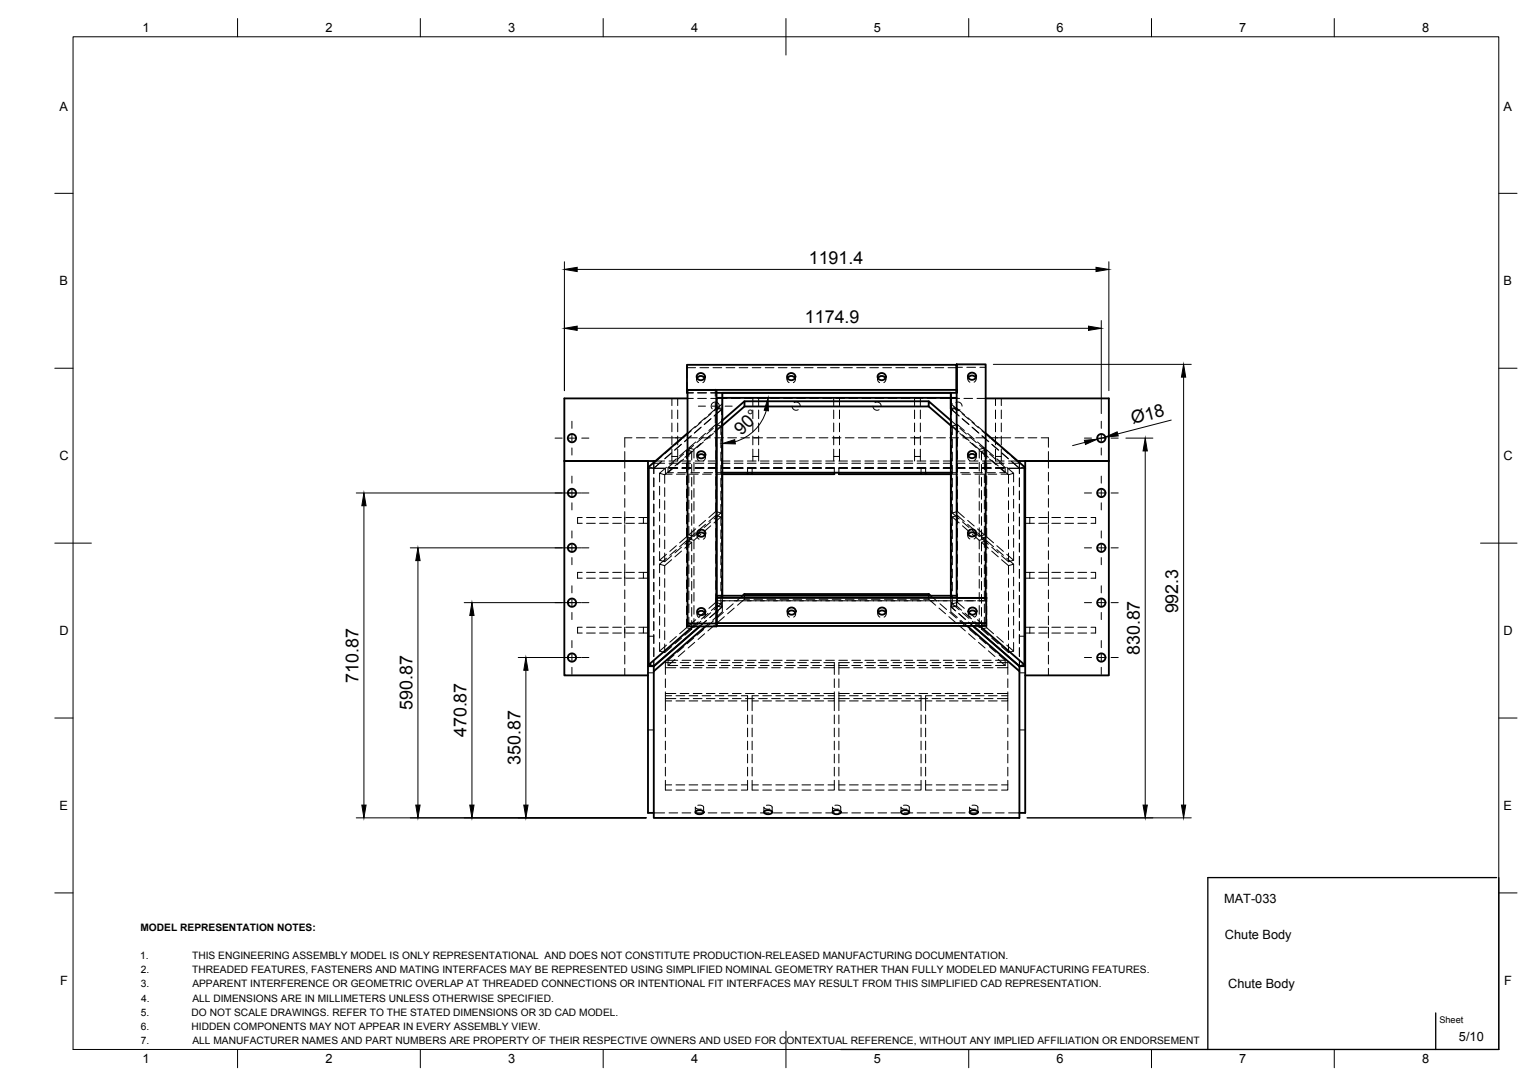
ISO-10303-21;
HEADER;
/* Generated by software containing ST-Developer
 * from STEP Tools, Inc. (www.steptools.com) 
 */

FILE_DESCRIPTION(
/* description */ ('STEP AP214'),
/* implementation_level */ '2;1');

FILE_NAME(
/* name */ 'Chute Body.step',
/* time_stamp */ '2026-11-14T07:13:32-08:00',
/* author */ (''),
/* organization */ (''),
/* preprocessor_version */ 'ST-DEVELOPER v20.2',
/* originating_system */ 'Autodesk Translation Framework v15.17.0.0',
/* authorisation */ '');

FILE_SCHEMA (('AUTOMOTIVE_DESIGN { 1 0 10303 214 3 1 1 }'));
ENDSEC;

DATA;
#10=MECHANICAL_DESIGN_GEOMETRIC_PRESENTATION_REPRESENTATION('',(#1325,#1326,#1327,#1328,#1329,#1330,#1331,#1332,#1333,#1334,#1335,#1336,#1337,#1338,#1339,#1340,#1341,#1342,#1343,#1344,#1345,#1346,#1347,#1348,#1349,#1350,#1351,#1352,#1353,#1354,#1355,#1356,#1357,#1358,#1359,#1360,#1361,#1362,#1363,#1364,#1365,#1366,#1367,#1368,#1369,#1370,#1371,#1372,#1373,#1374,#1375,#1376),#32903);
#682=SHAPE_REPRESENTATION_RELATIONSHIP('SRR','None',#33024,#696);
#696=ADVANCED_BREP_SHAPE_REPRESENTATION('',(#1414,#1415,#1416,#1417,#1418,
#1419,#1420,#1421,#1422,#1423,#1424,#1425,#1426,#1427,#1428,#1429,#1430,
#1431,#1432,#1433,#1434,#1435,#1436,#1437,#1438,#1439,#1440,#1441,#1442,
#1443,#1444,#1445,#1446,#1447,#1448,#1449,#1450,#1451,#1452,#1453,#1454,
#1455,#1456,#1457,#1458,#1459,#1460,#1461,#1462,#1463,#1464,#1465),#32899);
#969=CIRCLE('',#16556,40.);
#970=CIRCLE('',#16557,40.);
#971=CIRCLE('',#16559,75.);
#972=CIRCLE('',#16561,75.);
#973=CIRCLE('',#16569,40.);
#974=CIRCLE('',#16570,40.);
#975=CIRCLE('',#16572,75.);
#976=CIRCLE('',#16574,75.);
#977=CIRCLE('',#16582,8.99999999999999);
#978=CIRCLE('',#16583,8.99999999999999);
#979=CIRCLE('',#16585,8.99999999999999);
#980=CIRCLE('',#16586,8.99999999999999);
#981=CIRCLE('',#16588,8.99999999999998);
#982=CIRCLE('',#16589,8.99999999999998);
#983=CIRCLE('',#16591,9.);
#984=CIRCLE('',#16592,8.99999999999999);
#985=CIRCLE('',#16594,8.99999999999999);
#986=CIRCLE('',#16595,8.99999999999999);
#987=CIRCLE('',#16627,8.99999999999997);
#988=CIRCLE('',#16628,8.99999999999997);
#989=CIRCLE('',#16630,8.99999999999999);
#990=CIRCLE('',#16631,8.99999999999999);
#991=CIRCLE('',#16633,8.99999999999997);
#992=CIRCLE('',#16634,8.99999999999997);
#993=CIRCLE('',#16642,8.99999999999998);
#994=CIRCLE('',#16643,8.99999999999998);
#995=CIRCLE('',#16645,9.);
#996=CIRCLE('',#16646,9.);
#997=CIRCLE('',#16648,8.99999999999995);
#998=CIRCLE('',#16649,8.99999999999995);
#999=CIRCLE('',#16657,8.99999999999998);
#1000=CIRCLE('',#16658,8.99999999999998);
#1001=CIRCLE('',#16660,8.99999999999999);
#1002=CIRCLE('',#16661,8.99999999999999);
#1003=CIRCLE('',#16663,8.99999999999997);
#1004=CIRCLE('',#16664,8.99999999999997);
#1005=CIRCLE('',#16672,8.99999999999998);
#1006=CIRCLE('',#16673,8.99999999999998);
#1007=CIRCLE('',#16675,9.);
#1008=CIRCLE('',#16676,9.);
#1009=CIRCLE('',#16678,8.99999999999995);
#1010=CIRCLE('',#16679,8.99999999999995);
#1011=CIRCLE('',#16717,9.00000000000004);
#1012=CIRCLE('',#16718,9.00000000000004);
#1013=CIRCLE('',#16720,9.00000000000004);
#1014=CIRCLE('',#16721,9.00000000000004);
#1015=CIRCLE('',#16723,9.00000000000006);
#1016=CIRCLE('',#16724,9.00000000000006);
#1017=CIRCLE('',#16726,9.00000000000006);
#1018=CIRCLE('',#16727,9.00000000000006);
#1019=CIRCLE('',#16735,9.00000000000004);
#1020=CIRCLE('',#16736,9.00000000000004);
#1021=CIRCLE('',#16738,9.00000000000004);
#1022=CIRCLE('',#16739,9.00000000000004);
#1023=CIRCLE('',#16741,9.00000000000004);
#1024=CIRCLE('',#16742,9.00000000000004);
#1025=CIRCLE('',#16744,9.00000000000004);
#1026=CIRCLE('',#16745,9.00000000000004);
#1027=CIRCLE('',#16747,9.00000000000004);
#1028=CIRCLE('',#16748,9.00000000000004);
#1029=CIRCLE('',#16750,9.00000000000004);
#1030=CIRCLE('',#16751,9.00000000000004);
#1031=CIRCLE('',#16858,9.00000000000004);
#1032=CIRCLE('',#16859,9.00000000000004);
#1033=CIRCLE('',#16861,9.00000000000004);
#1034=CIRCLE('',#16862,9.00000000000004);
#1035=CIRCLE('',#16864,9.00000000000006);
#1036=CIRCLE('',#16865,9.00000000000006);
#1037=CIRCLE('',#16867,9.00000000000006);
#1038=CIRCLE('',#16868,9.00000000000006);
#1250=CYLINDRICAL_SURFACE('',#16555,40.);
#1251=CYLINDRICAL_SURFACE('',#16566,75.);
#1252=CYLINDRICAL_SURFACE('',#16568,40.);
#1253=CYLINDRICAL_SURFACE('',#16579,75.);
#1254=CYLINDRICAL_SURFACE('',#16581,8.99999999999999);
#1255=CYLINDRICAL_SURFACE('',#16584,8.99999999999999);
#1256=CYLINDRICAL_SURFACE('',#16587,8.99999999999998);
#1257=CYLINDRICAL_SURFACE('',#16590,9.);
#1258=CYLINDRICAL_SURFACE('',#16593,8.99999999999999);
#1259=CYLINDRICAL_SURFACE('',#16626,8.99999999999997);
#1260=CYLINDRICAL_SURFACE('',#16629,8.99999999999999);
#1261=CYLINDRICAL_SURFACE('',#16632,8.99999999999997);
#1262=CYLINDRICAL_SURFACE('',#16641,8.99999999999998);
#1263=CYLINDRICAL_SURFACE('',#16644,9.);
#1264=CYLINDRICAL_SURFACE('',#16647,8.99999999999995);
#1265=CYLINDRICAL_SURFACE('',#16656,8.99999999999998);
#1266=CYLINDRICAL_SURFACE('',#16659,8.99999999999999);
#1267=CYLINDRICAL_SURFACE('',#16662,8.99999999999997);
#1268=CYLINDRICAL_SURFACE('',#16671,8.99999999999998);
#1269=CYLINDRICAL_SURFACE('',#16674,9.);
#1270=CYLINDRICAL_SURFACE('',#16677,8.99999999999996);
#1271=CYLINDRICAL_SURFACE('',#16716,9.00000000000004);
#1272=CYLINDRICAL_SURFACE('',#16719,9.00000000000004);
#1273=CYLINDRICAL_SURFACE('',#16722,9.00000000000006);
#1274=CYLINDRICAL_SURFACE('',#16725,9.00000000000006);
#1275=CYLINDRICAL_SURFACE('',#16734,9.00000000000004);
#1276=CYLINDRICAL_SURFACE('',#16737,9.00000000000004);
#1277=CYLINDRICAL_SURFACE('',#16740,9.00000000000004);
#1278=CYLINDRICAL_SURFACE('',#16743,9.00000000000004);
#1279=CYLINDRICAL_SURFACE('',#16746,9.00000000000004);
#1280=CYLINDRICAL_SURFACE('',#16749,9.00000000000004);
#1281=CYLINDRICAL_SURFACE('',#16857,9.00000000000004);
#1282=CYLINDRICAL_SURFACE('',#16860,9.00000000000004);
#1283=CYLINDRICAL_SURFACE('',#16863,9.00000000000006);
#1284=CYLINDRICAL_SURFACE('',#16866,9.00000000000006);
#1325=STYLED_ITEM('',(#33101),#1414);
#1326=STYLED_ITEM('',(#33101),#1415);
#1327=STYLED_ITEM('',(#33101),#1416);
#1328=STYLED_ITEM('',(#33101),#1417);
#1329=STYLED_ITEM('',(#33101),#1418);
#1330=STYLED_ITEM('',(#33101),#1419);
#1331=STYLED_ITEM('',(#33101),#1420);
#1332=STYLED_ITEM('',(#33101),#1421);
#1333=STYLED_ITEM('',(#33101),#1422);
#1334=STYLED_ITEM('',(#33101),#1423);
#1335=STYLED_ITEM('',(#33101),#1424);
#1336=STYLED_ITEM('',(#33101),#1425);
#1337=STYLED_ITEM('',(#33101),#1426);
#1338=STYLED_ITEM('',(#33101),#1427);
#1339=STYLED_ITEM('',(#33101),#1428);
#1340=STYLED_ITEM('',(#33101),#1429);
#1341=STYLED_ITEM('',(#33101),#1430);
#1342=STYLED_ITEM('',(#33101),#1431);
#1343=STYLED_ITEM('',(#33101),#1432);
#1344=STYLED_ITEM('',(#33101),#1433);
#1345=STYLED_ITEM('',(#33101),#1434);
#1346=STYLED_ITEM('',(#33101),#1435);
#1347=STYLED_ITEM('',(#33101),#1436);
#1348=STYLED_ITEM('',(#33101),#1437);
#1349=STYLED_ITEM('',(#33101),#1438);
#1350=STYLED_ITEM('',(#33101),#1439);
#1351=STYLED_ITEM('',(#33101),#1440);
#1352=STYLED_ITEM('',(#33101),#1441);
#1353=STYLED_ITEM('',(#33101),#1442);
#1354=STYLED_ITEM('',(#33101),#1443);
#1355=STYLED_ITEM('',(#33101),#1444);
#1356=STYLED_ITEM('',(#33101),#1445);
#1357=STYLED_ITEM('',(#33101),#1446);
#1358=STYLED_ITEM('',(#33101),#1447);
#1359=STYLED_ITEM('',(#33101),#1448);
#1360=STYLED_ITEM('',(#33101),#1449);
#1361=STYLED_ITEM('',(#33101),#1450);
#1362=STYLED_ITEM('',(#33101),#1451);
#1363=STYLED_ITEM('',(#33101),#1452);
#1364=STYLED_ITEM('',(#33101),#1453);
#1365=STYLED_ITEM('',(#33101),#1454);
#1366=STYLED_ITEM('',(#33101),#1455);
#1367=STYLED_ITEM('',(#33101),#1456);
#1368=STYLED_ITEM('',(#33101),#1457);
#1369=STYLED_ITEM('',(#33101),#1458);
#1370=STYLED_ITEM('',(#33101),#1459);
#1371=STYLED_ITEM('',(#33101),#1460);
#1372=STYLED_ITEM('',(#33101),#1461);
#1373=STYLED_ITEM('',(#33101),#1462);
#1374=STYLED_ITEM('',(#33101),#1463);
#1375=STYLED_ITEM('',(#33101),#1464);
#1376=STYLED_ITEM('',(#33101),#1465);
#1414=MANIFOLD_SOLID_BREP('Body1',#15573);
#1415=MANIFOLD_SOLID_BREP('Body2',#15574);
#1416=MANIFOLD_SOLID_BREP('Body3',#15575);
#1417=MANIFOLD_SOLID_BREP('Body4',#15576);
#1418=MANIFOLD_SOLID_BREP('Body5',#15577);
#1419=MANIFOLD_SOLID_BREP('Body6',#15578);
#1420=MANIFOLD_SOLID_BREP('Body7',#15579);
#1421=MANIFOLD_SOLID_BREP('Body8',#15580);
#1422=MANIFOLD_SOLID_BREP('Body9',#15581);
#1423=MANIFOLD_SOLID_BREP('Body10',#15582);
#1424=MANIFOLD_SOLID_BREP('Body11',#15583);
#1425=MANIFOLD_SOLID_BREP('Body12',#15584);
#1426=MANIFOLD_SOLID_BREP('Body13',#15585);
#1427=MANIFOLD_SOLID_BREP('Body14',#15586);
#1428=MANIFOLD_SOLID_BREP('Body15',#15587);
#1429=MANIFOLD_SOLID_BREP('Body16',#15588);
#1430=MANIFOLD_SOLID_BREP('Body17',#15589);
#1431=MANIFOLD_SOLID_BREP('Body18',#15590);
#1432=MANIFOLD_SOLID_BREP('Body19',#15591);
#1433=MANIFOLD_SOLID_BREP('Body20',#15592);
#1434=MANIFOLD_SOLID_BREP('Body21',#15593);
#1435=MANIFOLD_SOLID_BREP('Body22',#15594);
#1436=MANIFOLD_SOLID_BREP('Body23',#15595);
#1437=MANIFOLD_SOLID_BREP('Body24',#15596);
#1438=MANIFOLD_SOLID_BREP('Body25',#15597);
#1439=MANIFOLD_SOLID_BREP('Body26',#15598);
#1440=MANIFOLD_SOLID_BREP('Body27',#15599);
#1441=MANIFOLD_SOLID_BREP('Body28',#15600);
#1442=MANIFOLD_SOLID_BREP('Body29',#15601);
#1443=MANIFOLD_SOLID_BREP('Body30',#15602);
#1444=MANIFOLD_SOLID_BREP('Body31',#15603);
#1445=MANIFOLD_SOLID_BREP('Body32',#15604);
#1446=MANIFOLD_SOLID_BREP('Body33',#15605);
#1447=MANIFOLD_SOLID_BREP('Body34',#15606);
#1448=MANIFOLD_SOLID_BREP('Body35',#15607);
#1449=MANIFOLD_SOLID_BREP('Body36',#15608);
#1450=MANIFOLD_SOLID_BREP('Body37',#15609);
#1451=MANIFOLD_SOLID_BREP('Body38',#15610);
#1452=MANIFOLD_SOLID_BREP('Body39',#15611);
#1453=MANIFOLD_SOLID_BREP('Body40',#15612);
#1454=MANIFOLD_SOLID_BREP('Body41',#15613);
#1455=MANIFOLD_SOLID_BREP('Body42',#15614);
#1456=MANIFOLD_SOLID_BREP('Body43',#15615);
#1457=MANIFOLD_SOLID_BREP('Body44',#15616);
#1458=MANIFOLD_SOLID_BREP('Body45',#15617);
#1459=MANIFOLD_SOLID_BREP('Body46',#15618);
#1460=MANIFOLD_SOLID_BREP('Body47',#15619);
#1461=MANIFOLD_SOLID_BREP('Body48',#15620);
#1462=MANIFOLD_SOLID_BREP('Body49',#15621);
#1463=MANIFOLD_SOLID_BREP('Body50',#15622);
#1464=MANIFOLD_SOLID_BREP('Body51',#15623);
#1465=MANIFOLD_SOLID_BREP('Body52',#15624);
#1605=FACE_BOUND('',#3169,.T.);
#1606=FACE_BOUND('',#3171,.T.);
#1607=FACE_BOUND('',#3180,.T.);
#1608=FACE_BOUND('',#3182,.T.);
#1609=FACE_BOUND('',#3195,.T.);
#1610=FACE_BOUND('',#3196,.T.);
#1611=FACE_BOUND('',#3197,.T.);
#1612=FACE_BOUND('',#3198,.T.);
#1613=FACE_BOUND('',#3199,.T.);
#1614=FACE_BOUND('',#3201,.T.);
#1615=FACE_BOUND('',#3202,.T.);
#1616=FACE_BOUND('',#3203,.T.);
#1617=FACE_BOUND('',#3204,.T.);
#1618=FACE_BOUND('',#3205,.T.);
#1619=FACE_BOUND('',#3238,.T.);
#1620=FACE_BOUND('',#3239,.T.);
#1621=FACE_BOUND('',#3240,.T.);
#1622=FACE_BOUND('',#3242,.T.);
#1623=FACE_BOUND('',#3243,.T.);
#1624=FACE_BOUND('',#3244,.T.);
#1625=FACE_BOUND('',#3253,.T.);
#1626=FACE_BOUND('',#3254,.T.);
#1627=FACE_BOUND('',#3255,.T.);
#1628=FACE_BOUND('',#3257,.T.);
#1629=FACE_BOUND('',#3258,.T.);
#1630=FACE_BOUND('',#3259,.T.);
#1631=FACE_BOUND('',#3268,.T.);
#1632=FACE_BOUND('',#3269,.T.);
#1633=FACE_BOUND('',#3270,.T.);
#1634=FACE_BOUND('',#3272,.T.);
#1635=FACE_BOUND('',#3273,.T.);
#1636=FACE_BOUND('',#3274,.T.);
#1637=FACE_BOUND('',#3283,.T.);
#1638=FACE_BOUND('',#3284,.T.);
#1639=FACE_BOUND('',#3285,.T.);
#1640=FACE_BOUND('',#3287,.T.);
#1641=FACE_BOUND('',#3288,.T.);
#1642=FACE_BOUND('',#3289,.T.);
#1643=FACE_BOUND('',#3329,.T.);
#1644=FACE_BOUND('',#3330,.T.);
#1645=FACE_BOUND('',#3331,.T.);
#1646=FACE_BOUND('',#3332,.T.);
#1647=FACE_BOUND('',#3334,.T.);
#1648=FACE_BOUND('',#3335,.T.);
#1649=FACE_BOUND('',#3336,.T.);
#1650=FACE_BOUND('',#3337,.T.);
#1651=FACE_BOUND('',#3353,.T.);
#1652=FACE_BOUND('',#3354,.T.);
#1653=FACE_BOUND('',#3355,.T.);
#1654=FACE_BOUND('',#3356,.T.);
#1655=FACE_BOUND('',#3357,.T.);
#1656=FACE_BOUND('',#3358,.T.);
#1657=FACE_BOUND('',#3360,.T.);
#1658=FACE_BOUND('',#3361,.T.);
#1659=FACE_BOUND('',#3362,.T.);
#1660=FACE_BOUND('',#3363,.T.);
#1661=FACE_BOUND('',#3364,.T.);
#1662=FACE_BOUND('',#3365,.T.);
#1663=FACE_BOUND('',#3470,.T.);
#1664=FACE_BOUND('',#3471,.T.);
#1665=FACE_BOUND('',#3472,.T.);
#1666=FACE_BOUND('',#3473,.T.);
#1667=FACE_BOUND('',#3475,.T.);
#1668=FACE_BOUND('',#3476,.T.);
#1669=FACE_BOUND('',#3477,.T.);
#1670=FACE_BOUND('',#3478,.T.);
#2130=FACE_OUTER_BOUND('',#3161,.T.);
#2131=FACE_OUTER_BOUND('',#3162,.T.);
#2132=FACE_OUTER_BOUND('',#3163,.T.);
#2133=FACE_OUTER_BOUND('',#3164,.T.);
#2134=FACE_OUTER_BOUND('',#3165,.T.);
#2135=FACE_OUTER_BOUND('',#3166,.T.);
#2136=FACE_OUTER_BOUND('',#3167,.T.);
#2137=FACE_OUTER_BOUND('',#3168,.T.);
#2138=FACE_OUTER_BOUND('',#3170,.T.);
#2139=FACE_OUTER_BOUND('',#3172,.T.);
#2140=FACE_OUTER_BOUND('',#3173,.T.);
#2141=FACE_OUTER_BOUND('',#3174,.T.);
#2142=FACE_OUTER_BOUND('',#3175,.T.);
#2143=FACE_OUTER_BOUND('',#3176,.T.);
#2144=FACE_OUTER_BOUND('',#3177,.T.);
#2145=FACE_OUTER_BOUND('',#3178,.T.);
#2146=FACE_OUTER_BOUND('',#3179,.T.);
#2147=FACE_OUTER_BOUND('',#3181,.T.);
#2148=FACE_OUTER_BOUND('',#3183,.T.);
#2149=FACE_OUTER_BOUND('',#3184,.T.);
#2150=FACE_OUTER_BOUND('',#3185,.T.);
#2151=FACE_OUTER_BOUND('',#3186,.T.);
#2152=FACE_OUTER_BOUND('',#3187,.T.);
#2153=FACE_OUTER_BOUND('',#3188,.T.);
#2154=FACE_OUTER_BOUND('',#3189,.T.);
#2155=FACE_OUTER_BOUND('',#3190,.T.);
#2156=FACE_OUTER_BOUND('',#3191,.T.);
#2157=FACE_OUTER_BOUND('',#3192,.T.);
#2158=FACE_OUTER_BOUND('',#3193,.T.);
#2159=FACE_OUTER_BOUND('',#3194,.T.);
#2160=FACE_OUTER_BOUND('',#3200,.T.);
#2161=FACE_OUTER_BOUND('',#3206,.T.);
#2162=FACE_OUTER_BOUND('',#3207,.T.);
#2163=FACE_OUTER_BOUND('',#3208,.T.);
#2164=FACE_OUTER_BOUND('',#3209,.T.);
#2165=FACE_OUTER_BOUND('',#3210,.T.);
#2166=FACE_OUTER_BOUND('',#3211,.T.);
#2167=FACE_OUTER_BOUND('',#3212,.T.);
#2168=FACE_OUTER_BOUND('',#3213,.T.);
#2169=FACE_OUTER_BOUND('',#3214,.T.);
#2170=FACE_OUTER_BOUND('',#3215,.T.);
#2171=FACE_OUTER_BOUND('',#3216,.T.);
#2172=FACE_OUTER_BOUND('',#3217,.T.);
#2173=FACE_OUTER_BOUND('',#3218,.T.);
#2174=FACE_OUTER_BOUND('',#3219,.T.);
#2175=FACE_OUTER_BOUND('',#3220,.T.);
#2176=FACE_OUTER_BOUND('',#3221,.T.);
#2177=FACE_OUTER_BOUND('',#3222,.T.);
#2178=FACE_OUTER_BOUND('',#3223,.T.);
#2179=FACE_OUTER_BOUND('',#3224,.T.);
#2180=FACE_OUTER_BOUND('',#3225,.T.);
#2181=FACE_OUTER_BOUND('',#3226,.T.);
#2182=FACE_OUTER_BOUND('',#3227,.T.);
#2183=FACE_OUTER_BOUND('',#3228,.T.);
#2184=FACE_OUTER_BOUND('',#3229,.T.);
#2185=FACE_OUTER_BOUND('',#3230,.T.);
#2186=FACE_OUTER_BOUND('',#3231,.T.);
#2187=FACE_OUTER_BOUND('',#3232,.T.);
#2188=FACE_OUTER_BOUND('',#3233,.T.);
#2189=FACE_OUTER_BOUND('',#3234,.T.);
#2190=FACE_OUTER_BOUND('',#3235,.T.);
#2191=FACE_OUTER_BOUND('',#3236,.T.);
#2192=FACE_OUTER_BOUND('',#3237,.T.);
#2193=FACE_OUTER_BOUND('',#3241,.T.);
#2194=FACE_OUTER_BOUND('',#3245,.T.);
#2195=FACE_OUTER_BOUND('',#3246,.T.);
#2196=FACE_OUTER_BOUND('',#3247,.T.);
#2197=FACE_OUTER_BOUND('',#3248,.T.);
#2198=FACE_OUTER_BOUND('',#3249,.T.);
#2199=FACE_OUTER_BOUND('',#3250,.T.);
#2200=FACE_OUTER_BOUND('',#3251,.T.);
#2201=FACE_OUTER_BOUND('',#3252,.T.);
#2202=FACE_OUTER_BOUND('',#3256,.T.);
#2203=FACE_OUTER_BOUND('',#3260,.T.);
#2204=FACE_OUTER_BOUND('',#3261,.T.);
#2205=FACE_OUTER_BOUND('',#3262,.T.);
#2206=FACE_OUTER_BOUND('',#3263,.T.);
#2207=FACE_OUTER_BOUND('',#3264,.T.);
#2208=FACE_OUTER_BOUND('',#3265,.T.);
#2209=FACE_OUTER_BOUND('',#3266,.T.);
#2210=FACE_OUTER_BOUND('',#3267,.T.);
#2211=FACE_OUTER_BOUND('',#3271,.T.);
#2212=FACE_OUTER_BOUND('',#3275,.T.);
#2213=FACE_OUTER_BOUND('',#3276,.T.);
#2214=FACE_OUTER_BOUND('',#3277,.T.);
#2215=FACE_OUTER_BOUND('',#3278,.T.);
#2216=FACE_OUTER_BOUND('',#3279,.T.);
#2217=FACE_OUTER_BOUND('',#3280,.T.);
#2218=FACE_OUTER_BOUND('',#3281,.T.);
#2219=FACE_OUTER_BOUND('',#3282,.T.);
#2220=FACE_OUTER_BOUND('',#3286,.T.);
#2221=FACE_OUTER_BOUND('',#3290,.T.);
#2222=FACE_OUTER_BOUND('',#3291,.T.);
#2223=FACE_OUTER_BOUND('',#3292,.T.);
#2224=FACE_OUTER_BOUND('',#3293,.T.);
#2225=FACE_OUTER_BOUND('',#3294,.T.);
#2226=FACE_OUTER_BOUND('',#3295,.T.);
#2227=FACE_OUTER_BOUND('',#3296,.T.);
#2228=FACE_OUTER_BOUND('',#3297,.T.);
#2229=FACE_OUTER_BOUND('',#3298,.T.);
#2230=FACE_OUTER_BOUND('',#3299,.T.);
#2231=FACE_OUTER_BOUND('',#3300,.T.);
#2232=FACE_OUTER_BOUND('',#3301,.T.);
#2233=FACE_OUTER_BOUND('',#3302,.T.);
#2234=FACE_OUTER_BOUND('',#3303,.T.);
#2235=FACE_OUTER_BOUND('',#3304,.T.);
#2236=FACE_OUTER_BOUND('',#3305,.T.);
#2237=FACE_OUTER_BOUND('',#3306,.T.);
#2238=FACE_OUTER_BOUND('',#3307,.T.);
#2239=FACE_OUTER_BOUND('',#3308,.T.);
#2240=FACE_OUTER_BOUND('',#3309,.T.);
#2241=FACE_OUTER_BOUND('',#3310,.T.);
#2242=FACE_OUTER_BOUND('',#3311,.T.);
#2243=FACE_OUTER_BOUND('',#3312,.T.);
#2244=FACE_OUTER_BOUND('',#3313,.T.);
#2245=FACE_OUTER_BOUND('',#3314,.T.);
#2246=FACE_OUTER_BOUND('',#3315,.T.);
#2247=FACE_OUTER_BOUND('',#3316,.T.);
#2248=FACE_OUTER_BOUND('',#3317,.T.);
#2249=FACE_OUTER_BOUND('',#3318,.T.);
#2250=FACE_OUTER_BOUND('',#3319,.T.);
#2251=FACE_OUTER_BOUND('',#3320,.T.);
#2252=FACE_OUTER_BOUND('',#3321,.T.);
#2253=FACE_OUTER_BOUND('',#3322,.T.);
#2254=FACE_OUTER_BOUND('',#3323,.T.);
#2255=FACE_OUTER_BOUND('',#3324,.T.);
#2256=FACE_OUTER_BOUND('',#3325,.T.);
#2257=FACE_OUTER_BOUND('',#3326,.T.);
#2258=FACE_OUTER_BOUND('',#3327,.T.);
#2259=FACE_OUTER_BOUND('',#3328,.T.);
#2260=FACE_OUTER_BOUND('',#3333,.T.);
#2261=FACE_OUTER_BOUND('',#3338,.T.);
#2262=FACE_OUTER_BOUND('',#3339,.T.);
#2263=FACE_OUTER_BOUND('',#3340,.T.);
#2264=FACE_OUTER_BOUND('',#3341,.T.);
#2265=FACE_OUTER_BOUND('',#3342,.T.);
#2266=FACE_OUTER_BOUND('',#3343,.T.);
#2267=FACE_OUTER_BOUND('',#3344,.T.);
#2268=FACE_OUTER_BOUND('',#3345,.T.);
#2269=FACE_OUTER_BOUND('',#3346,.T.);
#2270=FACE_OUTER_BOUND('',#3347,.T.);
#2271=FACE_OUTER_BOUND('',#3348,.T.);
#2272=FACE_OUTER_BOUND('',#3349,.T.);
#2273=FACE_OUTER_BOUND('',#3350,.T.);
#2274=FACE_OUTER_BOUND('',#3351,.T.);
#2275=FACE_OUTER_BOUND('',#3352,.T.);
#2276=FACE_OUTER_BOUND('',#3359,.T.);
#2277=FACE_OUTER_BOUND('',#3366,.T.);
#2278=FACE_OUTER_BOUND('',#3367,.T.);
#2279=FACE_OUTER_BOUND('',#3368,.T.);
#2280=FACE_OUTER_BOUND('',#3369,.T.);
#2281=FACE_OUTER_BOUND('',#3370,.T.);
#2282=FACE_OUTER_BOUND('',#3371,.T.);
#2283=FACE_OUTER_BOUND('',#3372,.T.);
#2284=FACE_OUTER_BOUND('',#3373,.T.);
#2285=FACE_OUTER_BOUND('',#3374,.T.);
#2286=FACE_OUTER_BOUND('',#3375,.T.);
#2287=FACE_OUTER_BOUND('',#3376,.T.);
#2288=FACE_OUTER_BOUND('',#3377,.T.);
#2289=FACE_OUTER_BOUND('',#3378,.T.);
#2290=FACE_OUTER_BOUND('',#3379,.T.);
#2291=FACE_OUTER_BOUND('',#3380,.T.);
#2292=FACE_OUTER_BOUND('',#3381,.T.);
#2293=FACE_OUTER_BOUND('',#3382,.T.);
#2294=FACE_OUTER_BOUND('',#3383,.T.);
#2295=FACE_OUTER_BOUND('',#3384,.T.);
#2296=FACE_OUTER_BOUND('',#3385,.T.);
#2297=FACE_OUTER_BOUND('',#3386,.T.);
#2298=FACE_OUTER_BOUND('',#3387,.T.);
#2299=FACE_OUTER_BOUND('',#3388,.T.);
#2300=FACE_OUTER_BOUND('',#3389,.T.);
#2301=FACE_OUTER_BOUND('',#3390,.T.);
#2302=FACE_OUTER_BOUND('',#3391,.T.);
#2303=FACE_OUTER_BOUND('',#3392,.T.);
#2304=FACE_OUTER_BOUND('',#3393,.T.);
#2305=FACE_OUTER_BOUND('',#3394,.T.);
#2306=FACE_OUTER_BOUND('',#3395,.T.);
#2307=FACE_OUTER_BOUND('',#3396,.T.);
#2308=FACE_OUTER_BOUND('',#3397,.T.);
#2309=FACE_OUTER_BOUND('',#3398,.T.);
#2310=FACE_OUTER_BOUND('',#3399,.T.);
#2311=FACE_OUTER_BOUND('',#3400,.T.);
#2312=FACE_OUTER_BOUND('',#3401,.T.);
#2313=FACE_OUTER_BOUND('',#3402,.T.);
#2314=FACE_OUTER_BOUND('',#3403,.T.);
#2315=FACE_OUTER_BOUND('',#3404,.T.);
#2316=FACE_OUTER_BOUND('',#3405,.T.);
#2317=FACE_OUTER_BOUND('',#3406,.T.);
#2318=FACE_OUTER_BOUND('',#3407,.T.);
#2319=FACE_OUTER_BOUND('',#3408,.T.);
#2320=FACE_OUTER_BOUND('',#3409,.T.);
#2321=FACE_OUTER_BOUND('',#3410,.T.);
#2322=FACE_OUTER_BOUND('',#3411,.T.);
#2323=FACE_OUTER_BOUND('',#3412,.T.);
#2324=FACE_OUTER_BOUND('',#3413,.T.);
#2325=FACE_OUTER_BOUND('',#3414,.T.);
#2326=FACE_OUTER_BOUND('',#3415,.T.);
#2327=FACE_OUTER_BOUND('',#3416,.T.);
#2328=FACE_OUTER_BOUND('',#3417,.T.);
#2329=FACE_OUTER_BOUND('',#3418,.T.);
#2330=FACE_OUTER_BOUND('',#3419,.T.);
#2331=FACE_OUTER_BOUND('',#3420,.T.);
#2332=FACE_OUTER_BOUND('',#3421,.T.);
#2333=FACE_OUTER_BOUND('',#3422,.T.);
#2334=FACE_OUTER_BOUND('',#3423,.T.);
#2335=FACE_OUTER_BOUND('',#3424,.T.);
#2336=FACE_OUTER_BOUND('',#3425,.T.);
#2337=FACE_OUTER_BOUND('',#3426,.T.);
#2338=FACE_OUTER_BOUND('',#3427,.T.);
#2339=FACE_OUTER_BOUND('',#3428,.T.);
#2340=FACE_OUTER_BOUND('',#3429,.T.);
#2341=FACE_OUTER_BOUND('',#3430,.T.);
#2342=FACE_OUTER_BOUND('',#3431,.T.);
#2343=FACE_OUTER_BOUND('',#3432,.T.);
#2344=FACE_OUTER_BOUND('',#3433,.T.);
#2345=FACE_OUTER_BOUND('',#3434,.T.);
#2346=FACE_OUTER_BOUND('',#3435,.T.);
#2347=FACE_OUTER_BOUND('',#3436,.T.);
#2348=FACE_OUTER_BOUND('',#3437,.T.);
#2349=FACE_OUTER_BOUND('',#3438,.T.);
#2350=FACE_OUTER_BOUND('',#3439,.T.);
#2351=FACE_OUTER_BOUND('',#3440,.T.);
#2352=FACE_OUTER_BOUND('',#3441,.T.);
#2353=FACE_OUTER_BOUND('',#3442,.T.);
#2354=FACE_OUTER_BOUND('',#3443,.T.);
#2355=FACE_OUTER_BOUND('',#3444,.T.);
#2356=FACE_OUTER_BOUND('',#3445,.T.);
#2357=FACE_OUTER_BOUND('',#3446,.T.);
#2358=FACE_OUTER_BOUND('',#3447,.T.);
#2359=FACE_OUTER_BOUND('',#3448,.T.);
#2360=FACE_OUTER_BOUND('',#3449,.T.);
#2361=FACE_OUTER_BOUND('',#3450,.T.);
#2362=FACE_OUTER_BOUND('',#3451,.T.);
#2363=FACE_OUTER_BOUND('',#3452,.T.);
#2364=FACE_OUTER_BOUND('',#3453,.T.);
#2365=FACE_OUTER_BOUND('',#3454,.T.);
#2366=FACE_OUTER_BOUND('',#3455,.T.);
#2367=FACE_OUTER_BOUND('',#3456,.T.);
#2368=FACE_OUTER_BOUND('',#3457,.T.);
#2369=FACE_OUTER_BOUND('',#3458,.T.);
#2370=FACE_OUTER_BOUND('',#3459,.T.);
#2371=FACE_OUTER_BOUND('',#3460,.T.);
#2372=FACE_OUTER_BOUND('',#3461,.T.);
#2373=FACE_OUTER_BOUND('',#3462,.T.);
#2374=FACE_OUTER_BOUND('',#3463,.T.);
#2375=FACE_OUTER_BOUND('',#3464,.T.);
#2376=FACE_OUTER_BOUND('',#3465,.T.);
#2377=FACE_OUTER_BOUND('',#3466,.T.);
#2378=FACE_OUTER_BOUND('',#3467,.T.);
#2379=FACE_OUTER_BOUND('',#3468,.T.);
#2380=FACE_OUTER_BOUND('',#3469,.T.);
#2381=FACE_OUTER_BOUND('',#3474,.T.);
#2382=FACE_OUTER_BOUND('',#3479,.T.);
#2383=FACE_OUTER_BOUND('',#3480,.T.);
#2384=FACE_OUTER_BOUND('',#3481,.T.);
#2385=FACE_OUTER_BOUND('',#3482,.T.);
#2386=FACE_OUTER_BOUND('',#3483,.T.);
#2387=FACE_OUTER_BOUND('',#3484,.T.);
#2388=FACE_OUTER_BOUND('',#3485,.T.);
#2389=FACE_OUTER_BOUND('',#3486,.T.);
#2390=FACE_OUTER_BOUND('',#3487,.T.);
#2391=FACE_OUTER_BOUND('',#3488,.T.);
#2392=FACE_OUTER_BOUND('',#3489,.T.);
#2393=FACE_OUTER_BOUND('',#3490,.T.);
#2394=FACE_OUTER_BOUND('',#3491,.T.);
#2395=FACE_OUTER_BOUND('',#3492,.T.);
#2396=FACE_OUTER_BOUND('',#3493,.T.);
#2397=FACE_OUTER_BOUND('',#3494,.T.);
#2398=FACE_OUTER_BOUND('',#3495,.T.);
#2399=FACE_OUTER_BOUND('',#3496,.T.);
#2400=FACE_OUTER_BOUND('',#3497,.T.);
#2401=FACE_OUTER_BOUND('',#3498,.T.);
#2402=FACE_OUTER_BOUND('',#3499,.T.);
#2403=FACE_OUTER_BOUND('',#3500,.T.);
#2404=FACE_OUTER_BOUND('',#3501,.T.);
#2405=FACE_OUTER_BOUND('',#3502,.T.);
#2406=FACE_OUTER_BOUND('',#3503,.T.);
#2407=FACE_OUTER_BOUND('',#3504,.T.);
#2408=FACE_OUTER_BOUND('',#3505,.T.);
#2409=FACE_OUTER_BOUND('',#3506,.T.);
#2410=FACE_OUTER_BOUND('',#3507,.T.);
#2411=FACE_OUTER_BOUND('',#3508,.T.);
#2412=FACE_OUTER_BOUND('',#3509,.T.);
#2413=FACE_OUTER_BOUND('',#3510,.T.);
#2414=FACE_OUTER_BOUND('',#3511,.T.);
#2415=FACE_OUTER_BOUND('',#3512,.T.);
#2416=FACE_OUTER_BOUND('',#3513,.T.);
#2417=FACE_OUTER_BOUND('',#3514,.T.);
#2418=FACE_OUTER_BOUND('',#3515,.T.);
#2419=FACE_OUTER_BOUND('',#3516,.T.);
#2420=FACE_OUTER_BOUND('',#3517,.T.);
#2421=FACE_OUTER_BOUND('',#3518,.T.);
#2422=FACE_OUTER_BOUND('',#3519,.T.);
#2423=FACE_OUTER_BOUND('',#3520,.T.);
#2424=FACE_OUTER_BOUND('',#3521,.T.);
#2425=FACE_OUTER_BOUND('',#3522,.T.);
#2426=FACE_OUTER_BOUND('',#3523,.T.);
#2427=FACE_OUTER_BOUND('',#3524,.T.);
#2428=FACE_OUTER_BOUND('',#3525,.T.);
#2429=FACE_OUTER_BOUND('',#3526,.T.);
#2430=FACE_OUTER_BOUND('',#3527,.T.);
#2431=FACE_OUTER_BOUND('',#3528,.T.);
#2432=FACE_OUTER_BOUND('',#3529,.T.);
#2433=FACE_OUTER_BOUND('',#3530,.T.);
#2434=FACE_OUTER_BOUND('',#3531,.T.);
#2435=FACE_OUTER_BOUND('',#3532,.T.);
#2436=FACE_OUTER_BOUND('',#3533,.T.);
#2437=FACE_OUTER_BOUND('',#3534,.T.);
#2438=FACE_OUTER_BOUND('',#3535,.T.);
#2439=FACE_OUTER_BOUND('',#3536,.T.);
#2440=FACE_OUTER_BOUND('',#3537,.T.);
#2441=FACE_OUTER_BOUND('',#3538,.T.);
#2442=FACE_OUTER_BOUND('',#3539,.T.);
#2443=FACE_OUTER_BOUND('',#3540,.T.);
#2444=FACE_OUTER_BOUND('',#3541,.T.);
#2445=FACE_OUTER_BOUND('',#3542,.T.);
#2446=FACE_OUTER_BOUND('',#3543,.T.);
#2447=FACE_OUTER_BOUND('',#3544,.T.);
#2448=FACE_OUTER_BOUND('',#3545,.T.);
#2449=FACE_OUTER_BOUND('',#3546,.T.);
#2450=FACE_OUTER_BOUND('',#3547,.T.);
#2451=FACE_OUTER_BOUND('',#3548,.T.);
#2452=FACE_OUTER_BOUND('',#3549,.T.);
#2453=FACE_OUTER_BOUND('',#3550,.T.);
#2454=FACE_OUTER_BOUND('',#3551,.T.);
#2455=FACE_OUTER_BOUND('',#3552,.T.);
#2456=FACE_OUTER_BOUND('',#3553,.T.);
#2457=FACE_OUTER_BOUND('',#3554,.T.);
#2458=FACE_OUTER_BOUND('',#3555,.T.);
#2459=FACE_OUTER_BOUND('',#3556,.T.);
#2460=FACE_OUTER_BOUND('',#3557,.T.);
#2461=FACE_OUTER_BOUND('',#3558,.T.);
#2462=FACE_OUTER_BOUND('',#3559,.T.);
#2463=FACE_OUTER_BOUND('',#3560,.T.);
#2464=FACE_OUTER_BOUND('',#3561,.T.);
#2465=FACE_OUTER_BOUND('',#3562,.T.);
#2466=FACE_OUTER_BOUND('',#3563,.T.);
#2467=FACE_OUTER_BOUND('',#3564,.T.);
#2468=FACE_OUTER_BOUND('',#3565,.T.);
#2469=FACE_OUTER_BOUND('',#3566,.T.);
#2470=FACE_OUTER_BOUND('',#3567,.T.);
#2471=FACE_OUTER_BOUND('',#3568,.T.);
#2472=FACE_OUTER_BOUND('',#3569,.T.);
#2473=FACE_OUTER_BOUND('',#3570,.T.);
#2474=FACE_OUTER_BOUND('',#3571,.T.);
#2475=FACE_OUTER_BOUND('',#3572,.T.);
#2476=FACE_OUTER_BOUND('',#3573,.T.);
#2477=FACE_OUTER_BOUND('',#3574,.T.);
#2478=FACE_OUTER_BOUND('',#3575,.T.);
#2479=FACE_OUTER_BOUND('',#3576,.T.);
#2480=FACE_OUTER_BOUND('',#3577,.T.);
#2481=FACE_OUTER_BOUND('',#3578,.T.);
#2482=FACE_OUTER_BOUND('',#3579,.T.);
#2483=FACE_OUTER_BOUND('',#3580,.T.);
#2484=FACE_OUTER_BOUND('',#3581,.T.);
#2485=FACE_OUTER_BOUND('',#3582,.T.);
#2486=FACE_OUTER_BOUND('',#3583,.T.);
#2487=FACE_OUTER_BOUND('',#3584,.T.);
#2488=FACE_OUTER_BOUND('',#3585,.T.);
#2489=FACE_OUTER_BOUND('',#3586,.T.);
#2490=FACE_OUTER_BOUND('',#3587,.T.);
#2491=FACE_OUTER_BOUND('',#3588,.T.);
#2492=FACE_OUTER_BOUND('',#3589,.T.);
#2493=FACE_OUTER_BOUND('',#3590,.T.);
#2494=FACE_OUTER_BOUND('',#3591,.T.);
#2495=FACE_OUTER_BOUND('',#3592,.T.);
#2496=FACE_OUTER_BOUND('',#3593,.T.);
#2497=FACE_OUTER_BOUND('',#3594,.T.);
#2498=FACE_OUTER_BOUND('',#3595,.T.);
#2499=FACE_OUTER_BOUND('',#3596,.T.);
#2500=FACE_OUTER_BOUND('',#3597,.T.);
#2501=FACE_OUTER_BOUND('',#3598,.T.);
#2502=FACE_OUTER_BOUND('',#3599,.T.);
#2503=FACE_OUTER_BOUND('',#3600,.T.);
#2504=FACE_OUTER_BOUND('',#3601,.T.);
#2505=FACE_OUTER_BOUND('',#3602,.T.);
#2506=FACE_OUTER_BOUND('',#3603,.T.);
#2507=FACE_OUTER_BOUND('',#3604,.T.);
#2508=FACE_OUTER_BOUND('',#3605,.T.);
#2509=FACE_OUTER_BOUND('',#3606,.T.);
#2510=FACE_OUTER_BOUND('',#3607,.T.);
#2511=FACE_OUTER_BOUND('',#3608,.T.);
#2512=FACE_OUTER_BOUND('',#3609,.T.);
#2513=FACE_OUTER_BOUND('',#3610,.T.);
#2514=FACE_OUTER_BOUND('',#3611,.T.);
#2515=FACE_OUTER_BOUND('',#3612,.T.);
#2516=FACE_OUTER_BOUND('',#3613,.T.);
#2517=FACE_OUTER_BOUND('',#3614,.T.);
#3161=EDGE_LOOP('',(#12121,#12122,#12123,#12124));
#3162=EDGE_LOOP('',(#12125,#12126,#12127,#12128));
#3163=EDGE_LOOP('',(#12129,#12130,#12131,#12132));
#3164=EDGE_LOOP('',(#12133,#12134,#12135,#12136));
#3165=EDGE_LOOP('',(#12137,#12138,#12139,#12140));
#3166=EDGE_LOOP('',(#12141,#12142,#12143,#12144));
#3167=EDGE_LOOP('',(#12145,#12146,#12147,#12148));
#3168=EDGE_LOOP('',(#12149,#12150,#12151,#12152,#12153,#12154));
#3169=EDGE_LOOP('',(#12155));
#3170=EDGE_LOOP('',(#12156,#12157,#12158,#12159,#12160,#12161));
#3171=EDGE_LOOP('',(#12162));
#3172=EDGE_LOOP('',(#12163,#12164,#12165,#12166));
#3173=EDGE_LOOP('',(#12167,#12168,#12169,#12170));
#3174=EDGE_LOOP('',(#12171,#12172,#12173,#12174));
#3175=EDGE_LOOP('',(#12175,#12176,#12177,#12178));
#3176=EDGE_LOOP('',(#12179,#12180,#12181,#12182));
#3177=EDGE_LOOP('',(#12183,#12184,#12185,#12186));
#3178=EDGE_LOOP('',(#12187,#12188,#12189,#12190));
#3179=EDGE_LOOP('',(#12191,#12192,#12193,#12194,#12195,#12196));
#3180=EDGE_LOOP('',(#12197));
#3181=EDGE_LOOP('',(#12198,#12199,#12200,#12201,#12202,#12203));
#3182=EDGE_LOOP('',(#12204));
#3183=EDGE_LOOP('',(#12205,#12206,#12207,#12208));
#3184=EDGE_LOOP('',(#12209,#12210,#12211,#12212));
#3185=EDGE_LOOP('',(#12213,#12214,#12215,#12216));
#3186=EDGE_LOOP('',(#12217,#12218,#12219,#12220));
#3187=EDGE_LOOP('',(#12221,#12222,#12223,#12224));
#3188=EDGE_LOOP('',(#12225,#12226,#12227,#12228));
#3189=EDGE_LOOP('',(#12229,#12230,#12231,#12232));
#3190=EDGE_LOOP('',(#12233,#12234,#12235,#12236));
#3191=EDGE_LOOP('',(#12237,#12238,#12239,#12240));
#3192=EDGE_LOOP('',(#12241,#12242,#12243,#12244));
#3193=EDGE_LOOP('',(#12245,#12246,#12247,#12248));
#3194=EDGE_LOOP('',(#12249,#12250,#12251,#12252,#12253,#12254,#12255,#12256));
#3195=EDGE_LOOP('',(#12257));
#3196=EDGE_LOOP('',(#12258));
#3197=EDGE_LOOP('',(#12259));
#3198=EDGE_LOOP('',(#12260));
#3199=EDGE_LOOP('',(#12261));
#3200=EDGE_LOOP('',(#12262,#12263,#12264,#12265,#12266,#12267,#12268,#12269));
#3201=EDGE_LOOP('',(#12270));
#3202=EDGE_LOOP('',(#12271));
#3203=EDGE_LOOP('',(#12272));
#3204=EDGE_LOOP('',(#12273));
#3205=EDGE_LOOP('',(#12274));
#3206=EDGE_LOOP('',(#12275,#12276,#12277,#12278));
#3207=EDGE_LOOP('',(#12279,#12280,#12281,#12282));
#3208=EDGE_LOOP('',(#12283,#12284,#12285,#12286));
#3209=EDGE_LOOP('',(#12287,#12288,#12289,#12290));
#3210=EDGE_LOOP('',(#12291,#12292,#12293,#12294));
#3211=EDGE_LOOP('',(#12295,#12296,#12297,#12298));
#3212=EDGE_LOOP('',(#12299,#12300,#12301,#12302));
#3213=EDGE_LOOP('',(#12303,#12304,#12305,#12306));
#3214=EDGE_LOOP('',(#12307,#12308,#12309,#12310));
#3215=EDGE_LOOP('',(#12311,#12312,#12313,#12314));
#3216=EDGE_LOOP('',(#12315,#12316,#12317,#12318));
#3217=EDGE_LOOP('',(#12319,#12320,#12321,#12322));
#3218=EDGE_LOOP('',(#12323,#12324,#12325,#12326));
#3219=EDGE_LOOP('',(#12327,#12328,#12329,#12330));
#3220=EDGE_LOOP('',(#12331,#12332,#12333,#12334));
#3221=EDGE_LOOP('',(#12335,#12336,#12337,#12338));
#3222=EDGE_LOOP('',(#12339,#12340,#12341,#12342));
#3223=EDGE_LOOP('',(#12343,#12344,#12345,#12346));
#3224=EDGE_LOOP('',(#12347,#12348,#12349,#12350));
#3225=EDGE_LOOP('',(#12351,#12352,#12353,#12354));
#3226=EDGE_LOOP('',(#12355,#12356,#12357,#12358));
#3227=EDGE_LOOP('',(#12359,#12360,#12361,#12362));
#3228=EDGE_LOOP('',(#12363,#12364,#12365,#12366));
#3229=EDGE_LOOP('',(#12367,#12368,#12369,#12370));
#3230=EDGE_LOOP('',(#12371,#12372,#12373,#12374));
#3231=EDGE_LOOP('',(#12375,#12376,#12377,#12378));
#3232=EDGE_LOOP('',(#12379,#12380,#12381,#12382,#12383,#12384));
#3233=EDGE_LOOP('',(#12385,#12386,#12387,#12388,#12389,#12390));
#3234=EDGE_LOOP('',(#12391,#12392,#12393,#12394));
#3235=EDGE_LOOP('',(#12395,#12396,#12397,#12398));
#3236=EDGE_LOOP('',(#12399,#12400,#12401,#12402));
#3237=EDGE_LOOP('',(#12403,#12404,#12405,#12406));
#3238=EDGE_LOOP('',(#12407));
#3239=EDGE_LOOP('',(#12408));
#3240=EDGE_LOOP('',(#12409));
#3241=EDGE_LOOP('',(#12410,#12411,#12412,#12413));
#3242=EDGE_LOOP('',(#12414));
#3243=EDGE_LOOP('',(#12415));
#3244=EDGE_LOOP('',(#12416));
#3245=EDGE_LOOP('',(#12417,#12418,#12419,#12420));
#3246=EDGE_LOOP('',(#12421,#12422,#12423,#12424));
#3247=EDGE_LOOP('',(#12425,#12426,#12427,#12428));
#3248=EDGE_LOOP('',(#12429,#12430,#12431,#12432));
#3249=EDGE_LOOP('',(#12433,#12434,#12435,#12436));
#3250=EDGE_LOOP('',(#12437,#12438,#12439,#12440));
#3251=EDGE_LOOP('',(#12441,#12442,#12443,#12444));
#3252=EDGE_LOOP('',(#12445,#12446,#12447,#12448));
#3253=EDGE_LOOP('',(#12449));
#3254=EDGE_LOOP('',(#12450));
#3255=EDGE_LOOP('',(#12451));
#3256=EDGE_LOOP('',(#12452,#12453,#12454,#12455));
#3257=EDGE_LOOP('',(#12456));
#3258=EDGE_LOOP('',(#12457));
#3259=EDGE_LOOP('',(#12458));
#3260=EDGE_LOOP('',(#12459,#12460,#12461,#12462));
#3261=EDGE_LOOP('',(#12463,#12464,#12465,#12466));
#3262=EDGE_LOOP('',(#12467,#12468,#12469,#12470));
#3263=EDGE_LOOP('',(#12471,#12472,#12473,#12474));
#3264=EDGE_LOOP('',(#12475,#12476,#12477,#12478));
#3265=EDGE_LOOP('',(#12479,#12480,#12481,#12482));
#3266=EDGE_LOOP('',(#12483,#12484,#12485,#12486));
#3267=EDGE_LOOP('',(#12487,#12488,#12489,#12490));
#3268=EDGE_LOOP('',(#12491));
#3269=EDGE_LOOP('',(#12492));
#3270=EDGE_LOOP('',(#12493));
#3271=EDGE_LOOP('',(#12494,#12495,#12496,#12497));
#3272=EDGE_LOOP('',(#12498));
#3273=EDGE_LOOP('',(#12499));
#3274=EDGE_LOOP('',(#12500));
#3275=EDGE_LOOP('',(#12501,#12502,#12503,#12504));
#3276=EDGE_LOOP('',(#12505,#12506,#12507,#12508));
#3277=EDGE_LOOP('',(#12509,#12510,#12511,#12512));
#3278=EDGE_LOOP('',(#12513,#12514,#12515,#12516));
#3279=EDGE_LOOP('',(#12517,#12518,#12519,#12520));
#3280=EDGE_LOOP('',(#12521,#12522,#12523,#12524));
#3281=EDGE_LOOP('',(#12525,#12526,#12527,#12528));
#3282=EDGE_LOOP('',(#12529,#12530,#12531,#12532));
#3283=EDGE_LOOP('',(#12533));
#3284=EDGE_LOOP('',(#12534));
#3285=EDGE_LOOP('',(#12535));
#3286=EDGE_LOOP('',(#12536,#12537,#12538,#12539));
#3287=EDGE_LOOP('',(#12540));
#3288=EDGE_LOOP('',(#12541));
#3289=EDGE_LOOP('',(#12542));
#3290=EDGE_LOOP('',(#12543,#12544,#12545,#12546));
#3291=EDGE_LOOP('',(#12547,#12548,#12549,#12550));
#3292=EDGE_LOOP('',(#12551,#12552,#12553,#12554));
#3293=EDGE_LOOP('',(#12555,#12556,#12557,#12558));
#3294=EDGE_LOOP('',(#12559,#12560,#12561,#12562));
#3295=EDGE_LOOP('',(#12563,#12564,#12565,#12566));
#3296=EDGE_LOOP('',(#12567,#12568,#12569,#12570));
#3297=EDGE_LOOP('',(#12571,#12572,#12573,#12574));
#3298=EDGE_LOOP('',(#12575,#12576,#12577,#12578));
#3299=EDGE_LOOP('',(#12579,#12580,#12581,#12582));
#3300=EDGE_LOOP('',(#12583,#12584,#12585,#12586));
#3301=EDGE_LOOP('',(#12587,#12588,#12589,#12590));
#3302=EDGE_LOOP('',(#12591,#12592,#12593,#12594));
#3303=EDGE_LOOP('',(#12595,#12596,#12597,#12598));
#3304=EDGE_LOOP('',(#12599,#12600,#12601,#12602));
#3305=EDGE_LOOP('',(#12603,#12604,#12605,#12606));
#3306=EDGE_LOOP('',(#12607,#12608,#12609,#12610));
#3307=EDGE_LOOP('',(#12611,#12612,#12613,#12614));
#3308=EDGE_LOOP('',(#12615,#12616,#12617,#12618));
#3309=EDGE_LOOP('',(#12619,#12620,#12621,#12622));
#3310=EDGE_LOOP('',(#12623,#12624,#12625,#12626));
#3311=EDGE_LOOP('',(#12627,#12628,#12629,#12630));
#3312=EDGE_LOOP('',(#12631,#12632,#12633,#12634));
#3313=EDGE_LOOP('',(#12635,#12636,#12637,#12638));
#3314=EDGE_LOOP('',(#12639,#12640,#12641,#12642));
#3315=EDGE_LOOP('',(#12643,#12644,#12645,#12646));
#3316=EDGE_LOOP('',(#12647,#12648,#12649,#12650));
#3317=EDGE_LOOP('',(#12651,#12652,#12653,#12654));
#3318=EDGE_LOOP('',(#12655,#12656,#12657,#12658));
#3319=EDGE_LOOP('',(#12659,#12660,#12661,#12662));
#3320=EDGE_LOOP('',(#12663,#12664,#12665,#12666));
#3321=EDGE_LOOP('',(#12667,#12668,#12669,#12670));
#3322=EDGE_LOOP('',(#12671,#12672,#12673,#12674));
#3323=EDGE_LOOP('',(#12675,#12676,#12677,#12678));
#3324=EDGE_LOOP('',(#12679,#12680,#12681,#12682));
#3325=EDGE_LOOP('',(#12683,#12684,#12685,#12686));
#3326=EDGE_LOOP('',(#12687,#12688,#12689,#12690));
#3327=EDGE_LOOP('',(#12691,#12692,#12693,#12694));
#3328=EDGE_LOOP('',(#12695,#12696,#12697,#12698));
#3329=EDGE_LOOP('',(#12699));
#3330=EDGE_LOOP('',(#12700));
#3331=EDGE_LOOP('',(#12701));
#3332=EDGE_LOOP('',(#12702));
#3333=EDGE_LOOP('',(#12703,#12704,#12705,#12706));
#3334=EDGE_LOOP('',(#12707));
#3335=EDGE_LOOP('',(#12708));
#3336=EDGE_LOOP('',(#12709));
#3337=EDGE_LOOP('',(#12710));
#3338=EDGE_LOOP('',(#12711,#12712,#12713,#12714));
#3339=EDGE_LOOP('',(#12715,#12716,#12717,#12718));
#3340=EDGE_LOOP('',(#12719,#12720,#12721,#12722));
#3341=EDGE_LOOP('',(#12723,#12724,#12725,#12726));
#3342=EDGE_LOOP('',(#12727,#12728,#12729,#12730));
#3343=EDGE_LOOP('',(#12731,#12732,#12733,#12734));
#3344=EDGE_LOOP('',(#12735,#12736,#12737,#12738));
#3345=EDGE_LOOP('',(#12739,#12740,#12741,#12742));
#3346=EDGE_LOOP('',(#12743,#12744,#12745,#12746));
#3347=EDGE_LOOP('',(#12747,#12748,#12749,#12750));
#3348=EDGE_LOOP('',(#12751,#12752,#12753,#12754));
#3349=EDGE_LOOP('',(#12755,#12756,#12757,#12758));
#3350=EDGE_LOOP('',(#12759,#12760,#12761,#12762));
#3351=EDGE_LOOP('',(#12763,#12764,#12765,#12766));
#3352=EDGE_LOOP('',(#12767,#12768,#12769,#12770));
#3353=EDGE_LOOP('',(#12771));
#3354=EDGE_LOOP('',(#12772));
#3355=EDGE_LOOP('',(#12773));
#3356=EDGE_LOOP('',(#12774));
#3357=EDGE_LOOP('',(#12775));
#3358=EDGE_LOOP('',(#12776));
#3359=EDGE_LOOP('',(#12777,#12778,#12779,#12780));
#3360=EDGE_LOOP('',(#12781));
#3361=EDGE_LOOP('',(#12782));
#3362=EDGE_LOOP('',(#12783));
#3363=EDGE_LOOP('',(#12784));
#3364=EDGE_LOOP('',(#12785));
#3365=EDGE_LOOP('',(#12786));
#3366=EDGE_LOOP('',(#12787,#12788,#12789,#12790));
#3367=EDGE_LOOP('',(#12791,#12792,#12793,#12794));
#3368=EDGE_LOOP('',(#12795,#12796,#12797,#12798));
#3369=EDGE_LOOP('',(#12799,#12800,#12801,#12802));
#3370=EDGE_LOOP('',(#12803,#12804,#12805,#12806));
#3371=EDGE_LOOP('',(#12807,#12808,#12809,#12810));
#3372=EDGE_LOOP('',(#12811,#12812,#12813,#12814));
#3373=EDGE_LOOP('',(#12815,#12816,#12817,#12818,#12819,#12820,#12821));
#3374=EDGE_LOOP('',(#12822,#12823,#12824,#12825,#12826,#12827,#12828));
#3375=EDGE_LOOP('',(#12829,#12830,#12831,#12832));
#3376=EDGE_LOOP('',(#12833,#12834,#12835,#12836));
#3377=EDGE_LOOP('',(#12837,#12838,#12839,#12840));
#3378=EDGE_LOOP('',(#12841,#12842,#12843,#12844));
#3379=EDGE_LOOP('',(#12845,#12846,#12847,#12848));
#3380=EDGE_LOOP('',(#12849,#12850,#12851,#12852));
#3381=EDGE_LOOP('',(#12853,#12854,#12855,#12856));
#3382=EDGE_LOOP('',(#12857,#12858,#12859,#12860,#12861,#12862,#12863));
#3383=EDGE_LOOP('',(#12864,#12865,#12866,#12867,#12868,#12869,#12870));
#3384=EDGE_LOOP('',(#12871,#12872,#12873,#12874));
#3385=EDGE_LOOP('',(#12875,#12876,#12877,#12878));
#3386=EDGE_LOOP('',(#12879,#12880,#12881,#12882));
#3387=EDGE_LOOP('',(#12883,#12884,#12885,#12886));
#3388=EDGE_LOOP('',(#12887,#12888,#12889,#12890));
#3389=EDGE_LOOP('',(#12891,#12892,#12893,#12894));
#3390=EDGE_LOOP('',(#12895,#12896,#12897,#12898));
#3391=EDGE_LOOP('',(#12899,#12900,#12901,#12902,#12903,#12904,#12905));
#3392=EDGE_LOOP('',(#12906,#12907,#12908,#12909,#12910,#12911,#12912));
#3393=EDGE_LOOP('',(#12913,#12914,#12915,#12916));
#3394=EDGE_LOOP('',(#12917,#12918,#12919,#12920));
#3395=EDGE_LOOP('',(#12921,#12922,#12923,#12924));
#3396=EDGE_LOOP('',(#12925,#12926,#12927,#12928));
#3397=EDGE_LOOP('',(#12929,#12930,#12931,#12932));
#3398=EDGE_LOOP('',(#12933,#12934,#12935,#12936));
#3399=EDGE_LOOP('',(#12937,#12938,#12939,#12940));
#3400=EDGE_LOOP('',(#12941,#12942,#12943,#12944,#12945,#12946,#12947));
#3401=EDGE_LOOP('',(#12948,#12949,#12950,#12951,#12952,#12953,#12954));
#3402=EDGE_LOOP('',(#12955,#12956,#12957,#12958));
#3403=EDGE_LOOP('',(#12959,#12960,#12961,#12962));
#3404=EDGE_LOOP('',(#12963,#12964,#12965,#12966));
#3405=EDGE_LOOP('',(#12967,#12968,#12969,#12970));
#3406=EDGE_LOOP('',(#12971,#12972,#12973,#12974));
#3407=EDGE_LOOP('',(#12975,#12976,#12977,#12978));
#3408=EDGE_LOOP('',(#12979,#12980,#12981,#12982));
#3409=EDGE_LOOP('',(#12983,#12984,#12985,#12986,#12987,#12988,#12989));
#3410=EDGE_LOOP('',(#12990,#12991,#12992,#12993,#12994,#12995,#12996));
#3411=EDGE_LOOP('',(#12997,#12998,#12999,#13000));
#3412=EDGE_LOOP('',(#13001,#13002,#13003,#13004));
#3413=EDGE_LOOP('',(#13005,#13006,#13007,#13008));
#3414=EDGE_LOOP('',(#13009,#13010,#13011,#13012));
#3415=EDGE_LOOP('',(#13013,#13014,#13015,#13016));
#3416=EDGE_LOOP('',(#13017,#13018,#13019,#13020));
#3417=EDGE_LOOP('',(#13021,#13022,#13023,#13024));
#3418=EDGE_LOOP('',(#13025,#13026,#13027,#13028,#13029,#13030,#13031));
#3419=EDGE_LOOP('',(#13032,#13033,#13034,#13035,#13036,#13037,#13038));
#3420=EDGE_LOOP('',(#13039,#13040,#13041,#13042));
#3421=EDGE_LOOP('',(#13043,#13044,#13045,#13046));
#3422=EDGE_LOOP('',(#13047,#13048,#13049,#13050));
#3423=EDGE_LOOP('',(#13051,#13052,#13053,#13054));
#3424=EDGE_LOOP('',(#13055,#13056,#13057,#13058));
#3425=EDGE_LOOP('',(#13059,#13060,#13061,#13062));
#3426=EDGE_LOOP('',(#13063,#13064,#13065,#13066));
#3427=EDGE_LOOP('',(#13067,#13068,#13069,#13070,#13071,#13072,#13073));
#3428=EDGE_LOOP('',(#13074,#13075,#13076,#13077,#13078,#13079,#13080));
#3429=EDGE_LOOP('',(#13081,#13082,#13083,#13084));
#3430=EDGE_LOOP('',(#13085,#13086,#13087,#13088));
#3431=EDGE_LOOP('',(#13089,#13090,#13091,#13092));
#3432=EDGE_LOOP('',(#13093,#13094,#13095,#13096));
#3433=EDGE_LOOP('',(#13097,#13098,#13099,#13100));
#3434=EDGE_LOOP('',(#13101,#13102,#13103,#13104));
#3435=EDGE_LOOP('',(#13105,#13106,#13107,#13108));
#3436=EDGE_LOOP('',(#13109,#13110,#13111,#13112,#13113,#13114,#13115));
#3437=EDGE_LOOP('',(#13116,#13117,#13118,#13119,#13120,#13121,#13122));
#3438=EDGE_LOOP('',(#13123,#13124,#13125,#13126));
#3439=EDGE_LOOP('',(#13127,#13128,#13129,#13130));
#3440=EDGE_LOOP('',(#13131,#13132,#13133,#13134));
#3441=EDGE_LOOP('',(#13135,#13136,#13137,#13138));
#3442=EDGE_LOOP('',(#13139,#13140,#13141,#13142));
#3443=EDGE_LOOP('',(#13143,#13144,#13145,#13146));
#3444=EDGE_LOOP('',(#13147,#13148,#13149,#13150));
#3445=EDGE_LOOP('',(#13151,#13152,#13153,#13154,#13155,#13156,#13157));
#3446=EDGE_LOOP('',(#13158,#13159,#13160,#13161,#13162,#13163,#13164));
#3447=EDGE_LOOP('',(#13165,#13166,#13167,#13168));
#3448=EDGE_LOOP('',(#13169,#13170,#13171,#13172));
#3449=EDGE_LOOP('',(#13173,#13174,#13175,#13176));
#3450=EDGE_LOOP('',(#13177,#13178,#13179,#13180));
#3451=EDGE_LOOP('',(#13181,#13182,#13183,#13184));
#3452=EDGE_LOOP('',(#13185,#13186,#13187,#13188));
#3453=EDGE_LOOP('',(#13189,#13190,#13191,#13192));
#3454=EDGE_LOOP('',(#13193,#13194,#13195,#13196,#13197,#13198,#13199));
#3455=EDGE_LOOP('',(#13200,#13201,#13202,#13203,#13204,#13205,#13206));
#3456=EDGE_LOOP('',(#13207,#13208,#13209,#13210));
#3457=EDGE_LOOP('',(#13211,#13212,#13213,#13214));
#3458=EDGE_LOOP('',(#13215,#13216,#13217,#13218));
#3459=EDGE_LOOP('',(#13219,#13220,#13221,#13222));
#3460=EDGE_LOOP('',(#13223,#13224,#13225,#13226));
#3461=EDGE_LOOP('',(#13227,#13228,#13229,#13230));
#3462=EDGE_LOOP('',(#13231,#13232,#13233,#13234));
#3463=EDGE_LOOP('',(#13235,#13236,#13237,#13238,#13239,#13240,#13241));
#3464=EDGE_LOOP('',(#13242,#13243,#13244,#13245,#13246,#13247,#13248));
#3465=EDGE_LOOP('',(#13249,#13250,#13251,#13252));
#3466=EDGE_LOOP('',(#13253,#13254,#13255,#13256));
#3467=EDGE_LOOP('',(#13257,#13258,#13259,#13260));
#3468=EDGE_LOOP('',(#13261,#13262,#13263,#13264));
#3469=EDGE_LOOP('',(#13265,#13266,#13267,#13268));
#3470=EDGE_LOOP('',(#13269));
#3471=EDGE_LOOP('',(#13270));
#3472=EDGE_LOOP('',(#13271));
#3473=EDGE_LOOP('',(#13272));
#3474=EDGE_LOOP('',(#13273,#13274,#13275,#13276));
#3475=EDGE_LOOP('',(#13277));
#3476=EDGE_LOOP('',(#13278));
#3477=EDGE_LOOP('',(#13279));
#3478=EDGE_LOOP('',(#13280));
#3479=EDGE_LOOP('',(#13281,#13282,#13283,#13284));
#3480=EDGE_LOOP('',(#13285,#13286,#13287,#13288));
#3481=EDGE_LOOP('',(#13289,#13290,#13291,#13292));
#3482=EDGE_LOOP('',(#13293,#13294,#13295,#13296));
#3483=EDGE_LOOP('',(#13297,#13298,#13299,#13300));
#3484=EDGE_LOOP('',(#13301,#13302,#13303,#13304));
#3485=EDGE_LOOP('',(#13305,#13306,#13307,#13308));
#3486=EDGE_LOOP('',(#13309,#13310,#13311,#13312));
#3487=EDGE_LOOP('',(#13313,#13314,#13315,#13316));
#3488=EDGE_LOOP('',(#13317,#13318,#13319,#13320));
#3489=EDGE_LOOP('',(#13321,#13322,#13323,#13324));
#3490=EDGE_LOOP('',(#13325,#13326,#13327,#13328));
#3491=EDGE_LOOP('',(#13329,#13330,#13331,#13332));
#3492=EDGE_LOOP('',(#13333,#13334,#13335,#13336));
#3493=EDGE_LOOP('',(#13337,#13338,#13339,#13340));
#3494=EDGE_LOOP('',(#13341,#13342,#13343,#13344));
#3495=EDGE_LOOP('',(#13345,#13346,#13347,#13348));
#3496=EDGE_LOOP('',(#13349,#13350,#13351,#13352));
#3497=EDGE_LOOP('',(#13353,#13354,#13355,#13356));
#3498=EDGE_LOOP('',(#13357,#13358,#13359,#13360));
#3499=EDGE_LOOP('',(#13361,#13362,#13363,#13364));
#3500=EDGE_LOOP('',(#13365,#13366,#13367,#13368));
#3501=EDGE_LOOP('',(#13369,#13370,#13371,#13372));
#3502=EDGE_LOOP('',(#13373,#13374,#13375,#13376));
#3503=EDGE_LOOP('',(#13377,#13378,#13379,#13380));
#3504=EDGE_LOOP('',(#13381,#13382,#13383,#13384));
#3505=EDGE_LOOP('',(#13385,#13386,#13387,#13388));
#3506=EDGE_LOOP('',(#13389,#13390,#13391,#13392));
#3507=EDGE_LOOP('',(#13393,#13394,#13395,#13396));
#3508=EDGE_LOOP('',(#13397,#13398,#13399,#13400));
#3509=EDGE_LOOP('',(#13401,#13402,#13403,#13404));
#3510=EDGE_LOOP('',(#13405,#13406,#13407,#13408));
#3511=EDGE_LOOP('',(#13409,#13410,#13411,#13412));
#3512=EDGE_LOOP('',(#13413,#13414,#13415,#13416));
#3513=EDGE_LOOP('',(#13417,#13418,#13419,#13420));
#3514=EDGE_LOOP('',(#13421,#13422,#13423,#13424));
#3515=EDGE_LOOP('',(#13425,#13426,#13427,#13428));
#3516=EDGE_LOOP('',(#13429,#13430,#13431,#13432));
#3517=EDGE_LOOP('',(#13433,#13434,#13435,#13436));
#3518=EDGE_LOOP('',(#13437,#13438,#13439,#13440));
#3519=EDGE_LOOP('',(#13441,#13442,#13443,#13444));
#3520=EDGE_LOOP('',(#13445,#13446,#13447,#13448));
#3521=EDGE_LOOP('',(#13449,#13450,#13451,#13452));
#3522=EDGE_LOOP('',(#13453,#13454,#13455,#13456));
#3523=EDGE_LOOP('',(#13457,#13458,#13459,#13460));
#3524=EDGE_LOOP('',(#13461,#13462,#13463,#13464));
#3525=EDGE_LOOP('',(#13465,#13466,#13467,#13468));
#3526=EDGE_LOOP('',(#13469,#13470,#13471,#13472));
#3527=EDGE_LOOP('',(#13473,#13474,#13475,#13476));
#3528=EDGE_LOOP('',(#13477,#13478,#13479,#13480));
#3529=EDGE_LOOP('',(#13481,#13482,#13483,#13484));
#3530=EDGE_LOOP('',(#13485,#13486,#13487,#13488));
#3531=EDGE_LOOP('',(#13489,#13490,#13491,#13492));
#3532=EDGE_LOOP('',(#13493,#13494,#13495,#13496));
#3533=EDGE_LOOP('',(#13497,#13498,#13499,#13500));
#3534=EDGE_LOOP('',(#13501,#13502,#13503,#13504));
#3535=EDGE_LOOP('',(#13505,#13506,#13507,#13508));
#3536=EDGE_LOOP('',(#13509,#13510,#13511,#13512));
#3537=EDGE_LOOP('',(#13513,#13514,#13515,#13516));
#3538=EDGE_LOOP('',(#13517,#13518,#13519,#13520));
#3539=EDGE_LOOP('',(#13521,#13522,#13523,#13524));
#3540=EDGE_LOOP('',(#13525,#13526,#13527,#13528));
#3541=EDGE_LOOP('',(#13529,#13530,#13531,#13532));
#3542=EDGE_LOOP('',(#13533,#13534,#13535,#13536));
#3543=EDGE_LOOP('',(#13537,#13538,#13539,#13540));
#3544=EDGE_LOOP('',(#13541,#13542,#13543,#13544));
#3545=EDGE_LOOP('',(#13545,#13546,#13547,#13548));
#3546=EDGE_LOOP('',(#13549,#13550,#13551,#13552));
#3547=EDGE_LOOP('',(#13553,#13554,#13555,#13556));
#3548=EDGE_LOOP('',(#13557,#13558,#13559,#13560));
#3549=EDGE_LOOP('',(#13561,#13562,#13563,#13564));
#3550=EDGE_LOOP('',(#13565,#13566,#13567,#13568));
#3551=EDGE_LOOP('',(#13569,#13570,#13571,#13572));
#3552=EDGE_LOOP('',(#13573,#13574,#13575,#13576));
#3553=EDGE_LOOP('',(#13577,#13578,#13579,#13580));
#3554=EDGE_LOOP('',(#13581,#13582,#13583,#13584));
#3555=EDGE_LOOP('',(#13585,#13586,#13587,#13588));
#3556=EDGE_LOOP('',(#13589,#13590,#13591,#13592));
#3557=EDGE_LOOP('',(#13593,#13594,#13595,#13596));
#3558=EDGE_LOOP('',(#13597,#13598,#13599,#13600));
#3559=EDGE_LOOP('',(#13601,#13602,#13603,#13604));
#3560=EDGE_LOOP('',(#13605,#13606,#13607,#13608));
#3561=EDGE_LOOP('',(#13609,#13610,#13611,#13612));
#3562=EDGE_LOOP('',(#13613,#13614,#13615,#13616));
#3563=EDGE_LOOP('',(#13617,#13618,#13619,#13620));
#3564=EDGE_LOOP('',(#13621,#13622,#13623,#13624));
#3565=EDGE_LOOP('',(#13625,#13626,#13627,#13628));
#3566=EDGE_LOOP('',(#13629,#13630,#13631,#13632));
#3567=EDGE_LOOP('',(#13633,#13634,#13635,#13636));
#3568=EDGE_LOOP('',(#13637,#13638,#13639,#13640));
#3569=EDGE_LOOP('',(#13641,#13642,#13643,#13644));
#3570=EDGE_LOOP('',(#13645,#13646,#13647,#13648));
#3571=EDGE_LOOP('',(#13649,#13650,#13651,#13652));
#3572=EDGE_LOOP('',(#13653,#13654,#13655,#13656));
#3573=EDGE_LOOP('',(#13657,#13658,#13659,#13660));
#3574=EDGE_LOOP('',(#13661,#13662,#13663,#13664));
#3575=EDGE_LOOP('',(#13665,#13666,#13667,#13668));
#3576=EDGE_LOOP('',(#13669,#13670,#13671,#13672));
#3577=EDGE_LOOP('',(#13673,#13674,#13675,#13676));
#3578=EDGE_LOOP('',(#13677,#13678,#13679,#13680));
#3579=EDGE_LOOP('',(#13681,#13682,#13683,#13684));
#3580=EDGE_LOOP('',(#13685,#13686,#13687,#13688));
#3581=EDGE_LOOP('',(#13689,#13690,#13691,#13692));
#3582=EDGE_LOOP('',(#13693,#13694,#13695,#13696));
#3583=EDGE_LOOP('',(#13697,#13698,#13699,#13700));
#3584=EDGE_LOOP('',(#13701,#13702,#13703,#13704));
#3585=EDGE_LOOP('',(#13705,#13706,#13707,#13708));
#3586=EDGE_LOOP('',(#13709,#13710,#13711,#13712));
#3587=EDGE_LOOP('',(#13713,#13714,#13715,#13716));
#3588=EDGE_LOOP('',(#13717,#13718,#13719,#13720));
#3589=EDGE_LOOP('',(#13721,#13722,#13723,#13724));
#3590=EDGE_LOOP('',(#13725,#13726,#13727,#13728));
#3591=EDGE_LOOP('',(#13729,#13730,#13731,#13732));
#3592=EDGE_LOOP('',(#13733,#13734,#13735,#13736));
#3593=EDGE_LOOP('',(#13737,#13738,#13739,#13740));
#3594=EDGE_LOOP('',(#13741,#13742,#13743,#13744));
#3595=EDGE_LOOP('',(#13745,#13746,#13747,#13748));
#3596=EDGE_LOOP('',(#13749,#13750,#13751,#13752));
#3597=EDGE_LOOP('',(#13753,#13754,#13755,#13756));
#3598=EDGE_LOOP('',(#13757,#13758,#13759,#13760));
#3599=EDGE_LOOP('',(#13761,#13762,#13763,#13764));
#3600=EDGE_LOOP('',(#13765,#13766,#13767,#13768));
#3601=EDGE_LOOP('',(#13769,#13770,#13771,#13772));
#3602=EDGE_LOOP('',(#13773,#13774,#13775,#13776));
#3603=EDGE_LOOP('',(#13777,#13778,#13779,#13780));
#3604=EDGE_LOOP('',(#13781,#13782,#13783,#13784));
#3605=EDGE_LOOP('',(#13785,#13786,#13787,#13788));
#3606=EDGE_LOOP('',(#13789,#13790,#13791,#13792));
#3607=EDGE_LOOP('',(#13793,#13794,#13795,#13796));
#3608=EDGE_LOOP('',(#13797,#13798,#13799,#13800));
#3609=EDGE_LOOP('',(#13801,#13802,#13803,#13804));
#3610=EDGE_LOOP('',(#13805,#13806,#13807,#13808));
#3611=EDGE_LOOP('',(#13809,#13810,#13811,#13812));
#3612=EDGE_LOOP('',(#13813,#13814,#13815,#13816));
#3613=EDGE_LOOP('',(#13817,#13818,#13819,#13820));
#3614=EDGE_LOOP('',(#13821,#13822,#13823,#13824));
#4262=LINE('',#30709,#5666);
#4263=LINE('',#30711,#5667);
#4264=LINE('',#30713,#5668);
#4265=LINE('',#30714,#5669);
#4266=LINE('',#30717,#5670);
#4267=LINE('',#30719,#5671);
#4268=LINE('',#30720,#5672);
#4269=LINE('',#30723,#5673);
#4270=LINE('',#30725,#5674);
#4271=LINE('',#30726,#5675);
#4272=LINE('',#30728,#5676);
#4273=LINE('',#30729,#5677);
#4274=LINE('',#30736,#5678);
#4275=LINE('',#30741,#5679);
#4276=LINE('',#30743,#5680);
#4277=LINE('',#30745,#5681);
#4278=LINE('',#30747,#5682);
#4279=LINE('',#30750,#5683);
#4280=LINE('',#30754,#5684);
#4281=LINE('',#30756,#5685);
#4282=LINE('',#30760,#5686);
#4283=LINE('',#30762,#5687);
#4284=LINE('',#30763,#5688);
#4285=LINE('',#30765,#5689);
#4286=LINE('',#30766,#5690);
#4287=LINE('',#30768,#5691);
#4288=LINE('',#30770,#5692);
#4289=LINE('',#30772,#5693);
#4290=LINE('',#30774,#5694);
#4291=LINE('',#30780,#5695);
#4292=LINE('',#30785,#5696);
#4293=LINE('',#30787,#5697);
#4294=LINE('',#30791,#5698);
#4295=LINE('',#30793,#5699);
#4296=LINE('',#30794,#5700);
#4297=LINE('',#30798,#5701);
#4298=LINE('',#30800,#5702);
#4299=LINE('',#30802,#5703);
#4300=LINE('',#30804,#5704);
#4301=LINE('',#30807,#5705);
#4302=LINE('',#30809,#5706);
#4303=LINE('',#30810,#5707);
#4304=LINE('',#30812,#5708);
#4305=LINE('',#30814,#5709);
#4306=LINE('',#30816,#5710);
#4307=LINE('',#30818,#5711);
#4308=LINE('',#30824,#5712);
#4309=LINE('',#30830,#5713);
#4310=LINE('',#30836,#5714);
#4311=LINE('',#30842,#5715);
#4312=LINE('',#30848,#5716);
#4313=LINE('',#30853,#5717);
#4314=LINE('',#30855,#5718);
#4315=LINE('',#30857,#5719);
#4316=LINE('',#30859,#5720);
#4317=LINE('',#30861,#5721);
#4318=LINE('',#30863,#5722);
#4319=LINE('',#30865,#5723);
#4320=LINE('',#30866,#5724);
#4321=LINE('',#30870,#5725);
#4322=LINE('',#30872,#5726);
#4323=LINE('',#30874,#5727);
#4324=LINE('',#30876,#5728);
#4325=LINE('',#30878,#5729);
#4326=LINE('',#30880,#5730);
#4327=LINE('',#30882,#5731);
#4328=LINE('',#30883,#5732);
#4329=LINE('',#30885,#5733);
#4330=LINE('',#30886,#5734);
#4331=LINE('',#30888,#5735);
#4332=LINE('',#30890,#5736);
#4333=LINE('',#30892,#5737);
#4334=LINE('',#30894,#5738);
#4335=LINE('',#30896,#5739);
#4336=LINE('',#30898,#5740);
#4337=LINE('',#30903,#5741);
#4338=LINE('',#30905,#5742);
#4339=LINE('',#30907,#5743);
#4340=LINE('',#30908,#5744);
#4341=LINE('',#30911,#5745);
#4342=LINE('',#30913,#5746);
#4343=LINE('',#30914,#5747);
#4344=LINE('',#30917,#5748);
#4345=LINE('',#30919,#5749);
#4346=LINE('',#30920,#5750);
#4347=LINE('',#30922,#5751);
#4348=LINE('',#30923,#5752);
#4349=LINE('',#30929,#5753);
#4350=LINE('',#30931,#5754);
#4351=LINE('',#30933,#5755);
#4352=LINE('',#30934,#5756);
#4353=LINE('',#30937,#5757);
#4354=LINE('',#30939,#5758);
#4355=LINE('',#30940,#5759);
#4356=LINE('',#30943,#5760);
#4357=LINE('',#30945,#5761);
#4358=LINE('',#30946,#5762);
#4359=LINE('',#30948,#5763);
#4360=LINE('',#30949,#5764);
#4361=LINE('',#30955,#5765);
#4362=LINE('',#30957,#5766);
#4363=LINE('',#30959,#5767);
#4364=LINE('',#30960,#5768);
#4365=LINE('',#30963,#5769);
#4366=LINE('',#30965,#5770);
#4367=LINE('',#30966,#5771);
#4368=LINE('',#30969,#5772);
#4369=LINE('',#30971,#5773);
#4370=LINE('',#30972,#5774);
#4371=LINE('',#30975,#5775);
#4372=LINE('',#30977,#5776);
#4373=LINE('',#30978,#5777);
#4374=LINE('',#30981,#5778);
#4375=LINE('',#30983,#5779);
#4376=LINE('',#30984,#5780);
#4377=LINE('',#30986,#5781);
#4378=LINE('',#30987,#5782);
#4379=LINE('',#30994,#5783);
#4380=LINE('',#31000,#5784);
#4381=LINE('',#31006,#5785);
#4382=LINE('',#31011,#5786);
#4383=LINE('',#31013,#5787);
#4384=LINE('',#31015,#5788);
#4385=LINE('',#31016,#5789);
#4386=LINE('',#31020,#5790);
#4387=LINE('',#31022,#5791);
#4388=LINE('',#31024,#5792);
#4389=LINE('',#31025,#5793);
#4390=LINE('',#31027,#5794);
#4391=LINE('',#31028,#5795);
#4392=LINE('',#31030,#5796);
#4393=LINE('',#31032,#5797);
#4394=LINE('',#31038,#5798);
#4395=LINE('',#31044,#5799);
#4396=LINE('',#31050,#5800);
#4397=LINE('',#31055,#5801);
#4398=LINE('',#31057,#5802);
#4399=LINE('',#31059,#5803);
#4400=LINE('',#31060,#5804);
#4401=LINE('',#31064,#5805);
#4402=LINE('',#31066,#5806);
#4403=LINE('',#31068,#5807);
#4404=LINE('',#31069,#5808);
#4405=LINE('',#31071,#5809);
#4406=LINE('',#31072,#5810);
#4407=LINE('',#31074,#5811);
#4408=LINE('',#31076,#5812);
#4409=LINE('',#31082,#5813);
#4410=LINE('',#31088,#5814);
#4411=LINE('',#31094,#5815);
#4412=LINE('',#31099,#5816);
#4413=LINE('',#31101,#5817);
#4414=LINE('',#31103,#5818);
#4415=LINE('',#31104,#5819);
#4416=LINE('',#31108,#5820);
#4417=LINE('',#31110,#5821);
#4418=LINE('',#31112,#5822);
#4419=LINE('',#31113,#5823);
#4420=LINE('',#31115,#5824);
#4421=LINE('',#31116,#5825);
#4422=LINE('',#31118,#5826);
#4423=LINE('',#31120,#5827);
#4424=LINE('',#31126,#5828);
#4425=LINE('',#31132,#5829);
#4426=LINE('',#31138,#5830);
#4427=LINE('',#31143,#5831);
#4428=LINE('',#31145,#5832);
#4429=LINE('',#31147,#5833);
#4430=LINE('',#31148,#5834);
#4431=LINE('',#31152,#5835);
#4432=LINE('',#31154,#5836);
#4433=LINE('',#31156,#5837);
#4434=LINE('',#31157,#5838);
#4435=LINE('',#31159,#5839);
#4436=LINE('',#31160,#5840);
#4437=LINE('',#31162,#5841);
#4438=LINE('',#31164,#5842);
#4439=LINE('',#31169,#5843);
#4440=LINE('',#31171,#5844);
#4441=LINE('',#31173,#5845);
#4442=LINE('',#31174,#5846);
#4443=LINE('',#31177,#5847);
#4444=LINE('',#31179,#5848);
#4445=LINE('',#31180,#5849);
#4446=LINE('',#31183,#5850);
#4447=LINE('',#31185,#5851);
#4448=LINE('',#31186,#5852);
#4449=LINE('',#31188,#5853);
#4450=LINE('',#31189,#5854);
#4451=LINE('',#31195,#5855);
#4452=LINE('',#31197,#5856);
#4453=LINE('',#31199,#5857);
#4454=LINE('',#31200,#5858);
#4455=LINE('',#31203,#5859);
#4456=LINE('',#31205,#5860);
#4457=LINE('',#31206,#5861);
#4458=LINE('',#31209,#5862);
#4459=LINE('',#31211,#5863);
#4460=LINE('',#31212,#5864);
#4461=LINE('',#31214,#5865);
#4462=LINE('',#31215,#5866);
#4463=LINE('',#31221,#5867);
#4464=LINE('',#31223,#5868);
#4465=LINE('',#31225,#5869);
#4466=LINE('',#31226,#5870);
#4467=LINE('',#31229,#5871);
#4468=LINE('',#31231,#5872);
#4469=LINE('',#31232,#5873);
#4470=LINE('',#31235,#5874);
#4471=LINE('',#31237,#5875);
#4472=LINE('',#31238,#5876);
#4473=LINE('',#31240,#5877);
#4474=LINE('',#31241,#5878);
#4475=LINE('',#31247,#5879);
#4476=LINE('',#31249,#5880);
#4477=LINE('',#31251,#5881);
#4478=LINE('',#31252,#5882);
#4479=LINE('',#31255,#5883);
#4480=LINE('',#31257,#5884);
#4481=LINE('',#31258,#5885);
#4482=LINE('',#31261,#5886);
#4483=LINE('',#31263,#5887);
#4484=LINE('',#31264,#5888);
#4485=LINE('',#31266,#5889);
#4486=LINE('',#31267,#5890);
#4487=LINE('',#31273,#5891);
#4488=LINE('',#31275,#5892);
#4489=LINE('',#31277,#5893);
#4490=LINE('',#31278,#5894);
#4491=LINE('',#31281,#5895);
#4492=LINE('',#31283,#5896);
#4493=LINE('',#31284,#5897);
#4494=LINE('',#31287,#5898);
#4495=LINE('',#31289,#5899);
#4496=LINE('',#31290,#5900);
#4497=LINE('',#31292,#5901);
#4498=LINE('',#31293,#5902);
#4499=LINE('',#31300,#5903);
#4500=LINE('',#31306,#5904);
#4501=LINE('',#31312,#5905);
#4502=LINE('',#31318,#5906);
#4503=LINE('',#31323,#5907);
#4504=LINE('',#31325,#5908);
#4505=LINE('',#31327,#5909);
#4506=LINE('',#31328,#5910);
#4507=LINE('',#31332,#5911);
#4508=LINE('',#31334,#5912);
#4509=LINE('',#31336,#5913);
#4510=LINE('',#31337,#5914);
#4511=LINE('',#31339,#5915);
#4512=LINE('',#31340,#5916);
#4513=LINE('',#31342,#5917);
#4514=LINE('',#31344,#5918);
#4515=LINE('',#31350,#5919);
#4516=LINE('',#31356,#5920);
#4517=LINE('',#31362,#5921);
#4518=LINE('',#31368,#5922);
#4519=LINE('',#31374,#5923);
#4520=LINE('',#31380,#5924);
#4521=LINE('',#31385,#5925);
#4522=LINE('',#31387,#5926);
#4523=LINE('',#31389,#5927);
#4524=LINE('',#31390,#5928);
#4525=LINE('',#31393,#5929);
#4526=LINE('',#31395,#5930);
#4527=LINE('',#31396,#5931);
#4528=LINE('',#31399,#5932);
#4529=LINE('',#31401,#5933);
#4530=LINE('',#31402,#5934);
#4531=LINE('',#31404,#5935);
#4532=LINE('',#31405,#5936);
#4533=LINE('',#31411,#5937);
#4534=LINE('',#31413,#5938);
#4535=LINE('',#31415,#5939);
#4536=LINE('',#31416,#5940);
#4537=LINE('',#31419,#5941);
#4538=LINE('',#31421,#5942);
#4539=LINE('',#31422,#5943);
#4540=LINE('',#31425,#5944);
#4541=LINE('',#31427,#5945);
#4542=LINE('',#31428,#5946);
#4543=LINE('',#31431,#5947);
#4544=LINE('',#31433,#5948);
#4545=LINE('',#31434,#5949);
#4546=LINE('',#31437,#5950);
#4547=LINE('',#31439,#5951);
#4548=LINE('',#31440,#5952);
#4549=LINE('',#31443,#5953);
#4550=LINE('',#31445,#5954);
#4551=LINE('',#31446,#5955);
#4552=LINE('',#31448,#5956);
#4553=LINE('',#31449,#5957);
#4554=LINE('',#31455,#5958);
#4555=LINE('',#31457,#5959);
#4556=LINE('',#31459,#5960);
#4557=LINE('',#31460,#5961);
#4558=LINE('',#31463,#5962);
#4559=LINE('',#31465,#5963);
#4560=LINE('',#31466,#5964);
#4561=LINE('',#31469,#5965);
#4562=LINE('',#31471,#5966);
#4563=LINE('',#31472,#5967);
#4564=LINE('',#31475,#5968);
#4565=LINE('',#31477,#5969);
#4566=LINE('',#31478,#5970);
#4567=LINE('',#31481,#5971);
#4568=LINE('',#31483,#5972);
#4569=LINE('',#31484,#5973);
#4570=LINE('',#31487,#5974);
#4571=LINE('',#31489,#5975);
#4572=LINE('',#31490,#5976);
#4573=LINE('',#31492,#5977);
#4574=LINE('',#31493,#5978);
#4575=LINE('',#31499,#5979);
#4576=LINE('',#31501,#5980);
#4577=LINE('',#31503,#5981);
#4578=LINE('',#31504,#5982);
#4579=LINE('',#31507,#5983);
#4580=LINE('',#31509,#5984);
#4581=LINE('',#31510,#5985);
#4582=LINE('',#31513,#5986);
#4583=LINE('',#31515,#5987);
#4584=LINE('',#31516,#5988);
#4585=LINE('',#31519,#5989);
#4586=LINE('',#31521,#5990);
#4587=LINE('',#31522,#5991);
#4588=LINE('',#31525,#5992);
#4589=LINE('',#31527,#5993);
#4590=LINE('',#31528,#5994);
#4591=LINE('',#31531,#5995);
#4592=LINE('',#31533,#5996);
#4593=LINE('',#31534,#5997);
#4594=LINE('',#31536,#5998);
#4595=LINE('',#31537,#5999);
#4596=LINE('',#31543,#6000);
#4597=LINE('',#31545,#6001);
#4598=LINE('',#31547,#6002);
#4599=LINE('',#31548,#6003);
#4600=LINE('',#31551,#6004);
#4601=LINE('',#31553,#6005);
#4602=LINE('',#31554,#6006);
#4603=LINE('',#31557,#6007);
#4604=LINE('',#31559,#6008);
#4605=LINE('',#31560,#6009);
#4606=LINE('',#31563,#6010);
#4607=LINE('',#31565,#6011);
#4608=LINE('',#31566,#6012);
#4609=LINE('',#31569,#6013);
#4610=LINE('',#31571,#6014);
#4611=LINE('',#31572,#6015);
#4612=LINE('',#31575,#6016);
#4613=LINE('',#31577,#6017);
#4614=LINE('',#31578,#6018);
#4615=LINE('',#31580,#6019);
#4616=LINE('',#31581,#6020);
#4617=LINE('',#31587,#6021);
#4618=LINE('',#31589,#6022);
#4619=LINE('',#31591,#6023);
#4620=LINE('',#31592,#6024);
#4621=LINE('',#31595,#6025);
#4622=LINE('',#31597,#6026);
#4623=LINE('',#31598,#6027);
#4624=LINE('',#31601,#6028);
#4625=LINE('',#31603,#6029);
#4626=LINE('',#31604,#6030);
#4627=LINE('',#31607,#6031);
#4628=LINE('',#31609,#6032);
#4629=LINE('',#31610,#6033);
#4630=LINE('',#31613,#6034);
#4631=LINE('',#31615,#6035);
#4632=LINE('',#31616,#6036);
#4633=LINE('',#31619,#6037);
#4634=LINE('',#31621,#6038);
#4635=LINE('',#31622,#6039);
#4636=LINE('',#31624,#6040);
#4637=LINE('',#31625,#6041);
#4638=LINE('',#31631,#6042);
#4639=LINE('',#31633,#6043);
#4640=LINE('',#31635,#6044);
#4641=LINE('',#31636,#6045);
#4642=LINE('',#31639,#6046);
#4643=LINE('',#31641,#6047);
#4644=LINE('',#31642,#6048);
#4645=LINE('',#31645,#6049);
#4646=LINE('',#31647,#6050);
#4647=LINE('',#31648,#6051);
#4648=LINE('',#31651,#6052);
#4649=LINE('',#31653,#6053);
#4650=LINE('',#31654,#6054);
#4651=LINE('',#31657,#6055);
#4652=LINE('',#31659,#6056);
#4653=LINE('',#31660,#6057);
#4654=LINE('',#31663,#6058);
#4655=LINE('',#31665,#6059);
#4656=LINE('',#31666,#6060);
#4657=LINE('',#31668,#6061);
#4658=LINE('',#31669,#6062);
#4659=LINE('',#31675,#6063);
#4660=LINE('',#31677,#6064);
#4661=LINE('',#31679,#6065);
#4662=LINE('',#31680,#6066);
#4663=LINE('',#31683,#6067);
#4664=LINE('',#31685,#6068);
#4665=LINE('',#31686,#6069);
#4666=LINE('',#31689,#6070);
#4667=LINE('',#31691,#6071);
#4668=LINE('',#31692,#6072);
#4669=LINE('',#31695,#6073);
#4670=LINE('',#31697,#6074);
#4671=LINE('',#31698,#6075);
#4672=LINE('',#31701,#6076);
#4673=LINE('',#31703,#6077);
#4674=LINE('',#31704,#6078);
#4675=LINE('',#31707,#6079);
#4676=LINE('',#31709,#6080);
#4677=LINE('',#31710,#6081);
#4678=LINE('',#31712,#6082);
#4679=LINE('',#31713,#6083);
#4680=LINE('',#31719,#6084);
#4681=LINE('',#31721,#6085);
#4682=LINE('',#31723,#6086);
#4683=LINE('',#31724,#6087);
#4684=LINE('',#31727,#6088);
#4685=LINE('',#31729,#6089);
#4686=LINE('',#31730,#6090);
#4687=LINE('',#31733,#6091);
#4688=LINE('',#31735,#6092);
#4689=LINE('',#31736,#6093);
#4690=LINE('',#31739,#6094);
#4691=LINE('',#31741,#6095);
#4692=LINE('',#31742,#6096);
#4693=LINE('',#31745,#6097);
#4694=LINE('',#31747,#6098);
#4695=LINE('',#31748,#6099);
#4696=LINE('',#31751,#6100);
#4697=LINE('',#31753,#6101);
#4698=LINE('',#31754,#6102);
#4699=LINE('',#31756,#6103);
#4700=LINE('',#31757,#6104);
#4701=LINE('',#31763,#6105);
#4702=LINE('',#31765,#6106);
#4703=LINE('',#31767,#6107);
#4704=LINE('',#31768,#6108);
#4705=LINE('',#31771,#6109);
#4706=LINE('',#31773,#6110);
#4707=LINE('',#31774,#6111);
#4708=LINE('',#31777,#6112);
#4709=LINE('',#31779,#6113);
#4710=LINE('',#31780,#6114);
#4711=LINE('',#31783,#6115);
#4712=LINE('',#31785,#6116);
#4713=LINE('',#31786,#6117);
#4714=LINE('',#31789,#6118);
#4715=LINE('',#31791,#6119);
#4716=LINE('',#31792,#6120);
#4717=LINE('',#31795,#6121);
#4718=LINE('',#31797,#6122);
#4719=LINE('',#31798,#6123);
#4720=LINE('',#31800,#6124);
#4721=LINE('',#31801,#6125);
#4722=LINE('',#31807,#6126);
#4723=LINE('',#31809,#6127);
#4724=LINE('',#31811,#6128);
#4725=LINE('',#31812,#6129);
#4726=LINE('',#31815,#6130);
#4727=LINE('',#31817,#6131);
#4728=LINE('',#31818,#6132);
#4729=LINE('',#31821,#6133);
#4730=LINE('',#31823,#6134);
#4731=LINE('',#31824,#6135);
#4732=LINE('',#31827,#6136);
#4733=LINE('',#31829,#6137);
#4734=LINE('',#31830,#6138);
#4735=LINE('',#31833,#6139);
#4736=LINE('',#31835,#6140);
#4737=LINE('',#31836,#6141);
#4738=LINE('',#31839,#6142);
#4739=LINE('',#31841,#6143);
#4740=LINE('',#31842,#6144);
#4741=LINE('',#31844,#6145);
#4742=LINE('',#31845,#6146);
#4743=LINE('',#31851,#6147);
#4744=LINE('',#31853,#6148);
#4745=LINE('',#31855,#6149);
#4746=LINE('',#31856,#6150);
#4747=LINE('',#31859,#6151);
#4748=LINE('',#31861,#6152);
#4749=LINE('',#31862,#6153);
#4750=LINE('',#31865,#6154);
#4751=LINE('',#31867,#6155);
#4752=LINE('',#31868,#6156);
#4753=LINE('',#31871,#6157);
#4754=LINE('',#31873,#6158);
#4755=LINE('',#31874,#6159);
#4756=LINE('',#31877,#6160);
#4757=LINE('',#31879,#6161);
#4758=LINE('',#31880,#6162);
#4759=LINE('',#31883,#6163);
#4760=LINE('',#31885,#6164);
#4761=LINE('',#31886,#6165);
#4762=LINE('',#31888,#6166);
#4763=LINE('',#31889,#6167);
#4764=LINE('',#31896,#6168);
#4765=LINE('',#31902,#6169);
#4766=LINE('',#31908,#6170);
#4767=LINE('',#31914,#6171);
#4768=LINE('',#31919,#6172);
#4769=LINE('',#31921,#6173);
#4770=LINE('',#31923,#6174);
#4771=LINE('',#31924,#6175);
#4772=LINE('',#31928,#6176);
#4773=LINE('',#31930,#6177);
#4774=LINE('',#31932,#6178);
#4775=LINE('',#31933,#6179);
#4776=LINE('',#31935,#6180);
#4777=LINE('',#31936,#6181);
#4778=LINE('',#31938,#6182);
#4779=LINE('',#31940,#6183);
#4780=LINE('',#31945,#6184);
#4781=LINE('',#31947,#6185);
#4782=LINE('',#31949,#6186);
#4783=LINE('',#31950,#6187);
#4784=LINE('',#31953,#6188);
#4785=LINE('',#31955,#6189);
#4786=LINE('',#31956,#6190);
#4787=LINE('',#31959,#6191);
#4788=LINE('',#31961,#6192);
#4789=LINE('',#31962,#6193);
#4790=LINE('',#31964,#6194);
#4791=LINE('',#31965,#6195);
#4792=LINE('',#31971,#6196);
#4793=LINE('',#31973,#6197);
#4794=LINE('',#31975,#6198);
#4795=LINE('',#31976,#6199);
#4796=LINE('',#31979,#6200);
#4797=LINE('',#31981,#6201);
#4798=LINE('',#31982,#6202);
#4799=LINE('',#31985,#6203);
#4800=LINE('',#31987,#6204);
#4801=LINE('',#31988,#6205);
#4802=LINE('',#31990,#6206);
#4803=LINE('',#31991,#6207);
#4804=LINE('',#31997,#6208);
#4805=LINE('',#31999,#6209);
#4806=LINE('',#32001,#6210);
#4807=LINE('',#32002,#6211);
#4808=LINE('',#32005,#6212);
#4809=LINE('',#32007,#6213);
#4810=LINE('',#32008,#6214);
#4811=LINE('',#32011,#6215);
#4812=LINE('',#32013,#6216);
#4813=LINE('',#32014,#6217);
#4814=LINE('',#32016,#6218);
#4815=LINE('',#32017,#6219);
#4816=LINE('',#32023,#6220);
#4817=LINE('',#32025,#6221);
#4818=LINE('',#32027,#6222);
#4819=LINE('',#32028,#6223);
#4820=LINE('',#32031,#6224);
#4821=LINE('',#32033,#6225);
#4822=LINE('',#32034,#6226);
#4823=LINE('',#32037,#6227);
#4824=LINE('',#32039,#6228);
#4825=LINE('',#32040,#6229);
#4826=LINE('',#32042,#6230);
#4827=LINE('',#32043,#6231);
#4828=LINE('',#32049,#6232);
#4829=LINE('',#32051,#6233);
#4830=LINE('',#32053,#6234);
#4831=LINE('',#32054,#6235);
#4832=LINE('',#32057,#6236);
#4833=LINE('',#32059,#6237);
#4834=LINE('',#32060,#6238);
#4835=LINE('',#32063,#6239);
#4836=LINE('',#32065,#6240);
#4837=LINE('',#32066,#6241);
#4838=LINE('',#32068,#6242);
#4839=LINE('',#32069,#6243);
#4840=LINE('',#32075,#6244);
#4841=LINE('',#32077,#6245);
#4842=LINE('',#32079,#6246);
#4843=LINE('',#32080,#6247);
#4844=LINE('',#32083,#6248);
#4845=LINE('',#32085,#6249);
#4846=LINE('',#32086,#6250);
#4847=LINE('',#32089,#6251);
#4848=LINE('',#32091,#6252);
#4849=LINE('',#32092,#6253);
#4850=LINE('',#32094,#6254);
#4851=LINE('',#32095,#6255);
#4852=LINE('',#32101,#6256);
#4853=LINE('',#32103,#6257);
#4854=LINE('',#32105,#6258);
#4855=LINE('',#32106,#6259);
#4856=LINE('',#32109,#6260);
#4857=LINE('',#32111,#6261);
#4858=LINE('',#32112,#6262);
#4859=LINE('',#32115,#6263);
#4860=LINE('',#32117,#6264);
#4861=LINE('',#32118,#6265);
#4862=LINE('',#32120,#6266);
#4863=LINE('',#32121,#6267);
#4864=LINE('',#32127,#6268);
#4865=LINE('',#32129,#6269);
#4866=LINE('',#32131,#6270);
#4867=LINE('',#32132,#6271);
#4868=LINE('',#32135,#6272);
#4869=LINE('',#32137,#6273);
#4870=LINE('',#32138,#6274);
#4871=LINE('',#32141,#6275);
#4872=LINE('',#32143,#6276);
#4873=LINE('',#32144,#6277);
#4874=LINE('',#32146,#6278);
#4875=LINE('',#32147,#6279);
#4876=LINE('',#32153,#6280);
#4877=LINE('',#32155,#6281);
#4878=LINE('',#32157,#6282);
#4879=LINE('',#32158,#6283);
#4880=LINE('',#32161,#6284);
#4881=LINE('',#32163,#6285);
#4882=LINE('',#32164,#6286);
#4883=LINE('',#32167,#6287);
#4884=LINE('',#32169,#6288);
#4885=LINE('',#32170,#6289);
#4886=LINE('',#32172,#6290);
#4887=LINE('',#32173,#6291);
#4888=LINE('',#32179,#6292);
#4889=LINE('',#32181,#6293);
#4890=LINE('',#32183,#6294);
#4891=LINE('',#32184,#6295);
#4892=LINE('',#32187,#6296);
#4893=LINE('',#32189,#6297);
#4894=LINE('',#32190,#6298);
#4895=LINE('',#32193,#6299);
#4896=LINE('',#32195,#6300);
#4897=LINE('',#32196,#6301);
#4898=LINE('',#32198,#6302);
#4899=LINE('',#32199,#6303);
#4900=LINE('',#32205,#6304);
#4901=LINE('',#32207,#6305);
#4902=LINE('',#32209,#6306);
#4903=LINE('',#32210,#6307);
#4904=LINE('',#32213,#6308);
#4905=LINE('',#32215,#6309);
#4906=LINE('',#32216,#6310);
#4907=LINE('',#32219,#6311);
#4908=LINE('',#32221,#6312);
#4909=LINE('',#32222,#6313);
#4910=LINE('',#32224,#6314);
#4911=LINE('',#32225,#6315);
#4912=LINE('',#32231,#6316);
#4913=LINE('',#32233,#6317);
#4914=LINE('',#32235,#6318);
#4915=LINE('',#32236,#6319);
#4916=LINE('',#32239,#6320);
#4917=LINE('',#32241,#6321);
#4918=LINE('',#32242,#6322);
#4919=LINE('',#32245,#6323);
#4920=LINE('',#32247,#6324);
#4921=LINE('',#32248,#6325);
#4922=LINE('',#32250,#6326);
#4923=LINE('',#32251,#6327);
#4924=LINE('',#32257,#6328);
#4925=LINE('',#32259,#6329);
#4926=LINE('',#32261,#6330);
#4927=LINE('',#32262,#6331);
#4928=LINE('',#32265,#6332);
#4929=LINE('',#32267,#6333);
#4930=LINE('',#32268,#6334);
#4931=LINE('',#32271,#6335);
#4932=LINE('',#32273,#6336);
#4933=LINE('',#32274,#6337);
#4934=LINE('',#32276,#6338);
#4935=LINE('',#32277,#6339);
#4936=LINE('',#32283,#6340);
#4937=LINE('',#32285,#6341);
#4938=LINE('',#32287,#6342);
#4939=LINE('',#32288,#6343);
#4940=LINE('',#32291,#6344);
#4941=LINE('',#32293,#6345);
#4942=LINE('',#32294,#6346);
#4943=LINE('',#32297,#6347);
#4944=LINE('',#32299,#6348);
#4945=LINE('',#32300,#6349);
#4946=LINE('',#32302,#6350);
#4947=LINE('',#32303,#6351);
#4948=LINE('',#32309,#6352);
#4949=LINE('',#32311,#6353);
#4950=LINE('',#32313,#6354);
#4951=LINE('',#32314,#6355);
#4952=LINE('',#32317,#6356);
#4953=LINE('',#32319,#6357);
#4954=LINE('',#32320,#6358);
#4955=LINE('',#32323,#6359);
#4956=LINE('',#32325,#6360);
#4957=LINE('',#32326,#6361);
#4958=LINE('',#32328,#6362);
#4959=LINE('',#32329,#6363);
#4960=LINE('',#32335,#6364);
#4961=LINE('',#32337,#6365);
#4962=LINE('',#32339,#6366);
#4963=LINE('',#32340,#6367);
#4964=LINE('',#32343,#6368);
#4965=LINE('',#32345,#6369);
#4966=LINE('',#32346,#6370);
#4967=LINE('',#32349,#6371);
#4968=LINE('',#32351,#6372);
#4969=LINE('',#32352,#6373);
#4970=LINE('',#32354,#6374);
#4971=LINE('',#32355,#6375);
#4972=LINE('',#32361,#6376);
#4973=LINE('',#32363,#6377);
#4974=LINE('',#32365,#6378);
#4975=LINE('',#32366,#6379);
#4976=LINE('',#32369,#6380);
#4977=LINE('',#32371,#6381);
#4978=LINE('',#32372,#6382);
#4979=LINE('',#32375,#6383);
#4980=LINE('',#32377,#6384);
#4981=LINE('',#32378,#6385);
#4982=LINE('',#32380,#6386);
#4983=LINE('',#32381,#6387);
#4984=LINE('',#32387,#6388);
#4985=LINE('',#32389,#6389);
#4986=LINE('',#32391,#6390);
#4987=LINE('',#32392,#6391);
#4988=LINE('',#32395,#6392);
#4989=LINE('',#32397,#6393);
#4990=LINE('',#32398,#6394);
#4991=LINE('',#32401,#6395);
#4992=LINE('',#32403,#6396);
#4993=LINE('',#32404,#6397);
#4994=LINE('',#32406,#6398);
#4995=LINE('',#32407,#6399);
#4996=LINE('',#32413,#6400);
#4997=LINE('',#32415,#6401);
#4998=LINE('',#32417,#6402);
#4999=LINE('',#32418,#6403);
#5000=LINE('',#32421,#6404);
#5001=LINE('',#32423,#6405);
#5002=LINE('',#32424,#6406);
#5003=LINE('',#32427,#6407);
#5004=LINE('',#32429,#6408);
#5005=LINE('',#32430,#6409);
#5006=LINE('',#32432,#6410);
#5007=LINE('',#32433,#6411);
#5008=LINE('',#32439,#6412);
#5009=LINE('',#32441,#6413);
#5010=LINE('',#32443,#6414);
#5011=LINE('',#32444,#6415);
#5012=LINE('',#32447,#6416);
#5013=LINE('',#32449,#6417);
#5014=LINE('',#32450,#6418);
#5015=LINE('',#32453,#6419);
#5016=LINE('',#32455,#6420);
#5017=LINE('',#32456,#6421);
#5018=LINE('',#32458,#6422);
#5019=LINE('',#32459,#6423);
#5020=LINE('',#32465,#6424);
#5021=LINE('',#32467,#6425);
#5022=LINE('',#32469,#6426);
#5023=LINE('',#32470,#6427);
#5024=LINE('',#32473,#6428);
#5025=LINE('',#32475,#6429);
#5026=LINE('',#32476,#6430);
#5027=LINE('',#32479,#6431);
#5028=LINE('',#32481,#6432);
#5029=LINE('',#32482,#6433);
#5030=LINE('',#32484,#6434);
#5031=LINE('',#32485,#6435);
#5032=LINE('',#32491,#6436);
#5033=LINE('',#32493,#6437);
#5034=LINE('',#32495,#6438);
#5035=LINE('',#32496,#6439);
#5036=LINE('',#32499,#6440);
#5037=LINE('',#32501,#6441);
#5038=LINE('',#32502,#6442);
#5039=LINE('',#32505,#6443);
#5040=LINE('',#32507,#6444);
#5041=LINE('',#32508,#6445);
#5042=LINE('',#32510,#6446);
#5043=LINE('',#32511,#6447);
#5666=VECTOR('',#19280,1000.);
#5667=VECTOR('',#19281,1000.);
#5668=VECTOR('',#19282,1000.);
#5669=VECTOR('',#19283,1000.);
#5670=VECTOR('',#19286,1000.);
#5671=VECTOR('',#19287,1000.);
#5672=VECTOR('',#19288,1000.);
#5673=VECTOR('',#19291,1000.);
#5674=VECTOR('',#19292,1000.);
#5675=VECTOR('',#19293,1000.);
#5676=VECTOR('',#19296,1000.);
#5677=VECTOR('',#19297,1000.);
#5678=VECTOR('',#19306,40.);
#5679=VECTOR('',#19311,1000.);
#5680=VECTOR('',#19312,1000.);
#5681=VECTOR('',#19313,1000.);
#5682=VECTOR('',#19314,1000.);
#5683=VECTOR('',#19317,1000.);
#5684=VECTOR('',#19320,1000.);
#5685=VECTOR('',#19321,1000.);
#5686=VECTOR('',#19324,1000.);
#5687=VECTOR('',#19325,1000.);
#5688=VECTOR('',#19326,1000.);
#5689=VECTOR('',#19329,1000.);
#5690=VECTOR('',#19330,1000.);
#5691=VECTOR('',#19333,1000.);
#5692=VECTOR('',#19336,1000.);
#5693=VECTOR('',#19339,1000.);
#5694=VECTOR('',#19342,1000.);
#5695=VECTOR('',#19349,40.);
#5696=VECTOR('',#19354,1000.);
#5697=VECTOR('',#19355,1000.);
#5698=VECTOR('',#19358,1000.);
#5699=VECTOR('',#19359,1000.);
#5700=VECTOR('',#19360,1000.);
#5701=VECTOR('',#19363,1000.);
#5702=VECTOR('',#19364,1000.);
#5703=VECTOR('',#19365,1000.);
#5704=VECTOR('',#19366,1000.);
#5705=VECTOR('',#19369,1000.);
#5706=VECTOR('',#19372,1000.);
#5707=VECTOR('',#19373,1000.);
#5708=VECTOR('',#19376,1000.);
#5709=VECTOR('',#19379,1000.);
#5710=VECTOR('',#19382,1000.);
#5711=VECTOR('',#19385,1000.);
#5712=VECTOR('',#19392,8.99999999999999);
#5713=VECTOR('',#19399,8.99999999999999);
#5714=VECTOR('',#19406,8.99999999999998);
#5715=VECTOR('',#19413,9.);
#5716=VECTOR('',#19420,8.99999999999999);
#5717=VECTOR('',#19425,1000.);
#5718=VECTOR('',#19426,1000.);
#5719=VECTOR('',#19427,1000.);
#5720=VECTOR('',#19428,1000.);
#5721=VECTOR('',#19429,1000.);
#5722=VECTOR('',#19430,1000.);
#5723=VECTOR('',#19431,1000.);
#5724=VECTOR('',#19432,1000.);
#5725=VECTOR('',#19435,1000.);
#5726=VECTOR('',#19436,1000.);
#5727=VECTOR('',#19437,1000.);
#5728=VECTOR('',#19438,1000.);
#5729=VECTOR('',#19439,1000.);
#5730=VECTOR('',#19440,1000.);
#5731=VECTOR('',#19441,1000.);
#5732=VECTOR('',#19442,1000.);
#5733=VECTOR('',#19445,1000.);
#5734=VECTOR('',#19446,1000.);
#5735=VECTOR('',#19449,1000.);
#5736=VECTOR('',#19452,1000.);
#5737=VECTOR('',#19455,1000.);
#5738=VECTOR('',#19458,1000.);
#5739=VECTOR('',#19461,1000.);
#5740=VECTOR('',#19464,1000.);
#5741=VECTOR('',#19469,1000.);
#5742=VECTOR('',#19470,1000.);
#5743=VECTOR('',#19471,1000.);
#5744=VECTOR('',#19472,1000.);
#5745=VECTOR('',#19475,1000.);
#5746=VECTOR('',#19476,1000.);
#5747=VECTOR('',#19477,1000.);
#5748=VECTOR('',#19480,1000.);
#5749=VECTOR('',#19481,1000.);
#5750=VECTOR('',#19482,1000.);
#5751=VECTOR('',#19485,1000.);
#5752=VECTOR('',#19486,1000.);
#5753=VECTOR('',#19493,1000.);
#5754=VECTOR('',#19494,1000.);
#5755=VECTOR('',#19495,1000.);
#5756=VECTOR('',#19496,1000.);
#5757=VECTOR('',#19499,1000.);
#5758=VECTOR('',#19500,1000.);
#5759=VECTOR('',#19501,1000.);
#5760=VECTOR('',#19504,1000.);
#5761=VECTOR('',#19505,1000.);
#5762=VECTOR('',#19506,1000.);
#5763=VECTOR('',#19509,1000.);
#5764=VECTOR('',#19510,1000.);
#5765=VECTOR('',#19517,1000.);
#5766=VECTOR('',#19518,1000.);
#5767=VECTOR('',#19519,1000.);
#5768=VECTOR('',#19520,1000.);
#5769=VECTOR('',#19523,1000.);
#5770=VECTOR('',#19524,1000.);
#5771=VECTOR('',#19525,1000.);
#5772=VECTOR('',#19528,1000.);
#5773=VECTOR('',#19529,1000.);
#5774=VECTOR('',#19530,1000.);
#5775=VECTOR('',#19533,1000.);
#5776=VECTOR('',#19534,1000.);
#5777=VECTOR('',#19535,1000.);
#5778=VECTOR('',#19538,1000.);
#5779=VECTOR('',#19539,1000.);
#5780=VECTOR('',#19540,1000.);
#5781=VECTOR('',#19543,1000.);
#5782=VECTOR('',#19544,1000.);
#5783=VECTOR('',#19553,8.99999999999997);
#5784=VECTOR('',#19560,8.99999999999999);
#5785=VECTOR('',#19567,8.99999999999997);
#5786=VECTOR('',#19572,1000.);
#5787=VECTOR('',#19573,1000.);
#5788=VECTOR('',#19574,1000.);
#5789=VECTOR('',#19575,1000.);
#5790=VECTOR('',#19578,1000.);
#5791=VECTOR('',#19579,1000.);
#5792=VECTOR('',#19580,1000.);
#5793=VECTOR('',#19581,1000.);
#5794=VECTOR('',#19584,1000.);
#5795=VECTOR('',#19585,1000.);
#5796=VECTOR('',#19588,1000.);
#5797=VECTOR('',#19591,1000.);
#5798=VECTOR('',#19598,8.99999999999998);
#5799=VECTOR('',#19605,9.);
#5800=VECTOR('',#19612,8.99999999999995);
#5801=VECTOR('',#19617,1000.);
#5802=VECTOR('',#19618,1000.);
#5803=VECTOR('',#19619,1000.);
#5804=VECTOR('',#19620,1000.);
#5805=VECTOR('',#19623,1000.);
#5806=VECTOR('',#19624,1000.);
#5807=VECTOR('',#19625,1000.);
#5808=VECTOR('',#19626,1000.);
#5809=VECTOR('',#19629,1000.);
#5810=VECTOR('',#19630,1000.);
#5811=VECTOR('',#19633,1000.);
#5812=VECTOR('',#19636,1000.);
#5813=VECTOR('',#19643,8.99999999999998);
#5814=VECTOR('',#19650,8.99999999999999);
#5815=VECTOR('',#19657,8.99999999999997);
#5816=VECTOR('',#19662,1000.);
#5817=VECTOR('',#19663,1000.);
#5818=VECTOR('',#19664,1000.);
#5819=VECTOR('',#19665,1000.);
#5820=VECTOR('',#19668,1000.);
#5821=VECTOR('',#19669,1000.);
#5822=VECTOR('',#19670,1000.);
#5823=VECTOR('',#19671,1000.);
#5824=VECTOR('',#19674,1000.);
#5825=VECTOR('',#19675,1000.);
#5826=VECTOR('',#19678,1000.);
#5827=VECTOR('',#19681,1000.);
#5828=VECTOR('',#19688,8.99999999999999);
#5829=VECTOR('',#19695,9.);
#5830=VECTOR('',#19702,8.99999999999996);
#5831=VECTOR('',#19707,1000.);
#5832=VECTOR('',#19708,1000.);
#5833=VECTOR('',#19709,1000.);
#5834=VECTOR('',#19710,1000.);
#5835=VECTOR('',#19713,1000.);
#5836=VECTOR('',#19714,1000.);
#5837=VECTOR('',#19715,1000.);
#5838=VECTOR('',#19716,1000.);
#5839=VECTOR('',#19719,1000.);
#5840=VECTOR('',#19720,1000.);
#5841=VECTOR('',#19723,1000.);
#5842=VECTOR('',#19726,1000.);
#5843=VECTOR('',#19731,1000.);
#5844=VECTOR('',#19732,1000.);
#5845=VECTOR('',#19733,1000.);
#5846=VECTOR('',#19734,1000.);
#5847=VECTOR('',#19737,1000.);
#5848=VECTOR('',#19738,1000.);
#5849=VECTOR('',#19739,1000.);
#5850=VECTOR('',#19742,1000.);
#5851=VECTOR('',#19743,1000.);
#5852=VECTOR('',#19744,1000.);
#5853=VECTOR('',#19747,1000.);
#5854=VECTOR('',#19748,1000.);
#5855=VECTOR('',#19755,1000.);
#5856=VECTOR('',#19756,1000.);
#5857=VECTOR('',#19757,1000.);
#5858=VECTOR('',#19758,1000.);
#5859=VECTOR('',#19761,1000.);
#5860=VECTOR('',#19762,1000.);
#5861=VECTOR('',#19763,1000.);
#5862=VECTOR('',#19766,1000.);
#5863=VECTOR('',#19767,1000.);
#5864=VECTOR('',#19768,1000.);
#5865=VECTOR('',#19771,1000.);
#5866=VECTOR('',#19772,1000.);
#5867=VECTOR('',#19779,1000.);
#5868=VECTOR('',#19780,1000.);
#5869=VECTOR('',#19781,1000.);
#5870=VECTOR('',#19782,1000.);
#5871=VECTOR('',#19785,1000.);
#5872=VECTOR('',#19786,1000.);
#5873=VECTOR('',#19787,1000.);
#5874=VECTOR('',#19790,1000.);
#5875=VECTOR('',#19791,1000.);
#5876=VECTOR('',#19792,1000.);
#5877=VECTOR('',#19795,1000.);
#5878=VECTOR('',#19796,1000.);
#5879=VECTOR('',#19803,1000.);
#5880=VECTOR('',#19804,1000.);
#5881=VECTOR('',#19805,1000.);
#5882=VECTOR('',#19806,1000.);
#5883=VECTOR('',#19809,1000.);
#5884=VECTOR('',#19810,1000.);
#5885=VECTOR('',#19811,1000.);
#5886=VECTOR('',#19814,1000.);
#5887=VECTOR('',#19815,1000.);
#5888=VECTOR('',#19816,1000.);
#5889=VECTOR('',#19819,1000.);
#5890=VECTOR('',#19820,1000.);
#5891=VECTOR('',#19827,1000.);
#5892=VECTOR('',#19828,1000.);
#5893=VECTOR('',#19829,1000.);
#5894=VECTOR('',#19830,1000.);
#5895=VECTOR('',#19833,1000.);
#5896=VECTOR('',#19834,1000.);
#5897=VECTOR('',#19835,1000.);
#5898=VECTOR('',#19838,1000.);
#5899=VECTOR('',#19839,1000.);
#5900=VECTOR('',#19840,1000.);
#5901=VECTOR('',#19843,1000.);
#5902=VECTOR('',#19844,1000.);
#5903=VECTOR('',#19853,9.00000000000004);
#5904=VECTOR('',#19860,9.00000000000004);
#5905=VECTOR('',#19867,9.00000000000006);
#5906=VECTOR('',#19874,9.00000000000006);
#5907=VECTOR('',#19879,1000.);
#5908=VECTOR('',#19880,1000.);
#5909=VECTOR('',#19881,1000.);
#5910=VECTOR('',#19882,1000.);
#5911=VECTOR('',#19885,1000.);
#5912=VECTOR('',#19886,1000.);
#5913=VECTOR('',#19887,1000.);
#5914=VECTOR('',#19888,1000.);
#5915=VECTOR('',#19891,1000.);
#5916=VECTOR('',#19892,1000.);
#5917=VECTOR('',#19895,1000.);
#5918=VECTOR('',#19898,1000.);
#5919=VECTOR('',#19905,9.00000000000004);
#5920=VECTOR('',#19912,9.00000000000004);
#5921=VECTOR('',#19919,9.00000000000004);
#5922=VECTOR('',#19926,9.00000000000004);
#5923=VECTOR('',#19933,9.00000000000004);
#5924=VECTOR('',#19940,9.00000000000004);
#5925=VECTOR('',#19945,1000.);
#5926=VECTOR('',#19946,1000.);
#5927=VECTOR('',#19947,1000.);
#5928=VECTOR('',#19948,1000.);
#5929=VECTOR('',#19951,1000.);
#5930=VECTOR('',#19952,1000.);
#5931=VECTOR('',#19953,1000.);
#5932=VECTOR('',#19956,1000.);
#5933=VECTOR('',#19957,1000.);
#5934=VECTOR('',#19958,1000.);
#5935=VECTOR('',#19961,1000.);
#5936=VECTOR('',#19962,1000.);
#5937=VECTOR('',#19969,1000.);
#5938=VECTOR('',#19970,1000.);
#5939=VECTOR('',#19971,1000.);
#5940=VECTOR('',#19972,1000.);
#5941=VECTOR('',#19975,1000.);
#5942=VECTOR('',#19976,1000.);
#5943=VECTOR('',#19977,1000.);
#5944=VECTOR('',#19980,1000.);
#5945=VECTOR('',#19981,1000.);
#5946=VECTOR('',#19982,1000.);
#5947=VECTOR('',#19985,1000.);
#5948=VECTOR('',#19986,1000.);
#5949=VECTOR('',#19987,1000.);
#5950=VECTOR('',#19990,1000.);
#5951=VECTOR('',#19991,1000.);
#5952=VECTOR('',#19992,1000.);
#5953=VECTOR('',#19995,1000.);
#5954=VECTOR('',#19996,1000.);
#5955=VECTOR('',#19997,1000.);
#5956=VECTOR('',#20000,1000.);
#5957=VECTOR('',#20001,1000.);
#5958=VECTOR('',#20008,1000.);
#5959=VECTOR('',#20009,1000.);
#5960=VECTOR('',#20010,1000.);
#5961=VECTOR('',#20011,1000.);
#5962=VECTOR('',#20014,1000.);
#5963=VECTOR('',#20015,1000.);
#5964=VECTOR('',#20016,1000.);
#5965=VECTOR('',#20019,1000.);
#5966=VECTOR('',#20020,1000.);
#5967=VECTOR('',#20021,1000.);
#5968=VECTOR('',#20024,1000.);
#5969=VECTOR('',#20025,1000.);
#5970=VECTOR('',#20026,1000.);
#5971=VECTOR('',#20029,1000.);
#5972=VECTOR('',#20030,1000.);
#5973=VECTOR('',#20031,1000.);
#5974=VECTOR('',#20034,1000.);
#5975=VECTOR('',#20035,1000.);
#5976=VECTOR('',#20036,1000.);
#5977=VECTOR('',#20039,1000.);
#5978=VECTOR('',#20040,1000.);
#5979=VECTOR('',#20047,1000.);
#5980=VECTOR('',#20048,1000.);
#5981=VECTOR('',#20049,1000.);
#5982=VECTOR('',#20050,1000.);
#5983=VECTOR('',#20053,1000.);
#5984=VECTOR('',#20054,1000.);
#5985=VECTOR('',#20055,1000.);
#5986=VECTOR('',#20058,1000.);
#5987=VECTOR('',#20059,1000.);
#5988=VECTOR('',#20060,1000.);
#5989=VECTOR('',#20063,1000.);
#5990=VECTOR('',#20064,1000.);
#5991=VECTOR('',#20065,1000.);
#5992=VECTOR('',#20068,1000.);
#5993=VECTOR('',#20069,1000.);
#5994=VECTOR('',#20070,1000.);
#5995=VECTOR('',#20073,1000.);
#5996=VECTOR('',#20074,1000.);
#5997=VECTOR('',#20075,1000.);
#5998=VECTOR('',#20078,1000.);
#5999=VECTOR('',#20079,1000.);
#6000=VECTOR('',#20086,1000.);
#6001=VECTOR('',#20087,1000.);
#6002=VECTOR('',#20088,1000.);
#6003=VECTOR('',#20089,1000.);
#6004=VECTOR('',#20092,1000.);
#6005=VECTOR('',#20093,1000.);
#6006=VECTOR('',#20094,1000.);
#6007=VECTOR('',#20097,1000.);
#6008=VECTOR('',#20098,1000.);
#6009=VECTOR('',#20099,1000.);
#6010=VECTOR('',#20102,1000.);
#6011=VECTOR('',#20103,1000.);
#6012=VECTOR('',#20104,1000.);
#6013=VECTOR('',#20107,1000.);
#6014=VECTOR('',#20108,1000.);
#6015=VECTOR('',#20109,1000.);
#6016=VECTOR('',#20112,1000.);
#6017=VECTOR('',#20113,1000.);
#6018=VECTOR('',#20114,1000.);
#6019=VECTOR('',#20117,1000.);
#6020=VECTOR('',#20118,1000.);
#6021=VECTOR('',#20125,1000.);
#6022=VECTOR('',#20126,1000.);
#6023=VECTOR('',#20127,1000.);
#6024=VECTOR('',#20128,1000.);
#6025=VECTOR('',#20131,1000.);
#6026=VECTOR('',#20132,1000.);
#6027=VECTOR('',#20133,1000.);
#6028=VECTOR('',#20136,1000.);
#6029=VECTOR('',#20137,1000.);
#6030=VECTOR('',#20138,1000.);
#6031=VECTOR('',#20141,1000.);
#6032=VECTOR('',#20142,1000.);
#6033=VECTOR('',#20143,1000.);
#6034=VECTOR('',#20146,1000.);
#6035=VECTOR('',#20147,1000.);
#6036=VECTOR('',#20148,1000.);
#6037=VECTOR('',#20151,1000.);
#6038=VECTOR('',#20152,1000.);
#6039=VECTOR('',#20153,1000.);
#6040=VECTOR('',#20156,1000.);
#6041=VECTOR('',#20157,1000.);
#6042=VECTOR('',#20164,1000.);
#6043=VECTOR('',#20165,1000.);
#6044=VECTOR('',#20166,1000.);
#6045=VECTOR('',#20167,1000.);
#6046=VECTOR('',#20170,1000.);
#6047=VECTOR('',#20171,1000.);
#6048=VECTOR('',#20172,1000.);
#6049=VECTOR('',#20175,1000.);
#6050=VECTOR('',#20176,1000.);
#6051=VECTOR('',#20177,1000.);
#6052=VECTOR('',#20180,1000.);
#6053=VECTOR('',#20181,1000.);
#6054=VECTOR('',#20182,1000.);
#6055=VECTOR('',#20185,1000.);
#6056=VECTOR('',#20186,1000.);
#6057=VECTOR('',#20187,1000.);
#6058=VECTOR('',#20190,1000.);
#6059=VECTOR('',#20191,1000.);
#6060=VECTOR('',#20192,1000.);
#6061=VECTOR('',#20195,1000.);
#6062=VECTOR('',#20196,1000.);
#6063=VECTOR('',#20203,1000.);
#6064=VECTOR('',#20204,1000.);
#6065=VECTOR('',#20205,1000.);
#6066=VECTOR('',#20206,1000.);
#6067=VECTOR('',#20209,1000.);
#6068=VECTOR('',#20210,1000.);
#6069=VECTOR('',#20211,1000.);
#6070=VECTOR('',#20214,1000.);
#6071=VECTOR('',#20215,1000.);
#6072=VECTOR('',#20216,1000.);
#6073=VECTOR('',#20219,1000.);
#6074=VECTOR('',#20220,1000.);
#6075=VECTOR('',#20221,1000.);
#6076=VECTOR('',#20224,1000.);
#6077=VECTOR('',#20225,1000.);
#6078=VECTOR('',#20226,1000.);
#6079=VECTOR('',#20229,1000.);
#6080=VECTOR('',#20230,1000.);
#6081=VECTOR('',#20231,1000.);
#6082=VECTOR('',#20234,1000.);
#6083=VECTOR('',#20235,1000.);
#6084=VECTOR('',#20242,1000.);
#6085=VECTOR('',#20243,1000.);
#6086=VECTOR('',#20244,1000.);
#6087=VECTOR('',#20245,1000.);
#6088=VECTOR('',#20248,1000.);
#6089=VECTOR('',#20249,1000.);
#6090=VECTOR('',#20250,1000.);
#6091=VECTOR('',#20253,1000.);
#6092=VECTOR('',#20254,1000.);
#6093=VECTOR('',#20255,1000.);
#6094=VECTOR('',#20258,1000.);
#6095=VECTOR('',#20259,1000.);
#6096=VECTOR('',#20260,1000.);
#6097=VECTOR('',#20263,1000.);
#6098=VECTOR('',#20264,1000.);
#6099=VECTOR('',#20265,1000.);
#6100=VECTOR('',#20268,1000.);
#6101=VECTOR('',#20269,1000.);
#6102=VECTOR('',#20270,1000.);
#6103=VECTOR('',#20273,1000.);
#6104=VECTOR('',#20274,1000.);
#6105=VECTOR('',#20281,1000.);
#6106=VECTOR('',#20282,1000.);
#6107=VECTOR('',#20283,1000.);
#6108=VECTOR('',#20284,1000.);
#6109=VECTOR('',#20287,1000.);
#6110=VECTOR('',#20288,1000.);
#6111=VECTOR('',#20289,1000.);
#6112=VECTOR('',#20292,1000.);
#6113=VECTOR('',#20293,1000.);
#6114=VECTOR('',#20294,1000.);
#6115=VECTOR('',#20297,1000.);
#6116=VECTOR('',#20298,1000.);
#6117=VECTOR('',#20299,1000.);
#6118=VECTOR('',#20302,1000.);
#6119=VECTOR('',#20303,1000.);
#6120=VECTOR('',#20304,1000.);
#6121=VECTOR('',#20307,1000.);
#6122=VECTOR('',#20308,1000.);
#6123=VECTOR('',#20309,1000.);
#6124=VECTOR('',#20312,1000.);
#6125=VECTOR('',#20313,1000.);
#6126=VECTOR('',#20320,1000.);
#6127=VECTOR('',#20321,1000.);
#6128=VECTOR('',#20322,1000.);
#6129=VECTOR('',#20323,1000.);
#6130=VECTOR('',#20326,1000.);
#6131=VECTOR('',#20327,1000.);
#6132=VECTOR('',#20328,1000.);
#6133=VECTOR('',#20331,1000.);
#6134=VECTOR('',#20332,1000.);
#6135=VECTOR('',#20333,1000.);
#6136=VECTOR('',#20336,1000.);
#6137=VECTOR('',#20337,1000.);
#6138=VECTOR('',#20338,1000.);
#6139=VECTOR('',#20341,1000.);
#6140=VECTOR('',#20342,1000.);
#6141=VECTOR('',#20343,1000.);
#6142=VECTOR('',#20346,1000.);
#6143=VECTOR('',#20347,1000.);
#6144=VECTOR('',#20348,1000.);
#6145=VECTOR('',#20351,1000.);
#6146=VECTOR('',#20352,1000.);
#6147=VECTOR('',#20359,1000.);
#6148=VECTOR('',#20360,1000.);
#6149=VECTOR('',#20361,1000.);
#6150=VECTOR('',#20362,1000.);
#6151=VECTOR('',#20365,1000.);
#6152=VECTOR('',#20366,1000.);
#6153=VECTOR('',#20367,1000.);
#6154=VECTOR('',#20370,1000.);
#6155=VECTOR('',#20371,1000.);
#6156=VECTOR('',#20372,1000.);
#6157=VECTOR('',#20375,1000.);
#6158=VECTOR('',#20376,1000.);
#6159=VECTOR('',#20377,1000.);
#6160=VECTOR('',#20380,1000.);
#6161=VECTOR('',#20381,1000.);
#6162=VECTOR('',#20382,1000.);
#6163=VECTOR('',#20385,1000.);
#6164=VECTOR('',#20386,1000.);
#6165=VECTOR('',#20387,1000.);
#6166=VECTOR('',#20390,1000.);
#6167=VECTOR('',#20391,1000.);
#6168=VECTOR('',#20400,9.00000000000004);
#6169=VECTOR('',#20407,9.00000000000004);
#6170=VECTOR('',#20414,9.00000000000006);
#6171=VECTOR('',#20421,9.00000000000006);
#6172=VECTOR('',#20426,1000.);
#6173=VECTOR('',#20427,1000.);
#6174=VECTOR('',#20428,1000.);
#6175=VECTOR('',#20429,1000.);
#6176=VECTOR('',#20432,1000.);
#6177=VECTOR('',#20433,1000.);
#6178=VECTOR('',#20434,1000.);
#6179=VECTOR('',#20435,1000.);
#6180=VECTOR('',#20438,1000.);
#6181=VECTOR('',#20439,1000.);
#6182=VECTOR('',#20442,1000.);
#6183=VECTOR('',#20445,1000.);
#6184=VECTOR('',#20450,1000.);
#6185=VECTOR('',#20451,1000.);
#6186=VECTOR('',#20452,1000.);
#6187=VECTOR('',#20453,1000.);
#6188=VECTOR('',#20456,1000.);
#6189=VECTOR('',#20457,1000.);
#6190=VECTOR('',#20458,1000.);
#6191=VECTOR('',#20461,1000.);
#6192=VECTOR('',#20462,1000.);
#6193=VECTOR('',#20463,1000.);
#6194=VECTOR('',#20466,1000.);
#6195=VECTOR('',#20467,1000.);
#6196=VECTOR('',#20474,1000.);
#6197=VECTOR('',#20475,1000.);
#6198=VECTOR('',#20476,1000.);
#6199=VECTOR('',#20477,1000.);
#6200=VECTOR('',#20480,1000.);
#6201=VECTOR('',#20481,1000.);
#6202=VECTOR('',#20482,1000.);
#6203=VECTOR('',#20485,1000.);
#6204=VECTOR('',#20486,1000.);
#6205=VECTOR('',#20487,1000.);
#6206=VECTOR('',#20490,1000.);
#6207=VECTOR('',#20491,1000.);
#6208=VECTOR('',#20498,1000.);
#6209=VECTOR('',#20499,1000.);
#6210=VECTOR('',#20500,1000.);
#6211=VECTOR('',#20501,1000.);
#6212=VECTOR('',#20504,1000.);
#6213=VECTOR('',#20505,1000.);
#6214=VECTOR('',#20506,1000.);
#6215=VECTOR('',#20509,1000.);
#6216=VECTOR('',#20510,1000.);
#6217=VECTOR('',#20511,1000.);
#6218=VECTOR('',#20514,1000.);
#6219=VECTOR('',#20515,1000.);
#6220=VECTOR('',#20522,1000.);
#6221=VECTOR('',#20523,1000.);
#6222=VECTOR('',#20524,1000.);
#6223=VECTOR('',#20525,1000.);
#6224=VECTOR('',#20528,1000.);
#6225=VECTOR('',#20529,1000.);
#6226=VECTOR('',#20530,1000.);
#6227=VECTOR('',#20533,1000.);
#6228=VECTOR('',#20534,1000.);
#6229=VECTOR('',#20535,1000.);
#6230=VECTOR('',#20538,1000.);
#6231=VECTOR('',#20539,1000.);
#6232=VECTOR('',#20546,1000.);
#6233=VECTOR('',#20547,1000.);
#6234=VECTOR('',#20548,1000.);
#6235=VECTOR('',#20549,1000.);
#6236=VECTOR('',#20552,1000.);
#6237=VECTOR('',#20553,1000.);
#6238=VECTOR('',#20554,1000.);
#6239=VECTOR('',#20557,1000.);
#6240=VECTOR('',#20558,1000.);
#6241=VECTOR('',#20559,1000.);
#6242=VECTOR('',#20562,1000.);
#6243=VECTOR('',#20563,1000.);
#6244=VECTOR('',#20570,1000.);
#6245=VECTOR('',#20571,1000.);
#6246=VECTOR('',#20572,1000.);
#6247=VECTOR('',#20573,1000.);
#6248=VECTOR('',#20576,1000.);
#6249=VECTOR('',#20577,1000.);
#6250=VECTOR('',#20578,1000.);
#6251=VECTOR('',#20581,1000.);
#6252=VECTOR('',#20582,1000.);
#6253=VECTOR('',#20583,1000.);
#6254=VECTOR('',#20586,1000.);
#6255=VECTOR('',#20587,1000.);
#6256=VECTOR('',#20594,1000.);
#6257=VECTOR('',#20595,1000.);
#6258=VECTOR('',#20596,1000.);
#6259=VECTOR('',#20597,1000.);
#6260=VECTOR('',#20600,1000.);
#6261=VECTOR('',#20601,1000.);
#6262=VECTOR('',#20602,1000.);
#6263=VECTOR('',#20605,1000.);
#6264=VECTOR('',#20606,1000.);
#6265=VECTOR('',#20607,1000.);
#6266=VECTOR('',#20610,1000.);
#6267=VECTOR('',#20611,1000.);
#6268=VECTOR('',#20618,1000.);
#6269=VECTOR('',#20619,1000.);
#6270=VECTOR('',#20620,1000.);
#6271=VECTOR('',#20621,1000.);
#6272=VECTOR('',#20624,1000.);
#6273=VECTOR('',#20625,1000.);
#6274=VECTOR('',#20626,1000.);
#6275=VECTOR('',#20629,1000.);
#6276=VECTOR('',#20630,1000.);
#6277=VECTOR('',#20631,1000.);
#6278=VECTOR('',#20634,1000.);
#6279=VECTOR('',#20635,1000.);
#6280=VECTOR('',#20642,1000.);
#6281=VECTOR('',#20643,1000.);
#6282=VECTOR('',#20644,1000.);
#6283=VECTOR('',#20645,1000.);
#6284=VECTOR('',#20648,1000.);
#6285=VECTOR('',#20649,1000.);
#6286=VECTOR('',#20650,1000.);
#6287=VECTOR('',#20653,1000.);
#6288=VECTOR('',#20654,1000.);
#6289=VECTOR('',#20655,1000.);
#6290=VECTOR('',#20658,1000.);
#6291=VECTOR('',#20659,1000.);
#6292=VECTOR('',#20666,1000.);
#6293=VECTOR('',#20667,1000.);
#6294=VECTOR('',#20668,1000.);
#6295=VECTOR('',#20669,1000.);
#6296=VECTOR('',#20672,1000.);
#6297=VECTOR('',#20673,1000.);
#6298=VECTOR('',#20674,1000.);
#6299=VECTOR('',#20677,1000.);
#6300=VECTOR('',#20678,1000.);
#6301=VECTOR('',#20679,1000.);
#6302=VECTOR('',#20682,1000.);
#6303=VECTOR('',#20683,1000.);
#6304=VECTOR('',#20690,1000.);
#6305=VECTOR('',#20691,1000.);
#6306=VECTOR('',#20692,1000.);
#6307=VECTOR('',#20693,1000.);
#6308=VECTOR('',#20696,1000.);
#6309=VECTOR('',#20697,1000.);
#6310=VECTOR('',#20698,1000.);
#6311=VECTOR('',#20701,1000.);
#6312=VECTOR('',#20702,1000.);
#6313=VECTOR('',#20703,1000.);
#6314=VECTOR('',#20706,1000.);
#6315=VECTOR('',#20707,1000.);
#6316=VECTOR('',#20714,1000.);
#6317=VECTOR('',#20715,1000.);
#6318=VECTOR('',#20716,1000.);
#6319=VECTOR('',#20717,1000.);
#6320=VECTOR('',#20720,1000.);
#6321=VECTOR('',#20721,1000.);
#6322=VECTOR('',#20722,1000.);
#6323=VECTOR('',#20725,1000.);
#6324=VECTOR('',#20726,1000.);
#6325=VECTOR('',#20727,1000.);
#6326=VECTOR('',#20730,1000.);
#6327=VECTOR('',#20731,1000.);
#6328=VECTOR('',#20738,1000.);
#6329=VECTOR('',#20739,1000.);
#6330=VECTOR('',#20740,1000.);
#6331=VECTOR('',#20741,1000.);
#6332=VECTOR('',#20744,1000.);
#6333=VECTOR('',#20745,1000.);
#6334=VECTOR('',#20746,1000.);
#6335=VECTOR('',#20749,1000.);
#6336=VECTOR('',#20750,1000.);
#6337=VECTOR('',#20751,1000.);
#6338=VECTOR('',#20754,1000.);
#6339=VECTOR('',#20755,1000.);
#6340=VECTOR('',#20762,1000.);
#6341=VECTOR('',#20763,1000.);
#6342=VECTOR('',#20764,1000.);
#6343=VECTOR('',#20765,1000.);
#6344=VECTOR('',#20768,1000.);
#6345=VECTOR('',#20769,1000.);
#6346=VECTOR('',#20770,1000.);
#6347=VECTOR('',#20773,1000.);
#6348=VECTOR('',#20774,1000.);
#6349=VECTOR('',#20775,1000.);
#6350=VECTOR('',#20778,1000.);
#6351=VECTOR('',#20779,1000.);
#6352=VECTOR('',#20786,1000.);
#6353=VECTOR('',#20787,1000.);
#6354=VECTOR('',#20788,1000.);
#6355=VECTOR('',#20789,1000.);
#6356=VECTOR('',#20792,1000.);
#6357=VECTOR('',#20793,1000.);
#6358=VECTOR('',#20794,1000.);
#6359=VECTOR('',#20797,1000.);
#6360=VECTOR('',#20798,1000.);
#6361=VECTOR('',#20799,1000.);
#6362=VECTOR('',#20802,1000.);
#6363=VECTOR('',#20803,1000.);
#6364=VECTOR('',#20810,1000.);
#6365=VECTOR('',#20811,1000.);
#6366=VECTOR('',#20812,1000.);
#6367=VECTOR('',#20813,1000.);
#6368=VECTOR('',#20816,1000.);
#6369=VECTOR('',#20817,1000.);
#6370=VECTOR('',#20818,1000.);
#6371=VECTOR('',#20821,1000.);
#6372=VECTOR('',#20822,1000.);
#6373=VECTOR('',#20823,1000.);
#6374=VECTOR('',#20826,1000.);
#6375=VECTOR('',#20827,1000.);
#6376=VECTOR('',#20834,1000.);
#6377=VECTOR('',#20835,1000.);
#6378=VECTOR('',#20836,1000.);
#6379=VECTOR('',#20837,1000.);
#6380=VECTOR('',#20840,1000.);
#6381=VECTOR('',#20841,1000.);
#6382=VECTOR('',#20842,1000.);
#6383=VECTOR('',#20845,1000.);
#6384=VECTOR('',#20846,1000.);
#6385=VECTOR('',#20847,1000.);
#6386=VECTOR('',#20850,1000.);
#6387=VECTOR('',#20851,1000.);
#6388=VECTOR('',#20858,1000.);
#6389=VECTOR('',#20859,1000.);
#6390=VECTOR('',#20860,1000.);
#6391=VECTOR('',#20861,1000.);
#6392=VECTOR('',#20864,1000.);
#6393=VECTOR('',#20865,1000.);
#6394=VECTOR('',#20866,1000.);
#6395=VECTOR('',#20869,1000.);
#6396=VECTOR('',#20870,1000.);
#6397=VECTOR('',#20871,1000.);
#6398=VECTOR('',#20874,1000.);
#6399=VECTOR('',#20875,1000.);
#6400=VECTOR('',#20882,1000.);
#6401=VECTOR('',#20883,1000.);
#6402=VECTOR('',#20884,1000.);
#6403=VECTOR('',#20885,1000.);
#6404=VECTOR('',#20888,1000.);
#6405=VECTOR('',#20889,1000.);
#6406=VECTOR('',#20890,1000.);
#6407=VECTOR('',#20893,1000.);
#6408=VECTOR('',#20894,1000.);
#6409=VECTOR('',#20895,1000.);
#6410=VECTOR('',#20898,1000.);
#6411=VECTOR('',#20899,1000.);
#6412=VECTOR('',#20906,1000.);
#6413=VECTOR('',#20907,1000.);
#6414=VECTOR('',#20908,1000.);
#6415=VECTOR('',#20909,1000.);
#6416=VECTOR('',#20912,1000.);
#6417=VECTOR('',#20913,1000.);
#6418=VECTOR('',#20914,1000.);
#6419=VECTOR('',#20917,1000.);
#6420=VECTOR('',#20918,1000.);
#6421=VECTOR('',#20919,1000.);
#6422=VECTOR('',#20922,1000.);
#6423=VECTOR('',#20923,1000.);
#6424=VECTOR('',#20930,1000.);
#6425=VECTOR('',#20931,1000.);
#6426=VECTOR('',#20932,1000.);
#6427=VECTOR('',#20933,1000.);
#6428=VECTOR('',#20936,1000.);
#6429=VECTOR('',#20937,1000.);
#6430=VECTOR('',#20938,1000.);
#6431=VECTOR('',#20941,1000.);
#6432=VECTOR('',#20942,1000.);
#6433=VECTOR('',#20943,1000.);
#6434=VECTOR('',#20946,1000.);
#6435=VECTOR('',#20947,1000.);
#6436=VECTOR('',#20954,1000.);
#6437=VECTOR('',#20955,1000.);
#6438=VECTOR('',#20956,1000.);
#6439=VECTOR('',#20957,1000.);
#6440=VECTOR('',#20960,1000.);
#6441=VECTOR('',#20961,1000.);
#6442=VECTOR('',#20962,1000.);
#6443=VECTOR('',#20965,1000.);
#6444=VECTOR('',#20966,1000.);
#6445=VECTOR('',#20967,1000.);
#6446=VECTOR('',#20970,1000.);
#6447=VECTOR('',#20971,1000.);
#7204=VERTEX_POINT('',#30707);
#7205=VERTEX_POINT('',#30708);
#7206=VERTEX_POINT('',#30710);
#7207=VERTEX_POINT('',#30712);
#7208=VERTEX_POINT('',#30716);
#7209=VERTEX_POINT('',#30718);
#7210=VERTEX_POINT('',#30722);
#7211=VERTEX_POINT('',#30724);
#7212=VERTEX_POINT('',#30733);
#7213=VERTEX_POINT('',#30735);
#7214=VERTEX_POINT('',#30739);
#7215=VERTEX_POINT('',#30740);
#7216=VERTEX_POINT('',#30742);
#7217=VERTEX_POINT('',#30744);
#7218=VERTEX_POINT('',#30746);
#7219=VERTEX_POINT('',#30748);
#7220=VERTEX_POINT('',#30752);
#7221=VERTEX_POINT('',#30753);
#7222=VERTEX_POINT('',#30755);
#7223=VERTEX_POINT('',#30757);
#7224=VERTEX_POINT('',#30759);
#7225=VERTEX_POINT('',#30761);
#7226=VERTEX_POINT('',#30777);
#7227=VERTEX_POINT('',#30779);
#7228=VERTEX_POINT('',#30783);
#7229=VERTEX_POINT('',#30784);
#7230=VERTEX_POINT('',#30786);
#7231=VERTEX_POINT('',#30788);
#7232=VERTEX_POINT('',#30790);
#7233=VERTEX_POINT('',#30792);
#7234=VERTEX_POINT('',#30796);
#7235=VERTEX_POINT('',#30797);
#7236=VERTEX_POINT('',#30799);
#7237=VERTEX_POINT('',#30801);
#7238=VERTEX_POINT('',#30803);
#7239=VERTEX_POINT('',#30805);
#7240=VERTEX_POINT('',#30821);
#7241=VERTEX_POINT('',#30823);
#7242=VERTEX_POINT('',#30827);
#7243=VERTEX_POINT('',#30829);
#7244=VERTEX_POINT('',#30833);
#7245=VERTEX_POINT('',#30835);
#7246=VERTEX_POINT('',#30839);
#7247=VERTEX_POINT('',#30841);
#7248=VERTEX_POINT('',#30845);
#7249=VERTEX_POINT('',#30847);
#7250=VERTEX_POINT('',#30851);
#7251=VERTEX_POINT('',#30852);
#7252=VERTEX_POINT('',#30854);
#7253=VERTEX_POINT('',#30856);
#7254=VERTEX_POINT('',#30858);
#7255=VERTEX_POINT('',#30860);
#7256=VERTEX_POINT('',#30862);
#7257=VERTEX_POINT('',#30864);
#7258=VERTEX_POINT('',#30868);
#7259=VERTEX_POINT('',#30869);
#7260=VERTEX_POINT('',#30871);
#7261=VERTEX_POINT('',#30873);
#7262=VERTEX_POINT('',#30875);
#7263=VERTEX_POINT('',#30877);
#7264=VERTEX_POINT('',#30879);
#7265=VERTEX_POINT('',#30881);
#7266=VERTEX_POINT('',#30901);
#7267=VERTEX_POINT('',#30902);
#7268=VERTEX_POINT('',#30904);
#7269=VERTEX_POINT('',#30906);
#7270=VERTEX_POINT('',#30910);
#7271=VERTEX_POINT('',#30912);
#7272=VERTEX_POINT('',#30916);
#7273=VERTEX_POINT('',#30918);
#7274=VERTEX_POINT('',#30927);
#7275=VERTEX_POINT('',#30928);
#7276=VERTEX_POINT('',#30930);
#7277=VERTEX_POINT('',#30932);
#7278=VERTEX_POINT('',#30936);
#7279=VERTEX_POINT('',#30938);
#7280=VERTEX_POINT('',#30942);
#7281=VERTEX_POINT('',#30944);
#7282=VERTEX_POINT('',#30953);
#7283=VERTEX_POINT('',#30954);
#7284=VERTEX_POINT('',#30956);
#7285=VERTEX_POINT('',#30958);
#7286=VERTEX_POINT('',#30962);
#7287=VERTEX_POINT('',#30964);
#7288=VERTEX_POINT('',#30968);
#7289=VERTEX_POINT('',#30970);
#7290=VERTEX_POINT('',#30974);
#7291=VERTEX_POINT('',#30976);
#7292=VERTEX_POINT('',#30980);
#7293=VERTEX_POINT('',#30982);
#7294=VERTEX_POINT('',#30991);
#7295=VERTEX_POINT('',#30993);
#7296=VERTEX_POINT('',#30997);
#7297=VERTEX_POINT('',#30999);
#7298=VERTEX_POINT('',#31003);
#7299=VERTEX_POINT('',#31005);
#7300=VERTEX_POINT('',#31009);
#7301=VERTEX_POINT('',#31010);
#7302=VERTEX_POINT('',#31012);
#7303=VERTEX_POINT('',#31014);
#7304=VERTEX_POINT('',#31018);
#7305=VERTEX_POINT('',#31019);
#7306=VERTEX_POINT('',#31021);
#7307=VERTEX_POINT('',#31023);
#7308=VERTEX_POINT('',#31035);
#7309=VERTEX_POINT('',#31037);
#7310=VERTEX_POINT('',#31041);
#7311=VERTEX_POINT('',#31043);
#7312=VERTEX_POINT('',#31047);
#7313=VERTEX_POINT('',#31049);
#7314=VERTEX_POINT('',#31053);
#7315=VERTEX_POINT('',#31054);
#7316=VERTEX_POINT('',#31056);
#7317=VERTEX_POINT('',#31058);
#7318=VERTEX_POINT('',#31062);
#7319=VERTEX_POINT('',#31063);
#7320=VERTEX_POINT('',#31065);
#7321=VERTEX_POINT('',#31067);
#7322=VERTEX_POINT('',#31079);
#7323=VERTEX_POINT('',#31081);
#7324=VERTEX_POINT('',#31085);
#7325=VERTEX_POINT('',#31087);
#7326=VERTEX_POINT('',#31091);
#7327=VERTEX_POINT('',#31093);
#7328=VERTEX_POINT('',#31097);
#7329=VERTEX_POINT('',#31098);
#7330=VERTEX_POINT('',#31100);
#7331=VERTEX_POINT('',#31102);
#7332=VERTEX_POINT('',#31106);
#7333=VERTEX_POINT('',#31107);
#7334=VERTEX_POINT('',#31109);
#7335=VERTEX_POINT('',#31111);
#7336=VERTEX_POINT('',#31123);
#7337=VERTEX_POINT('',#31125);
#7338=VERTEX_POINT('',#31129);
#7339=VERTEX_POINT('',#31131);
#7340=VERTEX_POINT('',#31135);
#7341=VERTEX_POINT('',#31137);
#7342=VERTEX_POINT('',#31141);
#7343=VERTEX_POINT('',#31142);
#7344=VERTEX_POINT('',#31144);
#7345=VERTEX_POINT('',#31146);
#7346=VERTEX_POINT('',#31150);
#7347=VERTEX_POINT('',#31151);
#7348=VERTEX_POINT('',#31153);
#7349=VERTEX_POINT('',#31155);
#7350=VERTEX_POINT('',#31167);
#7351=VERTEX_POINT('',#31168);
#7352=VERTEX_POINT('',#31170);
#7353=VERTEX_POINT('',#31172);
#7354=VERTEX_POINT('',#31176);
#7355=VERTEX_POINT('',#31178);
#7356=VERTEX_POINT('',#31182);
#7357=VERTEX_POINT('',#31184);
#7358=VERTEX_POINT('',#31193);
#7359=VERTEX_POINT('',#31194);
#7360=VERTEX_POINT('',#31196);
#7361=VERTEX_POINT('',#31198);
#7362=VERTEX_POINT('',#31202);
#7363=VERTEX_POINT('',#31204);
#7364=VERTEX_POINT('',#31208);
#7365=VERTEX_POINT('',#31210);
#7366=VERTEX_POINT('',#31219);
#7367=VERTEX_POINT('',#31220);
#7368=VERTEX_POINT('',#31222);
#7369=VERTEX_POINT('',#31224);
#7370=VERTEX_POINT('',#31228);
#7371=VERTEX_POINT('',#31230);
#7372=VERTEX_POINT('',#31234);
#7373=VERTEX_POINT('',#31236);
#7374=VERTEX_POINT('',#31245);
#7375=VERTEX_POINT('',#31246);
#7376=VERTEX_POINT('',#31248);
#7377=VERTEX_POINT('',#31250);
#7378=VERTEX_POINT('',#31254);
#7379=VERTEX_POINT('',#31256);
#7380=VERTEX_POINT('',#31260);
#7381=VERTEX_POINT('',#31262);
#7382=VERTEX_POINT('',#31271);
#7383=VERTEX_POINT('',#31272);
#7384=VERTEX_POINT('',#31274);
#7385=VERTEX_POINT('',#31276);
#7386=VERTEX_POINT('',#31280);
#7387=VERTEX_POINT('',#31282);
#7388=VERTEX_POINT('',#31286);
#7389=VERTEX_POINT('',#31288);
#7390=VERTEX_POINT('',#31297);
#7391=VERTEX_POINT('',#31299);
#7392=VERTEX_POINT('',#31303);
#7393=VERTEX_POINT('',#31305);
#7394=VERTEX_POINT('',#31309);
#7395=VERTEX_POINT('',#31311);
#7396=VERTEX_POINT('',#31315);
#7397=VERTEX_POINT('',#31317);
#7398=VERTEX_POINT('',#31321);
#7399=VERTEX_POINT('',#31322);
#7400=VERTEX_POINT('',#31324);
#7401=VERTEX_POINT('',#31326);
#7402=VERTEX_POINT('',#31330);
#7403=VERTEX_POINT('',#31331);
#7404=VERTEX_POINT('',#31333);
#7405=VERTEX_POINT('',#31335);
#7406=VERTEX_POINT('',#31347);
#7407=VERTEX_POINT('',#31349);
#7408=VERTEX_POINT('',#31353);
#7409=VERTEX_POINT('',#31355);
#7410=VERTEX_POINT('',#31359);
#7411=VERTEX_POINT('',#31361);
#7412=VERTEX_POINT('',#31365);
#7413=VERTEX_POINT('',#31367);
#7414=VERTEX_POINT('',#31371);
#7415=VERTEX_POINT('',#31373);
#7416=VERTEX_POINT('',#31377);
#7417=VERTEX_POINT('',#31379);
#7418=VERTEX_POINT('',#31383);
#7419=VERTEX_POINT('',#31384);
#7420=VERTEX_POINT('',#31386);
#7421=VERTEX_POINT('',#31388);
#7422=VERTEX_POINT('',#31392);
#7423=VERTEX_POINT('',#31394);
#7424=VERTEX_POINT('',#31398);
#7425=VERTEX_POINT('',#31400);
#7426=VERTEX_POINT('',#31409);
#7427=VERTEX_POINT('',#31410);
#7428=VERTEX_POINT('',#31412);
#7429=VERTEX_POINT('',#31414);
#7430=VERTEX_POINT('',#31418);
#7431=VERTEX_POINT('',#31420);
#7432=VERTEX_POINT('',#31424);
#7433=VERTEX_POINT('',#31426);
#7434=VERTEX_POINT('',#31430);
#7435=VERTEX_POINT('',#31432);
#7436=VERTEX_POINT('',#31436);
#7437=VERTEX_POINT('',#31438);
#7438=VERTEX_POINT('',#31442);
#7439=VERTEX_POINT('',#31444);
#7440=VERTEX_POINT('',#31453);
#7441=VERTEX_POINT('',#31454);
#7442=VERTEX_POINT('',#31456);
#7443=VERTEX_POINT('',#31458);
#7444=VERTEX_POINT('',#31462);
#7445=VERTEX_POINT('',#31464);
#7446=VERTEX_POINT('',#31468);
#7447=VERTEX_POINT('',#31470);
#7448=VERTEX_POINT('',#31474);
#7449=VERTEX_POINT('',#31476);
#7450=VERTEX_POINT('',#31480);
#7451=VERTEX_POINT('',#31482);
#7452=VERTEX_POINT('',#31486);
#7453=VERTEX_POINT('',#31488);
#7454=VERTEX_POINT('',#31497);
#7455=VERTEX_POINT('',#31498);
#7456=VERTEX_POINT('',#31500);
#7457=VERTEX_POINT('',#31502);
#7458=VERTEX_POINT('',#31506);
#7459=VERTEX_POINT('',#31508);
#7460=VERTEX_POINT('',#31512);
#7461=VERTEX_POINT('',#31514);
#7462=VERTEX_POINT('',#31518);
#7463=VERTEX_POINT('',#31520);
#7464=VERTEX_POINT('',#31524);
#7465=VERTEX_POINT('',#31526);
#7466=VERTEX_POINT('',#31530);
#7467=VERTEX_POINT('',#31532);
#7468=VERTEX_POINT('',#31541);
#7469=VERTEX_POINT('',#31542);
#7470=VERTEX_POINT('',#31544);
#7471=VERTEX_POINT('',#31546);
#7472=VERTEX_POINT('',#31550);
#7473=VERTEX_POINT('',#31552);
#7474=VERTEX_POINT('',#31556);
#7475=VERTEX_POINT('',#31558);
#7476=VERTEX_POINT('',#31562);
#7477=VERTEX_POINT('',#31564);
#7478=VERTEX_POINT('',#31568);
#7479=VERTEX_POINT('',#31570);
#7480=VERTEX_POINT('',#31574);
#7481=VERTEX_POINT('',#31576);
#7482=VERTEX_POINT('',#31585);
#7483=VERTEX_POINT('',#31586);
#7484=VERTEX_POINT('',#31588);
#7485=VERTEX_POINT('',#31590);
#7486=VERTEX_POINT('',#31594);
#7487=VERTEX_POINT('',#31596);
#7488=VERTEX_POINT('',#31600);
#7489=VERTEX_POINT('',#31602);
#7490=VERTEX_POINT('',#31606);
#7491=VERTEX_POINT('',#31608);
#7492=VERTEX_POINT('',#31612);
#7493=VERTEX_POINT('',#31614);
#7494=VERTEX_POINT('',#31618);
#7495=VERTEX_POINT('',#31620);
#7496=VERTEX_POINT('',#31629);
#7497=VERTEX_POINT('',#31630);
#7498=VERTEX_POINT('',#31632);
#7499=VERTEX_POINT('',#31634);
#7500=VERTEX_POINT('',#31638);
#7501=VERTEX_POINT('',#31640);
#7502=VERTEX_POINT('',#31644);
#7503=VERTEX_POINT('',#31646);
#7504=VERTEX_POINT('',#31650);
#7505=VERTEX_POINT('',#31652);
#7506=VERTEX_POINT('',#31656);
#7507=VERTEX_POINT('',#31658);
#7508=VERTEX_POINT('',#31662);
#7509=VERTEX_POINT('',#31664);
#7510=VERTEX_POINT('',#31673);
#7511=VERTEX_POINT('',#31674);
#7512=VERTEX_POINT('',#31676);
#7513=VERTEX_POINT('',#31678);
#7514=VERTEX_POINT('',#31682);
#7515=VERTEX_POINT('',#31684);
#7516=VERTEX_POINT('',#31688);
#7517=VERTEX_POINT('',#31690);
#7518=VERTEX_POINT('',#31694);
#7519=VERTEX_POINT('',#31696);
#7520=VERTEX_POINT('',#31700);
#7521=VERTEX_POINT('',#31702);
#7522=VERTEX_POINT('',#31706);
#7523=VERTEX_POINT('',#31708);
#7524=VERTEX_POINT('',#31717);
#7525=VERTEX_POINT('',#31718);
#7526=VERTEX_POINT('',#31720);
#7527=VERTEX_POINT('',#31722);
#7528=VERTEX_POINT('',#31726);
#7529=VERTEX_POINT('',#31728);
#7530=VERTEX_POINT('',#31732);
#7531=VERTEX_POINT('',#31734);
#7532=VERTEX_POINT('',#31738);
#7533=VERTEX_POINT('',#31740);
#7534=VERTEX_POINT('',#31744);
#7535=VERTEX_POINT('',#31746);
#7536=VERTEX_POINT('',#31750);
#7537=VERTEX_POINT('',#31752);
#7538=VERTEX_POINT('',#31761);
#7539=VERTEX_POINT('',#31762);
#7540=VERTEX_POINT('',#31764);
#7541=VERTEX_POINT('',#31766);
#7542=VERTEX_POINT('',#31770);
#7543=VERTEX_POINT('',#31772);
#7544=VERTEX_POINT('',#31776);
#7545=VERTEX_POINT('',#31778);
#7546=VERTEX_POINT('',#31782);
#7547=VERTEX_POINT('',#31784);
#7548=VERTEX_POINT('',#31788);
#7549=VERTEX_POINT('',#31790);
#7550=VERTEX_POINT('',#31794);
#7551=VERTEX_POINT('',#31796);
#7552=VERTEX_POINT('',#31805);
#7553=VERTEX_POINT('',#31806);
#7554=VERTEX_POINT('',#31808);
#7555=VERTEX_POINT('',#31810);
#7556=VERTEX_POINT('',#31814);
#7557=VERTEX_POINT('',#31816);
#7558=VERTEX_POINT('',#31820);
#7559=VERTEX_POINT('',#31822);
#7560=VERTEX_POINT('',#31826);
#7561=VERTEX_POINT('',#31828);
#7562=VERTEX_POINT('',#31832);
#7563=VERTEX_POINT('',#31834);
#7564=VERTEX_POINT('',#31838);
#7565=VERTEX_POINT('',#31840);
#7566=VERTEX_POINT('',#31849);
#7567=VERTEX_POINT('',#31850);
#7568=VERTEX_POINT('',#31852);
#7569=VERTEX_POINT('',#31854);
#7570=VERTEX_POINT('',#31858);
#7571=VERTEX_POINT('',#31860);
#7572=VERTEX_POINT('',#31864);
#7573=VERTEX_POINT('',#31866);
#7574=VERTEX_POINT('',#31870);
#7575=VERTEX_POINT('',#31872);
#7576=VERTEX_POINT('',#31876);
#7577=VERTEX_POINT('',#31878);
#7578=VERTEX_POINT('',#31882);
#7579=VERTEX_POINT('',#31884);
#7580=VERTEX_POINT('',#31893);
#7581=VERTEX_POINT('',#31895);
#7582=VERTEX_POINT('',#31899);
#7583=VERTEX_POINT('',#31901);
#7584=VERTEX_POINT('',#31905);
#7585=VERTEX_POINT('',#31907);
#7586=VERTEX_POINT('',#31911);
#7587=VERTEX_POINT('',#31913);
#7588=VERTEX_POINT('',#31917);
#7589=VERTEX_POINT('',#31918);
#7590=VERTEX_POINT('',#31920);
#7591=VERTEX_POINT('',#31922);
#7592=VERTEX_POINT('',#31926);
#7593=VERTEX_POINT('',#31927);
#7594=VERTEX_POINT('',#31929);
#7595=VERTEX_POINT('',#31931);
#7596=VERTEX_POINT('',#31943);
#7597=VERTEX_POINT('',#31944);
#7598=VERTEX_POINT('',#31946);
#7599=VERTEX_POINT('',#31948);
#7600=VERTEX_POINT('',#31952);
#7601=VERTEX_POINT('',#31954);
#7602=VERTEX_POINT('',#31958);
#7603=VERTEX_POINT('',#31960);
#7604=VERTEX_POINT('',#31969);
#7605=VERTEX_POINT('',#31970);
#7606=VERTEX_POINT('',#31972);
#7607=VERTEX_POINT('',#31974);
#7608=VERTEX_POINT('',#31978);
#7609=VERTEX_POINT('',#31980);
#7610=VERTEX_POINT('',#31984);
#7611=VERTEX_POINT('',#31986);
#7612=VERTEX_POINT('',#31995);
#7613=VERTEX_POINT('',#31996);
#7614=VERTEX_POINT('',#31998);
#7615=VERTEX_POINT('',#32000);
#7616=VERTEX_POINT('',#32004);
#7617=VERTEX_POINT('',#32006);
#7618=VERTEX_POINT('',#32010);
#7619=VERTEX_POINT('',#32012);
#7620=VERTEX_POINT('',#32021);
#7621=VERTEX_POINT('',#32022);
#7622=VERTEX_POINT('',#32024);
#7623=VERTEX_POINT('',#32026);
#7624=VERTEX_POINT('',#32030);
#7625=VERTEX_POINT('',#32032);
#7626=VERTEX_POINT('',#32036);
#7627=VERTEX_POINT('',#32038);
#7628=VERTEX_POINT('',#32047);
#7629=VERTEX_POINT('',#32048);
#7630=VERTEX_POINT('',#32050);
#7631=VERTEX_POINT('',#32052);
#7632=VERTEX_POINT('',#32056);
#7633=VERTEX_POINT('',#32058);
#7634=VERTEX_POINT('',#32062);
#7635=VERTEX_POINT('',#32064);
#7636=VERTEX_POINT('',#32073);
#7637=VERTEX_POINT('',#32074);
#7638=VERTEX_POINT('',#32076);
#7639=VERTEX_POINT('',#32078);
#7640=VERTEX_POINT('',#32082);
#7641=VERTEX_POINT('',#32084);
#7642=VERTEX_POINT('',#32088);
#7643=VERTEX_POINT('',#32090);
#7644=VERTEX_POINT('',#32099);
#7645=VERTEX_POINT('',#32100);
#7646=VERTEX_POINT('',#32102);
#7647=VERTEX_POINT('',#32104);
#7648=VERTEX_POINT('',#32108);
#7649=VERTEX_POINT('',#32110);
#7650=VERTEX_POINT('',#32114);
#7651=VERTEX_POINT('',#32116);
#7652=VERTEX_POINT('',#32125);
#7653=VERTEX_POINT('',#32126);
#7654=VERTEX_POINT('',#32128);
#7655=VERTEX_POINT('',#32130);
#7656=VERTEX_POINT('',#32134);
#7657=VERTEX_POINT('',#32136);
#7658=VERTEX_POINT('',#32140);
#7659=VERTEX_POINT('',#32142);
#7660=VERTEX_POINT('',#32151);
#7661=VERTEX_POINT('',#32152);
#7662=VERTEX_POINT('',#32154);
#7663=VERTEX_POINT('',#32156);
#7664=VERTEX_POINT('',#32160);
#7665=VERTEX_POINT('',#32162);
#7666=VERTEX_POINT('',#32166);
#7667=VERTEX_POINT('',#32168);
#7668=VERTEX_POINT('',#32177);
#7669=VERTEX_POINT('',#32178);
#7670=VERTEX_POINT('',#32180);
#7671=VERTEX_POINT('',#32182);
#7672=VERTEX_POINT('',#32186);
#7673=VERTEX_POINT('',#32188);
#7674=VERTEX_POINT('',#32192);
#7675=VERTEX_POINT('',#32194);
#7676=VERTEX_POINT('',#32203);
#7677=VERTEX_POINT('',#32204);
#7678=VERTEX_POINT('',#32206);
#7679=VERTEX_POINT('',#32208);
#7680=VERTEX_POINT('',#32212);
#7681=VERTEX_POINT('',#32214);
#7682=VERTEX_POINT('',#32218);
#7683=VERTEX_POINT('',#32220);
#7684=VERTEX_POINT('',#32229);
#7685=VERTEX_POINT('',#32230);
#7686=VERTEX_POINT('',#32232);
#7687=VERTEX_POINT('',#32234);
#7688=VERTEX_POINT('',#32238);
#7689=VERTEX_POINT('',#32240);
#7690=VERTEX_POINT('',#32244);
#7691=VERTEX_POINT('',#32246);
#7692=VERTEX_POINT('',#32255);
#7693=VERTEX_POINT('',#32256);
#7694=VERTEX_POINT('',#32258);
#7695=VERTEX_POINT('',#32260);
#7696=VERTEX_POINT('',#32264);
#7697=VERTEX_POINT('',#32266);
#7698=VERTEX_POINT('',#32270);
#7699=VERTEX_POINT('',#32272);
#7700=VERTEX_POINT('',#32281);
#7701=VERTEX_POINT('',#32282);
#7702=VERTEX_POINT('',#32284);
#7703=VERTEX_POINT('',#32286);
#7704=VERTEX_POINT('',#32290);
#7705=VERTEX_POINT('',#32292);
#7706=VERTEX_POINT('',#32296);
#7707=VERTEX_POINT('',#32298);
#7708=VERTEX_POINT('',#32307);
#7709=VERTEX_POINT('',#32308);
#7710=VERTEX_POINT('',#32310);
#7711=VERTEX_POINT('',#32312);
#7712=VERTEX_POINT('',#32316);
#7713=VERTEX_POINT('',#32318);
#7714=VERTEX_POINT('',#32322);
#7715=VERTEX_POINT('',#32324);
#7716=VERTEX_POINT('',#32333);
#7717=VERTEX_POINT('',#32334);
#7718=VERTEX_POINT('',#32336);
#7719=VERTEX_POINT('',#32338);
#7720=VERTEX_POINT('',#32342);
#7721=VERTEX_POINT('',#32344);
#7722=VERTEX_POINT('',#32348);
#7723=VERTEX_POINT('',#32350);
#7724=VERTEX_POINT('',#32359);
#7725=VERTEX_POINT('',#32360);
#7726=VERTEX_POINT('',#32362);
#7727=VERTEX_POINT('',#32364);
#7728=VERTEX_POINT('',#32368);
#7729=VERTEX_POINT('',#32370);
#7730=VERTEX_POINT('',#32374);
#7731=VERTEX_POINT('',#32376);
#7732=VERTEX_POINT('',#32385);
#7733=VERTEX_POINT('',#32386);
#7734=VERTEX_POINT('',#32388);
#7735=VERTEX_POINT('',#32390);
#7736=VERTEX_POINT('',#32394);
#7737=VERTEX_POINT('',#32396);
#7738=VERTEX_POINT('',#32400);
#7739=VERTEX_POINT('',#32402);
#7740=VERTEX_POINT('',#32411);
#7741=VERTEX_POINT('',#32412);
#7742=VERTEX_POINT('',#32414);
#7743=VERTEX_POINT('',#32416);
#7744=VERTEX_POINT('',#32420);
#7745=VERTEX_POINT('',#32422);
#7746=VERTEX_POINT('',#32426);
#7747=VERTEX_POINT('',#32428);
#7748=VERTEX_POINT('',#32437);
#7749=VERTEX_POINT('',#32438);
#7750=VERTEX_POINT('',#32440);
#7751=VERTEX_POINT('',#32442);
#7752=VERTEX_POINT('',#32446);
#7753=VERTEX_POINT('',#32448);
#7754=VERTEX_POINT('',#32452);
#7755=VERTEX_POINT('',#32454);
#7756=VERTEX_POINT('',#32463);
#7757=VERTEX_POINT('',#32464);
#7758=VERTEX_POINT('',#32466);
#7759=VERTEX_POINT('',#32468);
#7760=VERTEX_POINT('',#32472);
#7761=VERTEX_POINT('',#32474);
#7762=VERTEX_POINT('',#32478);
#7763=VERTEX_POINT('',#32480);
#7764=VERTEX_POINT('',#32489);
#7765=VERTEX_POINT('',#32490);
#7766=VERTEX_POINT('',#32492);
#7767=VERTEX_POINT('',#32494);
#7768=VERTEX_POINT('',#32498);
#7769=VERTEX_POINT('',#32500);
#7770=VERTEX_POINT('',#32504);
#7771=VERTEX_POINT('',#32506);
#8944=EDGE_CURVE('',#7204,#7205,#4262,.T.);
#8945=EDGE_CURVE('',#7206,#7205,#4263,.T.);
#8946=EDGE_CURVE('',#7207,#7206,#4264,.T.);
#8947=EDGE_CURVE('',#7207,#7204,#4265,.T.);
#8948=EDGE_CURVE('',#7205,#7208,#4266,.T.);
#8949=EDGE_CURVE('',#7209,#7208,#4267,.T.);
#8950=EDGE_CURVE('',#7206,#7209,#4268,.T.);
#8951=EDGE_CURVE('',#7208,#7210,#4269,.T.);
#8952=EDGE_CURVE('',#7211,#7210,#4270,.T.);
#8953=EDGE_CURVE('',#7209,#7211,#4271,.T.);
#8954=EDGE_CURVE('',#7210,#7204,#4272,.T.);
#8955=EDGE_CURVE('',#7211,#7207,#4273,.T.);
#8956=EDGE_CURVE('',#7212,#7212,#969,.T.);
#8957=EDGE_CURVE('',#7212,#7213,#4274,.T.);
#8958=EDGE_CURVE('',#7213,#7213,#970,.T.);
#8959=EDGE_CURVE('',#7214,#7215,#4275,.T.);
#8960=EDGE_CURVE('',#7215,#7216,#4276,.T.);
#8961=EDGE_CURVE('',#7216,#7217,#4277,.T.);
#8962=EDGE_CURVE('',#7217,#7218,#4278,.T.);
#8963=EDGE_CURVE('',#7218,#7219,#971,.T.);
#8964=EDGE_CURVE('',#7219,#7214,#4279,.T.);
#8965=EDGE_CURVE('',#7220,#7221,#4280,.T.);
#8966=EDGE_CURVE('',#7222,#7220,#4281,.T.);
#8967=EDGE_CURVE('',#7223,#7222,#972,.T.);
#8968=EDGE_CURVE('',#7224,#7223,#4282,.T.);
#8969=EDGE_CURVE('',#7225,#7224,#4283,.T.);
#8970=EDGE_CURVE('',#7221,#7225,#4284,.T.);
#8971=EDGE_CURVE('',#7215,#7221,#4285,.T.);
#8972=EDGE_CURVE('',#7214,#7220,#4286,.T.);
#8973=EDGE_CURVE('',#7216,#7225,#4287,.T.);
#8974=EDGE_CURVE('',#7217,#7224,#4288,.T.);
#8975=EDGE_CURVE('',#7218,#7223,#4289,.T.);
#8976=EDGE_CURVE('',#7219,#7222,#4290,.T.);
#8977=EDGE_CURVE('',#7226,#7226,#973,.T.);
#8978=EDGE_CURVE('',#7226,#7227,#4291,.T.);
#8979=EDGE_CURVE('',#7227,#7227,#974,.T.);
#8980=EDGE_CURVE('',#7228,#7229,#4292,.T.);
#8981=EDGE_CURVE('',#7230,#7228,#4293,.T.);
#8982=EDGE_CURVE('',#7231,#7230,#975,.T.);
#8983=EDGE_CURVE('',#7232,#7231,#4294,.T.);
#8984=EDGE_CURVE('',#7233,#7232,#4295,.T.);
#8985=EDGE_CURVE('',#7229,#7233,#4296,.T.);
#8986=EDGE_CURVE('',#7234,#7235,#4297,.T.);
#8987=EDGE_CURVE('',#7235,#7236,#4298,.T.);
#8988=EDGE_CURVE('',#7236,#7237,#4299,.T.);
#8989=EDGE_CURVE('',#7237,#7238,#4300,.T.);
#8990=EDGE_CURVE('',#7238,#7239,#976,.T.);
#8991=EDGE_CURVE('',#7239,#7234,#4301,.T.);
#8992=EDGE_CURVE('',#7228,#7234,#4302,.T.);
#8993=EDGE_CURVE('',#7229,#7235,#4303,.T.);
#8994=EDGE_CURVE('',#7233,#7236,#4304,.T.);
#8995=EDGE_CURVE('',#7232,#7237,#4305,.T.);
#8996=EDGE_CURVE('',#7231,#7238,#4306,.T.);
#8997=EDGE_CURVE('',#7230,#7239,#4307,.T.);
#8998=EDGE_CURVE('',#7240,#7240,#977,.T.);
#8999=EDGE_CURVE('',#7240,#7241,#4308,.T.);
#9000=EDGE_CURVE('',#7241,#7241,#978,.T.);
#9001=EDGE_CURVE('',#7242,#7242,#979,.T.);
#9002=EDGE_CURVE('',#7242,#7243,#4309,.T.);
#9003=EDGE_CURVE('',#7243,#7243,#980,.T.);
#9004=EDGE_CURVE('',#7244,#7244,#981,.T.);
#9005=EDGE_CURVE('',#7244,#7245,#4310,.T.);
#9006=EDGE_CURVE('',#7245,#7245,#982,.T.);
#9007=EDGE_CURVE('',#7246,#7246,#983,.T.);
#9008=EDGE_CURVE('',#7246,#7247,#4311,.T.);
#9009=EDGE_CURVE('',#7247,#7247,#984,.T.);
#9010=EDGE_CURVE('',#7248,#7248,#985,.T.);
#9011=EDGE_CURVE('',#7248,#7249,#4312,.T.);
#9012=EDGE_CURVE('',#7249,#7249,#986,.T.);
#9013=EDGE_CURVE('',#7250,#7251,#4313,.T.);
#9014=EDGE_CURVE('',#7251,#7252,#4314,.T.);
#9015=EDGE_CURVE('',#7252,#7253,#4315,.T.);
#9016=EDGE_CURVE('',#7253,#7254,#4316,.T.);
#9017=EDGE_CURVE('',#7254,#7255,#4317,.T.);
#9018=EDGE_CURVE('',#7255,#7256,#4318,.T.);
#9019=EDGE_CURVE('',#7256,#7257,#4319,.T.);
#9020=EDGE_CURVE('',#7257,#7250,#4320,.T.);
#9021=EDGE_CURVE('',#7258,#7259,#4321,.T.);
#9022=EDGE_CURVE('',#7260,#7258,#4322,.T.);
#9023=EDGE_CURVE('',#7261,#7260,#4323,.T.);
#9024=EDGE_CURVE('',#7262,#7261,#4324,.T.);
#9025=EDGE_CURVE('',#7263,#7262,#4325,.T.);
#9026=EDGE_CURVE('',#7264,#7263,#4326,.T.);
#9027=EDGE_CURVE('',#7265,#7264,#4327,.T.);
#9028=EDGE_CURVE('',#7259,#7265,#4328,.T.);
#9029=EDGE_CURVE('',#7251,#7259,#4329,.T.);
#9030=EDGE_CURVE('',#7250,#7258,#4330,.T.);
#9031=EDGE_CURVE('',#7252,#7265,#4331,.T.);
#9032=EDGE_CURVE('',#7253,#7264,#4332,.T.);
#9033=EDGE_CURVE('',#7254,#7263,#4333,.T.);
#9034=EDGE_CURVE('',#7255,#7262,#4334,.T.);
#9035=EDGE_CURVE('',#7256,#7261,#4335,.T.);
#9036=EDGE_CURVE('',#7257,#7260,#4336,.T.);
#9037=EDGE_CURVE('',#7266,#7267,#4337,.T.);
#9038=EDGE_CURVE('',#7268,#7267,#4338,.T.);
#9039=EDGE_CURVE('',#7269,#7268,#4339,.T.);
#9040=EDGE_CURVE('',#7269,#7266,#4340,.T.);
#9041=EDGE_CURVE('',#7267,#7270,#4341,.T.);
#9042=EDGE_CURVE('',#7271,#7270,#4342,.T.);
#9043=EDGE_CURVE('',#7268,#7271,#4343,.T.);
#9044=EDGE_CURVE('',#7270,#7272,#4344,.T.);
#9045=EDGE_CURVE('',#7273,#7272,#4345,.T.);
#9046=EDGE_CURVE('',#7271,#7273,#4346,.T.);
#9047=EDGE_CURVE('',#7272,#7266,#4347,.T.);
#9048=EDGE_CURVE('',#7273,#7269,#4348,.T.);
#9049=EDGE_CURVE('',#7274,#7275,#4349,.T.);
#9050=EDGE_CURVE('',#7276,#7275,#4350,.T.);
#9051=EDGE_CURVE('',#7277,#7276,#4351,.T.);
#9052=EDGE_CURVE('',#7277,#7274,#4352,.T.);
#9053=EDGE_CURVE('',#7275,#7278,#4353,.T.);
#9054=EDGE_CURVE('',#7279,#7278,#4354,.T.);
#9055=EDGE_CURVE('',#7276,#7279,#4355,.T.);
#9056=EDGE_CURVE('',#7278,#7280,#4356,.T.);
#9057=EDGE_CURVE('',#7281,#7280,#4357,.T.);
#9058=EDGE_CURVE('',#7279,#7281,#4358,.T.);
#9059=EDGE_CURVE('',#7280,#7274,#4359,.T.);
#9060=EDGE_CURVE('',#7281,#7277,#4360,.T.);
#9061=EDGE_CURVE('',#7282,#7283,#4361,.T.);
#9062=EDGE_CURVE('',#7284,#7283,#4362,.T.);
#9063=EDGE_CURVE('',#7285,#7284,#4363,.T.);
#9064=EDGE_CURVE('',#7285,#7282,#4364,.T.);
#9065=EDGE_CURVE('',#7283,#7286,#4365,.T.);
#9066=EDGE_CURVE('',#7287,#7286,#4366,.T.);
#9067=EDGE_CURVE('',#7284,#7287,#4367,.T.);
#9068=EDGE_CURVE('',#7286,#7288,#4368,.T.);
#9069=EDGE_CURVE('',#7289,#7288,#4369,.T.);
#9070=EDGE_CURVE('',#7287,#7289,#4370,.T.);
#9071=EDGE_CURVE('',#7288,#7290,#4371,.T.);
#9072=EDGE_CURVE('',#7291,#7290,#4372,.T.);
#9073=EDGE_CURVE('',#7289,#7291,#4373,.T.);
#9074=EDGE_CURVE('',#7290,#7292,#4374,.T.);
#9075=EDGE_CURVE('',#7293,#7292,#4375,.T.);
#9076=EDGE_CURVE('',#7291,#7293,#4376,.T.);
#9077=EDGE_CURVE('',#7292,#7282,#4377,.T.);
#9078=EDGE_CURVE('',#7293,#7285,#4378,.T.);
#9079=EDGE_CURVE('',#7294,#7294,#987,.T.);
#9080=EDGE_CURVE('',#7294,#7295,#4379,.T.);
#9081=EDGE_CURVE('',#7295,#7295,#988,.T.);
#9082=EDGE_CURVE('',#7296,#7296,#989,.T.);
#9083=EDGE_CURVE('',#7296,#7297,#4380,.T.);
#9084=EDGE_CURVE('',#7297,#7297,#990,.T.);
#9085=EDGE_CURVE('',#7298,#7298,#991,.T.);
#9086=EDGE_CURVE('',#7298,#7299,#4381,.T.);
#9087=EDGE_CURVE('',#7299,#7299,#992,.T.);
#9088=EDGE_CURVE('',#7300,#7301,#4382,.T.);
#9089=EDGE_CURVE('',#7301,#7302,#4383,.T.);
#9090=EDGE_CURVE('',#7302,#7303,#4384,.T.);
#9091=EDGE_CURVE('',#7303,#7300,#4385,.T.);
#9092=EDGE_CURVE('',#7304,#7305,#4386,.T.);
#9093=EDGE_CURVE('',#7306,#7304,#4387,.T.);
#9094=EDGE_CURVE('',#7307,#7306,#4388,.T.);
#9095=EDGE_CURVE('',#7305,#7307,#4389,.T.);
#9096=EDGE_CURVE('',#7301,#7305,#4390,.T.);
#9097=EDGE_CURVE('',#7300,#7304,#4391,.T.);
#9098=EDGE_CURVE('',#7302,#7307,#4392,.T.);
#9099=EDGE_CURVE('',#7303,#7306,#4393,.T.);
#9100=EDGE_CURVE('',#7308,#7308,#993,.T.);
#9101=EDGE_CURVE('',#7308,#7309,#4394,.T.);
#9102=EDGE_CURVE('',#7309,#7309,#994,.T.);
#9103=EDGE_CURVE('',#7310,#7310,#995,.T.);
#9104=EDGE_CURVE('',#7310,#7311,#4395,.T.);
#9105=EDGE_CURVE('',#7311,#7311,#996,.T.);
#9106=EDGE_CURVE('',#7312,#7312,#997,.T.);
#9107=EDGE_CURVE('',#7312,#7313,#4396,.T.);
#9108=EDGE_CURVE('',#7313,#7313,#998,.T.);
#9109=EDGE_CURVE('',#7314,#7315,#4397,.T.);
#9110=EDGE_CURVE('',#7315,#7316,#4398,.T.);
#9111=EDGE_CURVE('',#7316,#7317,#4399,.T.);
#9112=EDGE_CURVE('',#7317,#7314,#4400,.T.);
#9113=EDGE_CURVE('',#7318,#7319,#4401,.T.);
#9114=EDGE_CURVE('',#7320,#7318,#4402,.T.);
#9115=EDGE_CURVE('',#7321,#7320,#4403,.T.);
#9116=EDGE_CURVE('',#7319,#7321,#4404,.T.);
#9117=EDGE_CURVE('',#7315,#7319,#4405,.T.);
#9118=EDGE_CURVE('',#7314,#7318,#4406,.T.);
#9119=EDGE_CURVE('',#7316,#7321,#4407,.T.);
#9120=EDGE_CURVE('',#7317,#7320,#4408,.T.);
#9121=EDGE_CURVE('',#7322,#7322,#999,.T.);
#9122=EDGE_CURVE('',#7322,#7323,#4409,.T.);
#9123=EDGE_CURVE('',#7323,#7323,#1000,.T.);
#9124=EDGE_CURVE('',#7324,#7324,#1001,.T.);
#9125=EDGE_CURVE('',#7324,#7325,#4410,.T.);
#9126=EDGE_CURVE('',#7325,#7325,#1002,.T.);
#9127=EDGE_CURVE('',#7326,#7326,#1003,.T.);
#9128=EDGE_CURVE('',#7326,#7327,#4411,.T.);
#9129=EDGE_CURVE('',#7327,#7327,#1004,.T.);
#9130=EDGE_CURVE('',#7328,#7329,#4412,.T.);
#9131=EDGE_CURVE('',#7329,#7330,#4413,.T.);
#9132=EDGE_CURVE('',#7330,#7331,#4414,.T.);
#9133=EDGE_CURVE('',#7331,#7328,#4415,.T.);
#9134=EDGE_CURVE('',#7332,#7333,#4416,.T.);
#9135=EDGE_CURVE('',#7334,#7332,#4417,.T.);
#9136=EDGE_CURVE('',#7335,#7334,#4418,.T.);
#9137=EDGE_CURVE('',#7333,#7335,#4419,.T.);
#9138=EDGE_CURVE('',#7329,#7333,#4420,.T.);
#9139=EDGE_CURVE('',#7328,#7332,#4421,.T.);
#9140=EDGE_CURVE('',#7330,#7335,#4422,.T.);
#9141=EDGE_CURVE('',#7331,#7334,#4423,.T.);
#9142=EDGE_CURVE('',#7336,#7336,#1005,.T.);
#9143=EDGE_CURVE('',#7336,#7337,#4424,.T.);
#9144=EDGE_CURVE('',#7337,#7337,#1006,.T.);
#9145=EDGE_CURVE('',#7338,#7338,#1007,.T.);
#9146=EDGE_CURVE('',#7338,#7339,#4425,.T.);
#9147=EDGE_CURVE('',#7339,#7339,#1008,.T.);
#9148=EDGE_CURVE('',#7340,#7340,#1009,.T.);
#9149=EDGE_CURVE('',#7340,#7341,#4426,.T.);
#9150=EDGE_CURVE('',#7341,#7341,#1010,.T.);
#9151=EDGE_CURVE('',#7342,#7343,#4427,.T.);
#9152=EDGE_CURVE('',#7343,#7344,#4428,.T.);
#9153=EDGE_CURVE('',#7344,#7345,#4429,.T.);
#9154=EDGE_CURVE('',#7345,#7342,#4430,.T.);
#9155=EDGE_CURVE('',#7346,#7347,#4431,.T.);
#9156=EDGE_CURVE('',#7348,#7346,#4432,.T.);
#9157=EDGE_CURVE('',#7349,#7348,#4433,.T.);
#9158=EDGE_CURVE('',#7347,#7349,#4434,.T.);
#9159=EDGE_CURVE('',#7343,#7347,#4435,.T.);
#9160=EDGE_CURVE('',#7342,#7346,#4436,.T.);
#9161=EDGE_CURVE('',#7344,#7349,#4437,.T.);
#9162=EDGE_CURVE('',#7345,#7348,#4438,.T.);
#9163=EDGE_CURVE('',#7350,#7351,#4439,.T.);
#9164=EDGE_CURVE('',#7352,#7350,#4440,.T.);
#9165=EDGE_CURVE('',#7352,#7353,#4441,.T.);
#9166=EDGE_CURVE('',#7353,#7351,#4442,.T.);
#9167=EDGE_CURVE('',#7351,#7354,#4443,.T.);
#9168=EDGE_CURVE('',#7353,#7355,#4444,.T.);
#9169=EDGE_CURVE('',#7355,#7354,#4445,.T.);
#9170=EDGE_CURVE('',#7354,#7356,#4446,.T.);
#9171=EDGE_CURVE('',#7355,#7357,#4447,.T.);
#9172=EDGE_CURVE('',#7357,#7356,#4448,.T.);
#9173=EDGE_CURVE('',#7356,#7350,#4449,.T.);
#9174=EDGE_CURVE('',#7357,#7352,#4450,.T.);
#9175=EDGE_CURVE('',#7358,#7359,#4451,.T.);
#9176=EDGE_CURVE('',#7360,#7358,#4452,.T.);
#9177=EDGE_CURVE('',#7360,#7361,#4453,.T.);
#9178=EDGE_CURVE('',#7361,#7359,#4454,.T.);
#9179=EDGE_CURVE('',#7359,#7362,#4455,.T.);
#9180=EDGE_CURVE('',#7361,#7363,#4456,.T.);
#9181=EDGE_CURVE('',#7363,#7362,#4457,.T.);
#9182=EDGE_CURVE('',#7362,#7364,#4458,.T.);
#9183=EDGE_CURVE('',#7363,#7365,#4459,.T.);
#9184=EDGE_CURVE('',#7365,#7364,#4460,.T.);
#9185=EDGE_CURVE('',#7364,#7358,#4461,.T.);
#9186=EDGE_CURVE('',#7365,#7360,#4462,.T.);
#9187=EDGE_CURVE('',#7366,#7367,#4463,.T.);
#9188=EDGE_CURVE('',#7368,#7366,#4464,.T.);
#9189=EDGE_CURVE('',#7368,#7369,#4465,.T.);
#9190=EDGE_CURVE('',#7369,#7367,#4466,.T.);
#9191=EDGE_CURVE('',#7370,#7366,#4467,.T.);
#9192=EDGE_CURVE('',#7371,#7370,#4468,.T.);
#9193=EDGE_CURVE('',#7371,#7368,#4469,.T.);
#9194=EDGE_CURVE('',#7372,#7370,#4470,.T.);
#9195=EDGE_CURVE('',#7373,#7372,#4471,.T.);
#9196=EDGE_CURVE('',#7373,#7371,#4472,.T.);
#9197=EDGE_CURVE('',#7367,#7372,#4473,.T.);
#9198=EDGE_CURVE('',#7369,#7373,#4474,.T.);
#9199=EDGE_CURVE('',#7374,#7375,#4475,.T.);
#9200=EDGE_CURVE('',#7376,#7374,#4476,.T.);
#9201=EDGE_CURVE('',#7376,#7377,#4477,.T.);
#9202=EDGE_CURVE('',#7377,#7375,#4478,.T.);
#9203=EDGE_CURVE('',#7378,#7374,#4479,.T.);
#9204=EDGE_CURVE('',#7379,#7378,#4480,.T.);
#9205=EDGE_CURVE('',#7379,#7376,#4481,.T.);
#9206=EDGE_CURVE('',#7380,#7378,#4482,.T.);
#9207=EDGE_CURVE('',#7381,#7380,#4483,.T.);
#9208=EDGE_CURVE('',#7381,#7379,#4484,.T.);
#9209=EDGE_CURVE('',#7375,#7380,#4485,.T.);
#9210=EDGE_CURVE('',#7377,#7381,#4486,.T.);
#9211=EDGE_CURVE('',#7382,#7383,#4487,.T.);
#9212=EDGE_CURVE('',#7384,#7383,#4488,.T.);
#9213=EDGE_CURVE('',#7385,#7384,#4489,.T.);
#9214=EDGE_CURVE('',#7385,#7382,#4490,.T.);
#9215=EDGE_CURVE('',#7386,#7382,#4491,.T.);
#9216=EDGE_CURVE('',#7387,#7385,#4492,.T.);
#9217=EDGE_CURVE('',#7387,#7386,#4493,.T.);
#9218=EDGE_CURVE('',#7388,#7386,#4494,.T.);
#9219=EDGE_CURVE('',#7389,#7387,#4495,.T.);
#9220=EDGE_CURVE('',#7389,#7388,#4496,.T.);
#9221=EDGE_CURVE('',#7383,#7388,#4497,.T.);
#9222=EDGE_CURVE('',#7384,#7389,#4498,.T.);
#9223=EDGE_CURVE('',#7390,#7390,#1011,.T.);
#9224=EDGE_CURVE('',#7390,#7391,#4499,.T.);
#9225=EDGE_CURVE('',#7391,#7391,#1012,.T.);
#9226=EDGE_CURVE('',#7392,#7392,#1013,.T.);
#9227=EDGE_CURVE('',#7392,#7393,#4500,.T.);
#9228=EDGE_CURVE('',#7393,#7393,#1014,.T.);
#9229=EDGE_CURVE('',#7394,#7394,#1015,.T.);
#9230=EDGE_CURVE('',#7394,#7395,#4501,.T.);
#9231=EDGE_CURVE('',#7395,#7395,#1016,.T.);
#9232=EDGE_CURVE('',#7396,#7396,#1017,.T.);
#9233=EDGE_CURVE('',#7396,#7397,#4502,.T.);
#9234=EDGE_CURVE('',#7397,#7397,#1018,.T.);
#9235=EDGE_CURVE('',#7398,#7399,#4503,.T.);
#9236=EDGE_CURVE('',#7399,#7400,#4504,.T.);
#9237=EDGE_CURVE('',#7400,#7401,#4505,.T.);
#9238=EDGE_CURVE('',#7401,#7398,#4506,.T.);
#9239=EDGE_CURVE('',#7402,#7403,#4507,.T.);
#9240=EDGE_CURVE('',#7404,#7402,#4508,.T.);
#9241=EDGE_CURVE('',#7405,#7404,#4509,.T.);
#9242=EDGE_CURVE('',#7403,#7405,#4510,.T.);
#9243=EDGE_CURVE('',#7399,#7403,#4511,.T.);
#9244=EDGE_CURVE('',#7398,#7402,#4512,.T.);
#9245=EDGE_CURVE('',#7400,#7405,#4513,.T.);
#9246=EDGE_CURVE('',#7401,#7404,#4514,.T.);
#9247=EDGE_CURVE('',#7406,#7406,#1019,.T.);
#9248=EDGE_CURVE('',#7406,#7407,#4515,.T.);
#9249=EDGE_CURVE('',#7407,#7407,#1020,.T.);
#9250=EDGE_CURVE('',#7408,#7408,#1021,.T.);
#9251=EDGE_CURVE('',#7408,#7409,#4516,.T.);
#9252=EDGE_CURVE('',#7409,#7409,#1022,.T.);
#9253=EDGE_CURVE('',#7410,#7410,#1023,.T.);
#9254=EDGE_CURVE('',#7410,#7411,#4517,.T.);
#9255=EDGE_CURVE('',#7411,#7411,#1024,.T.);
#9256=EDGE_CURVE('',#7412,#7412,#1025,.T.);
#9257=EDGE_CURVE('',#7412,#7413,#4518,.T.);
#9258=EDGE_CURVE('',#7413,#7413,#1026,.T.);
#9259=EDGE_CURVE('',#7414,#7414,#1027,.T.);
#9260=EDGE_CURVE('',#7414,#7415,#4519,.T.);
#9261=EDGE_CURVE('',#7415,#7415,#1028,.T.);
#9262=EDGE_CURVE('',#7416,#7416,#1029,.T.);
#9263=EDGE_CURVE('',#7416,#7417,#4520,.T.);
#9264=EDGE_CURVE('',#7417,#7417,#1030,.T.);
#9265=EDGE_CURVE('',#7418,#7419,#4521,.T.);
#9266=EDGE_CURVE('',#7420,#7418,#4522,.T.);
#9267=EDGE_CURVE('',#7420,#7421,#4523,.T.);
#9268=EDGE_CURVE('',#7421,#7419,#4524,.T.);
#9269=EDGE_CURVE('',#7422,#7418,#4525,.T.);
#9270=EDGE_CURVE('',#7423,#7422,#4526,.T.);
#9271=EDGE_CURVE('',#7423,#7420,#4527,.T.);
#9272=EDGE_CURVE('',#7424,#7422,#4528,.T.);
#9273=EDGE_CURVE('',#7425,#7424,#4529,.T.);
#9274=EDGE_CURVE('',#7425,#7423,#4530,.T.);
#9275=EDGE_CURVE('',#7419,#7424,#4531,.T.);
#9276=EDGE_CURVE('',#7421,#7425,#4532,.T.);
#9277=EDGE_CURVE('',#7426,#7427,#4533,.T.);
#9278=EDGE_CURVE('',#7428,#7427,#4534,.T.);
#9279=EDGE_CURVE('',#7429,#7428,#4535,.T.);
#9280=EDGE_CURVE('',#7429,#7426,#4536,.T.);
#9281=EDGE_CURVE('',#7427,#7430,#4537,.T.);
#9282=EDGE_CURVE('',#7431,#7430,#4538,.T.);
#9283=EDGE_CURVE('',#7428,#7431,#4539,.T.);
#9284=EDGE_CURVE('',#7430,#7432,#4540,.T.);
#9285=EDGE_CURVE('',#7433,#7432,#4541,.T.);
#9286=EDGE_CURVE('',#7431,#7433,#4542,.T.);
#9287=EDGE_CURVE('',#7432,#7434,#4543,.T.);
#9288=EDGE_CURVE('',#7435,#7434,#4544,.T.);
#9289=EDGE_CURVE('',#7433,#7435,#4545,.T.);
#9290=EDGE_CURVE('',#7434,#7436,#4546,.T.);
#9291=EDGE_CURVE('',#7437,#7436,#4547,.T.);
#9292=EDGE_CURVE('',#7435,#7437,#4548,.T.);
#9293=EDGE_CURVE('',#7436,#7438,#4549,.T.);
#9294=EDGE_CURVE('',#7439,#7438,#4550,.T.);
#9295=EDGE_CURVE('',#7437,#7439,#4551,.T.);
#9296=EDGE_CURVE('',#7438,#7426,#4552,.T.);
#9297=EDGE_CURVE('',#7439,#7429,#4553,.T.);
#9298=EDGE_CURVE('',#7440,#7441,#4554,.T.);
#9299=EDGE_CURVE('',#7442,#7441,#4555,.T.);
#9300=EDGE_CURVE('',#7443,#7442,#4556,.T.);
#9301=EDGE_CURVE('',#7443,#7440,#4557,.T.);
#9302=EDGE_CURVE('',#7441,#7444,#4558,.T.);
#9303=EDGE_CURVE('',#7445,#7444,#4559,.T.);
#9304=EDGE_CURVE('',#7442,#7445,#4560,.T.);
#9305=EDGE_CURVE('',#7444,#7446,#4561,.T.);
#9306=EDGE_CURVE('',#7447,#7446,#4562,.T.);
#9307=EDGE_CURVE('',#7445,#7447,#4563,.T.);
#9308=EDGE_CURVE('',#7446,#7448,#4564,.T.);
#9309=EDGE_CURVE('',#7449,#7448,#4565,.T.);
#9310=EDGE_CURVE('',#7447,#7449,#4566,.T.);
#9311=EDGE_CURVE('',#7448,#7450,#4567,.T.);
#9312=EDGE_CURVE('',#7451,#7450,#4568,.T.);
#9313=EDGE_CURVE('',#7449,#7451,#4569,.T.);
#9314=EDGE_CURVE('',#7450,#7452,#4570,.T.);
#9315=EDGE_CURVE('',#7453,#7452,#4571,.T.);
#9316=EDGE_CURVE('',#7451,#7453,#4572,.T.);
#9317=EDGE_CURVE('',#7452,#7440,#4573,.T.);
#9318=EDGE_CURVE('',#7453,#7443,#4574,.T.);
#9319=EDGE_CURVE('',#7454,#7455,#4575,.T.);
#9320=EDGE_CURVE('',#7456,#7455,#4576,.T.);
#9321=EDGE_CURVE('',#7457,#7456,#4577,.T.);
#9322=EDGE_CURVE('',#7457,#7454,#4578,.T.);
#9323=EDGE_CURVE('',#7455,#7458,#4579,.T.);
#9324=EDGE_CURVE('',#7459,#7458,#4580,.T.);
#9325=EDGE_CURVE('',#7456,#7459,#4581,.T.);
#9326=EDGE_CURVE('',#7458,#7460,#4582,.T.);
#9327=EDGE_CURVE('',#7461,#7460,#4583,.T.);
#9328=EDGE_CURVE('',#7459,#7461,#4584,.T.);
#9329=EDGE_CURVE('',#7460,#7462,#4585,.T.);
#9330=EDGE_CURVE('',#7463,#7462,#4586,.T.);
#9331=EDGE_CURVE('',#7461,#7463,#4587,.T.);
#9332=EDGE_CURVE('',#7462,#7464,#4588,.T.);
#9333=EDGE_CURVE('',#7465,#7464,#4589,.T.);
#9334=EDGE_CURVE('',#7463,#7465,#4590,.T.);
#9335=EDGE_CURVE('',#7464,#7466,#4591,.T.);
#9336=EDGE_CURVE('',#7467,#7466,#4592,.T.);
#9337=EDGE_CURVE('',#7465,#7467,#4593,.T.);
#9338=EDGE_CURVE('',#7466,#7454,#4594,.T.);
#9339=EDGE_CURVE('',#7467,#7457,#4595,.T.);
#9340=EDGE_CURVE('',#7468,#7469,#4596,.T.);
#9341=EDGE_CURVE('',#7470,#7468,#4597,.T.);
#9342=EDGE_CURVE('',#7470,#7471,#4598,.T.);
#9343=EDGE_CURVE('',#7471,#7469,#4599,.T.);
#9344=EDGE_CURVE('',#7472,#7468,#4600,.T.);
#9345=EDGE_CURVE('',#7473,#7472,#4601,.T.);
#9346=EDGE_CURVE('',#7473,#7470,#4602,.T.);
#9347=EDGE_CURVE('',#7474,#7472,#4603,.T.);
#9348=EDGE_CURVE('',#7475,#7474,#4604,.T.);
#9349=EDGE_CURVE('',#7475,#7473,#4605,.T.);
#9350=EDGE_CURVE('',#7476,#7474,#4606,.T.);
#9351=EDGE_CURVE('',#7477,#7476,#4607,.T.);
#9352=EDGE_CURVE('',#7477,#7475,#4608,.T.);
#9353=EDGE_CURVE('',#7478,#7476,#4609,.T.);
#9354=EDGE_CURVE('',#7479,#7478,#4610,.T.);
#9355=EDGE_CURVE('',#7479,#7477,#4611,.T.);
#9356=EDGE_CURVE('',#7480,#7478,#4612,.T.);
#9357=EDGE_CURVE('',#7481,#7480,#4613,.T.);
#9358=EDGE_CURVE('',#7481,#7479,#4614,.T.);
#9359=EDGE_CURVE('',#7469,#7480,#4615,.T.);
#9360=EDGE_CURVE('',#7471,#7481,#4616,.T.);
#9361=EDGE_CURVE('',#7482,#7483,#4617,.T.);
#9362=EDGE_CURVE('',#7484,#7482,#4618,.T.);
#9363=EDGE_CURVE('',#7484,#7485,#4619,.T.);
#9364=EDGE_CURVE('',#7485,#7483,#4620,.T.);
#9365=EDGE_CURVE('',#7486,#7482,#4621,.T.);
#9366=EDGE_CURVE('',#7487,#7486,#4622,.T.);
#9367=EDGE_CURVE('',#7487,#7484,#4623,.T.);
#9368=EDGE_CURVE('',#7488,#7486,#4624,.T.);
#9369=EDGE_CURVE('',#7489,#7488,#4625,.T.);
#9370=EDGE_CURVE('',#7489,#7487,#4626,.T.);
#9371=EDGE_CURVE('',#7490,#7488,#4627,.T.);
#9372=EDGE_CURVE('',#7491,#7490,#4628,.T.);
#9373=EDGE_CURVE('',#7491,#7489,#4629,.T.);
#9374=EDGE_CURVE('',#7492,#7490,#4630,.T.);
#9375=EDGE_CURVE('',#7493,#7492,#4631,.T.);
#9376=EDGE_CURVE('',#7493,#7491,#4632,.T.);
#9377=EDGE_CURVE('',#7494,#7492,#4633,.T.);
#9378=EDGE_CURVE('',#7495,#7494,#4634,.T.);
#9379=EDGE_CURVE('',#7495,#7493,#4635,.T.);
#9380=EDGE_CURVE('',#7483,#7494,#4636,.T.);
#9381=EDGE_CURVE('',#7485,#7495,#4637,.T.);
#9382=EDGE_CURVE('',#7496,#7497,#4638,.T.);
#9383=EDGE_CURVE('',#7498,#7496,#4639,.T.);
#9384=EDGE_CURVE('',#7498,#7499,#4640,.T.);
#9385=EDGE_CURVE('',#7499,#7497,#4641,.T.);
#9386=EDGE_CURVE('',#7500,#7496,#4642,.T.);
#9387=EDGE_CURVE('',#7501,#7500,#4643,.T.);
#9388=EDGE_CURVE('',#7501,#7498,#4644,.T.);
#9389=EDGE_CURVE('',#7502,#7500,#4645,.T.);
#9390=EDGE_CURVE('',#7503,#7502,#4646,.T.);
#9391=EDGE_CURVE('',#7503,#7501,#4647,.T.);
#9392=EDGE_CURVE('',#7504,#7502,#4648,.T.);
#9393=EDGE_CURVE('',#7505,#7504,#4649,.T.);
#9394=EDGE_CURVE('',#7505,#7503,#4650,.T.);
#9395=EDGE_CURVE('',#7506,#7504,#4651,.T.);
#9396=EDGE_CURVE('',#7507,#7506,#4652,.T.);
#9397=EDGE_CURVE('',#7507,#7505,#4653,.T.);
#9398=EDGE_CURVE('',#7508,#7506,#4654,.T.);
#9399=EDGE_CURVE('',#7509,#7508,#4655,.T.);
#9400=EDGE_CURVE('',#7509,#7507,#4656,.T.);
#9401=EDGE_CURVE('',#7497,#7508,#4657,.T.);
#9402=EDGE_CURVE('',#7499,#7509,#4658,.T.);
#9403=EDGE_CURVE('',#7510,#7511,#4659,.T.);
#9404=EDGE_CURVE('',#7512,#7511,#4660,.T.);
#9405=EDGE_CURVE('',#7513,#7512,#4661,.T.);
#9406=EDGE_CURVE('',#7513,#7510,#4662,.T.);
#9407=EDGE_CURVE('',#7514,#7510,#4663,.T.);
#9408=EDGE_CURVE('',#7515,#7513,#4664,.T.);
#9409=EDGE_CURVE('',#7515,#7514,#4665,.T.);
#9410=EDGE_CURVE('',#7516,#7514,#4666,.T.);
#9411=EDGE_CURVE('',#7517,#7515,#4667,.T.);
#9412=EDGE_CURVE('',#7517,#7516,#4668,.T.);
#9413=EDGE_CURVE('',#7518,#7516,#4669,.T.);
#9414=EDGE_CURVE('',#7519,#7517,#4670,.T.);
#9415=EDGE_CURVE('',#7519,#7518,#4671,.T.);
#9416=EDGE_CURVE('',#7520,#7518,#4672,.T.);
#9417=EDGE_CURVE('',#7521,#7519,#4673,.T.);
#9418=EDGE_CURVE('',#7521,#7520,#4674,.T.);
#9419=EDGE_CURVE('',#7522,#7520,#4675,.T.);
#9420=EDGE_CURVE('',#7523,#7521,#4676,.T.);
#9421=EDGE_CURVE('',#7523,#7522,#4677,.T.);
#9422=EDGE_CURVE('',#7511,#7522,#4678,.T.);
#9423=EDGE_CURVE('',#7512,#7523,#4679,.T.);
#9424=EDGE_CURVE('',#7524,#7525,#4680,.T.);
#9425=EDGE_CURVE('',#7526,#7525,#4681,.T.);
#9426=EDGE_CURVE('',#7527,#7526,#4682,.T.);
#9427=EDGE_CURVE('',#7527,#7524,#4683,.T.);
#9428=EDGE_CURVE('',#7528,#7524,#4684,.T.);
#9429=EDGE_CURVE('',#7529,#7527,#4685,.T.);
#9430=EDGE_CURVE('',#7529,#7528,#4686,.T.);
#9431=EDGE_CURVE('',#7530,#7528,#4687,.T.);
#9432=EDGE_CURVE('',#7531,#7529,#4688,.T.);
#9433=EDGE_CURVE('',#7531,#7530,#4689,.T.);
#9434=EDGE_CURVE('',#7532,#7530,#4690,.T.);
#9435=EDGE_CURVE('',#7533,#7531,#4691,.T.);
#9436=EDGE_CURVE('',#7533,#7532,#4692,.T.);
#9437=EDGE_CURVE('',#7534,#7532,#4693,.T.);
#9438=EDGE_CURVE('',#7535,#7533,#4694,.T.);
#9439=EDGE_CURVE('',#7535,#7534,#4695,.T.);
#9440=EDGE_CURVE('',#7536,#7534,#4696,.T.);
#9441=EDGE_CURVE('',#7537,#7535,#4697,.T.);
#9442=EDGE_CURVE('',#7537,#7536,#4698,.T.);
#9443=EDGE_CURVE('',#7525,#7536,#4699,.T.);
#9444=EDGE_CURVE('',#7526,#7537,#4700,.T.);
#9445=EDGE_CURVE('',#7538,#7539,#4701,.T.);
#9446=EDGE_CURVE('',#7540,#7538,#4702,.T.);
#9447=EDGE_CURVE('',#7540,#7541,#4703,.T.);
#9448=EDGE_CURVE('',#7541,#7539,#4704,.T.);
#9449=EDGE_CURVE('',#7539,#7542,#4705,.T.);
#9450=EDGE_CURVE('',#7541,#7543,#4706,.T.);
#9451=EDGE_CURVE('',#7543,#7542,#4707,.T.);
#9452=EDGE_CURVE('',#7542,#7544,#4708,.T.);
#9453=EDGE_CURVE('',#7543,#7545,#4709,.T.);
#9454=EDGE_CURVE('',#7545,#7544,#4710,.T.);
#9455=EDGE_CURVE('',#7544,#7546,#4711,.T.);
#9456=EDGE_CURVE('',#7545,#7547,#4712,.T.);
#9457=EDGE_CURVE('',#7547,#7546,#4713,.T.);
#9458=EDGE_CURVE('',#7546,#7548,#4714,.T.);
#9459=EDGE_CURVE('',#7547,#7549,#4715,.T.);
#9460=EDGE_CURVE('',#7549,#7548,#4716,.T.);
#9461=EDGE_CURVE('',#7548,#7550,#4717,.T.);
#9462=EDGE_CURVE('',#7549,#7551,#4718,.T.);
#9463=EDGE_CURVE('',#7551,#7550,#4719,.T.);
#9464=EDGE_CURVE('',#7550,#7538,#4720,.T.);
#9465=EDGE_CURVE('',#7551,#7540,#4721,.T.);
#9466=EDGE_CURVE('',#7552,#7553,#4722,.T.);
#9467=EDGE_CURVE('',#7554,#7552,#4723,.T.);
#9468=EDGE_CURVE('',#7554,#7555,#4724,.T.);
#9469=EDGE_CURVE('',#7555,#7553,#4725,.T.);
#9470=EDGE_CURVE('',#7553,#7556,#4726,.T.);
#9471=EDGE_CURVE('',#7555,#7557,#4727,.T.);
#9472=EDGE_CURVE('',#7557,#7556,#4728,.T.);
#9473=EDGE_CURVE('',#7556,#7558,#4729,.T.);
#9474=EDGE_CURVE('',#7557,#7559,#4730,.T.);
#9475=EDGE_CURVE('',#7559,#7558,#4731,.T.);
#9476=EDGE_CURVE('',#7558,#7560,#4732,.T.);
#9477=EDGE_CURVE('',#7559,#7561,#4733,.T.);
#9478=EDGE_CURVE('',#7561,#7560,#4734,.T.);
#9479=EDGE_CURVE('',#7560,#7562,#4735,.T.);
#9480=EDGE_CURVE('',#7561,#7563,#4736,.T.);
#9481=EDGE_CURVE('',#7563,#7562,#4737,.T.);
#9482=EDGE_CURVE('',#7562,#7564,#4738,.T.);
#9483=EDGE_CURVE('',#7563,#7565,#4739,.T.);
#9484=EDGE_CURVE('',#7565,#7564,#4740,.T.);
#9485=EDGE_CURVE('',#7564,#7552,#4741,.T.);
#9486=EDGE_CURVE('',#7565,#7554,#4742,.T.);
#9487=EDGE_CURVE('',#7566,#7567,#4743,.T.);
#9488=EDGE_CURVE('',#7568,#7566,#4744,.T.);
#9489=EDGE_CURVE('',#7568,#7569,#4745,.T.);
#9490=EDGE_CURVE('',#7569,#7567,#4746,.T.);
#9491=EDGE_CURVE('',#7567,#7570,#4747,.T.);
#9492=EDGE_CURVE('',#7569,#7571,#4748,.T.);
#9493=EDGE_CURVE('',#7571,#7570,#4749,.T.);
#9494=EDGE_CURVE('',#7570,#7572,#4750,.T.);
#9495=EDGE_CURVE('',#7571,#7573,#4751,.T.);
#9496=EDGE_CURVE('',#7573,#7572,#4752,.T.);
#9497=EDGE_CURVE('',#7572,#7574,#4753,.T.);
#9498=EDGE_CURVE('',#7573,#7575,#4754,.T.);
#9499=EDGE_CURVE('',#7575,#7574,#4755,.T.);
#9500=EDGE_CURVE('',#7574,#7576,#4756,.T.);
#9501=EDGE_CURVE('',#7575,#7577,#4757,.T.);
#9502=EDGE_CURVE('',#7577,#7576,#4758,.T.);
#9503=EDGE_CURVE('',#7576,#7578,#4759,.T.);
#9504=EDGE_CURVE('',#7577,#7579,#4760,.T.);
#9505=EDGE_CURVE('',#7579,#7578,#4761,.T.);
#9506=EDGE_CURVE('',#7578,#7566,#4762,.T.);
#9507=EDGE_CURVE('',#7579,#7568,#4763,.T.);
#9508=EDGE_CURVE('',#7580,#7580,#1031,.T.);
#9509=EDGE_CURVE('',#7580,#7581,#4764,.T.);
#9510=EDGE_CURVE('',#7581,#7581,#1032,.T.);
#9511=EDGE_CURVE('',#7582,#7582,#1033,.T.);
#9512=EDGE_CURVE('',#7582,#7583,#4765,.T.);
#9513=EDGE_CURVE('',#7583,#7583,#1034,.T.);
#9514=EDGE_CURVE('',#7584,#7584,#1035,.T.);
#9515=EDGE_CURVE('',#7584,#7585,#4766,.T.);
#9516=EDGE_CURVE('',#7585,#7585,#1036,.T.);
#9517=EDGE_CURVE('',#7586,#7586,#1037,.T.);
#9518=EDGE_CURVE('',#7586,#7587,#4767,.T.);
#9519=EDGE_CURVE('',#7587,#7587,#1038,.T.);
#9520=EDGE_CURVE('',#7588,#7589,#4768,.T.);
#9521=EDGE_CURVE('',#7590,#7588,#4769,.T.);
#9522=EDGE_CURVE('',#7591,#7590,#4770,.T.);
#9523=EDGE_CURVE('',#7589,#7591,#4771,.T.);
#9524=EDGE_CURVE('',#7592,#7593,#4772,.T.);
#9525=EDGE_CURVE('',#7593,#7594,#4773,.T.);
#9526=EDGE_CURVE('',#7594,#7595,#4774,.T.);
#9527=EDGE_CURVE('',#7595,#7592,#4775,.T.);
#9528=EDGE_CURVE('',#7588,#7592,#4776,.T.);
#9529=EDGE_CURVE('',#7589,#7593,#4777,.T.);
#9530=EDGE_CURVE('',#7591,#7594,#4778,.T.);
#9531=EDGE_CURVE('',#7590,#7595,#4779,.T.);
#9532=EDGE_CURVE('',#7596,#7597,#4780,.T.);
#9533=EDGE_CURVE('',#7598,#7597,#4781,.T.);
#9534=EDGE_CURVE('',#7599,#7598,#4782,.T.);
#9535=EDGE_CURVE('',#7599,#7596,#4783,.T.);
#9536=EDGE_CURVE('',#7597,#7600,#4784,.T.);
#9537=EDGE_CURVE('',#7601,#7600,#4785,.T.);
#9538=EDGE_CURVE('',#7598,#7601,#4786,.T.);
#9539=EDGE_CURVE('',#7600,#7602,#4787,.T.);
#9540=EDGE_CURVE('',#7603,#7602,#4788,.T.);
#9541=EDGE_CURVE('',#7601,#7603,#4789,.T.);
#9542=EDGE_CURVE('',#7602,#7596,#4790,.T.);
#9543=EDGE_CURVE('',#7603,#7599,#4791,.T.);
#9544=EDGE_CURVE('',#7604,#7605,#4792,.T.);
#9545=EDGE_CURVE('',#7606,#7605,#4793,.T.);
#9546=EDGE_CURVE('',#7607,#7606,#4794,.T.);
#9547=EDGE_CURVE('',#7607,#7604,#4795,.T.);
#9548=EDGE_CURVE('',#7605,#7608,#4796,.T.);
#9549=EDGE_CURVE('',#7609,#7608,#4797,.T.);
#9550=EDGE_CURVE('',#7606,#7609,#4798,.T.);
#9551=EDGE_CURVE('',#7608,#7610,#4799,.T.);
#9552=EDGE_CURVE('',#7611,#7610,#4800,.T.);
#9553=EDGE_CURVE('',#7609,#7611,#4801,.T.);
#9554=EDGE_CURVE('',#7610,#7604,#4802,.T.);
#9555=EDGE_CURVE('',#7611,#7607,#4803,.T.);
#9556=EDGE_CURVE('',#7612,#7613,#4804,.T.);
#9557=EDGE_CURVE('',#7614,#7613,#4805,.T.);
#9558=EDGE_CURVE('',#7615,#7614,#4806,.T.);
#9559=EDGE_CURVE('',#7615,#7612,#4807,.T.);
#9560=EDGE_CURVE('',#7613,#7616,#4808,.T.);
#9561=EDGE_CURVE('',#7617,#7616,#4809,.T.);
#9562=EDGE_CURVE('',#7614,#7617,#4810,.T.);
#9563=EDGE_CURVE('',#7616,#7618,#4811,.T.);
#9564=EDGE_CURVE('',#7619,#7618,#4812,.T.);
#9565=EDGE_CURVE('',#7617,#7619,#4813,.T.);
#9566=EDGE_CURVE('',#7618,#7612,#4814,.T.);
#9567=EDGE_CURVE('',#7619,#7615,#4815,.T.);
#9568=EDGE_CURVE('',#7620,#7621,#4816,.T.);
#9569=EDGE_CURVE('',#7622,#7621,#4817,.T.);
#9570=EDGE_CURVE('',#7623,#7622,#4818,.T.);
#9571=EDGE_CURVE('',#7623,#7620,#4819,.T.);
#9572=EDGE_CURVE('',#7621,#7624,#4820,.T.);
#9573=EDGE_CURVE('',#7625,#7624,#4821,.T.);
#9574=EDGE_CURVE('',#7622,#7625,#4822,.T.);
#9575=EDGE_CURVE('',#7624,#7626,#4823,.T.);
#9576=EDGE_CURVE('',#7627,#7626,#4824,.T.);
#9577=EDGE_CURVE('',#7625,#7627,#4825,.T.);
#9578=EDGE_CURVE('',#7626,#7620,#4826,.T.);
#9579=EDGE_CURVE('',#7627,#7623,#4827,.T.);
#9580=EDGE_CURVE('',#7628,#7629,#4828,.T.);
#9581=EDGE_CURVE('',#7630,#7629,#4829,.T.);
#9582=EDGE_CURVE('',#7631,#7630,#4830,.T.);
#9583=EDGE_CURVE('',#7631,#7628,#4831,.T.);
#9584=EDGE_CURVE('',#7629,#7632,#4832,.T.);
#9585=EDGE_CURVE('',#7633,#7632,#4833,.T.);
#9586=EDGE_CURVE('',#7630,#7633,#4834,.T.);
#9587=EDGE_CURVE('',#7632,#7634,#4835,.T.);
#9588=EDGE_CURVE('',#7635,#7634,#4836,.T.);
#9589=EDGE_CURVE('',#7633,#7635,#4837,.T.);
#9590=EDGE_CURVE('',#7634,#7628,#4838,.T.);
#9591=EDGE_CURVE('',#7635,#7631,#4839,.T.);
#9592=EDGE_CURVE('',#7636,#7637,#4840,.T.);
#9593=EDGE_CURVE('',#7638,#7637,#4841,.T.);
#9594=EDGE_CURVE('',#7639,#7638,#4842,.T.);
#9595=EDGE_CURVE('',#7639,#7636,#4843,.T.);
#9596=EDGE_CURVE('',#7637,#7640,#4844,.T.);
#9597=EDGE_CURVE('',#7641,#7640,#4845,.T.);
#9598=EDGE_CURVE('',#7638,#7641,#4846,.T.);
#9599=EDGE_CURVE('',#7640,#7642,#4847,.T.);
#9600=EDGE_CURVE('',#7643,#7642,#4848,.T.);
#9601=EDGE_CURVE('',#7641,#7643,#4849,.T.);
#9602=EDGE_CURVE('',#7642,#7636,#4850,.T.);
#9603=EDGE_CURVE('',#7643,#7639,#4851,.T.);
#9604=EDGE_CURVE('',#7644,#7645,#4852,.T.);
#9605=EDGE_CURVE('',#7646,#7645,#4853,.T.);
#9606=EDGE_CURVE('',#7647,#7646,#4854,.T.);
#9607=EDGE_CURVE('',#7647,#7644,#4855,.T.);
#9608=EDGE_CURVE('',#7645,#7648,#4856,.T.);
#9609=EDGE_CURVE('',#7649,#7648,#4857,.T.);
#9610=EDGE_CURVE('',#7646,#7649,#4858,.T.);
#9611=EDGE_CURVE('',#7648,#7650,#4859,.T.);
#9612=EDGE_CURVE('',#7651,#7650,#4860,.T.);
#9613=EDGE_CURVE('',#7649,#7651,#4861,.T.);
#9614=EDGE_CURVE('',#7650,#7644,#4862,.T.);
#9615=EDGE_CURVE('',#7651,#7647,#4863,.T.);
#9616=EDGE_CURVE('',#7652,#7653,#4864,.T.);
#9617=EDGE_CURVE('',#7654,#7653,#4865,.T.);
#9618=EDGE_CURVE('',#7655,#7654,#4866,.T.);
#9619=EDGE_CURVE('',#7655,#7652,#4867,.T.);
#9620=EDGE_CURVE('',#7653,#7656,#4868,.T.);
#9621=EDGE_CURVE('',#7657,#7656,#4869,.T.);
#9622=EDGE_CURVE('',#7654,#7657,#4870,.T.);
#9623=EDGE_CURVE('',#7656,#7658,#4871,.T.);
#9624=EDGE_CURVE('',#7659,#7658,#4872,.T.);
#9625=EDGE_CURVE('',#7657,#7659,#4873,.T.);
#9626=EDGE_CURVE('',#7658,#7652,#4874,.T.);
#9627=EDGE_CURVE('',#7659,#7655,#4875,.T.);
#9628=EDGE_CURVE('',#7660,#7661,#4876,.T.);
#9629=EDGE_CURVE('',#7662,#7661,#4877,.T.);
#9630=EDGE_CURVE('',#7663,#7662,#4878,.T.);
#9631=EDGE_CURVE('',#7663,#7660,#4879,.T.);
#9632=EDGE_CURVE('',#7661,#7664,#4880,.T.);
#9633=EDGE_CURVE('',#7665,#7664,#4881,.T.);
#9634=EDGE_CURVE('',#7662,#7665,#4882,.T.);
#9635=EDGE_CURVE('',#7664,#7666,#4883,.T.);
#9636=EDGE_CURVE('',#7667,#7666,#4884,.T.);
#9637=EDGE_CURVE('',#7665,#7667,#4885,.T.);
#9638=EDGE_CURVE('',#7666,#7660,#4886,.T.);
#9639=EDGE_CURVE('',#7667,#7663,#4887,.T.);
#9640=EDGE_CURVE('',#7668,#7669,#4888,.T.);
#9641=EDGE_CURVE('',#7670,#7669,#4889,.T.);
#9642=EDGE_CURVE('',#7671,#7670,#4890,.T.);
#9643=EDGE_CURVE('',#7671,#7668,#4891,.T.);
#9644=EDGE_CURVE('',#7669,#7672,#4892,.T.);
#9645=EDGE_CURVE('',#7673,#7672,#4893,.T.);
#9646=EDGE_CURVE('',#7670,#7673,#4894,.T.);
#9647=EDGE_CURVE('',#7672,#7674,#4895,.T.);
#9648=EDGE_CURVE('',#7675,#7674,#4896,.T.);
#9649=EDGE_CURVE('',#7673,#7675,#4897,.T.);
#9650=EDGE_CURVE('',#7674,#7668,#4898,.T.);
#9651=EDGE_CURVE('',#7675,#7671,#4899,.T.);
#9652=EDGE_CURVE('',#7676,#7677,#4900,.T.);
#9653=EDGE_CURVE('',#7678,#7677,#4901,.T.);
#9654=EDGE_CURVE('',#7679,#7678,#4902,.T.);
#9655=EDGE_CURVE('',#7679,#7676,#4903,.T.);
#9656=EDGE_CURVE('',#7677,#7680,#4904,.T.);
#9657=EDGE_CURVE('',#7681,#7680,#4905,.T.);
#9658=EDGE_CURVE('',#7678,#7681,#4906,.T.);
#9659=EDGE_CURVE('',#7680,#7682,#4907,.T.);
#9660=EDGE_CURVE('',#7683,#7682,#4908,.T.);
#9661=EDGE_CURVE('',#7681,#7683,#4909,.T.);
#9662=EDGE_CURVE('',#7682,#7676,#4910,.T.);
#9663=EDGE_CURVE('',#7683,#7679,#4911,.T.);
#9664=EDGE_CURVE('',#7684,#7685,#4912,.T.);
#9665=EDGE_CURVE('',#7686,#7684,#4913,.T.);
#9666=EDGE_CURVE('',#7686,#7687,#4914,.T.);
#9667=EDGE_CURVE('',#7687,#7685,#4915,.T.);
#9668=EDGE_CURVE('',#7685,#7688,#4916,.T.);
#9669=EDGE_CURVE('',#7687,#7689,#4917,.T.);
#9670=EDGE_CURVE('',#7689,#7688,#4918,.T.);
#9671=EDGE_CURVE('',#7688,#7690,#4919,.T.);
#9672=EDGE_CURVE('',#7689,#7691,#4920,.T.);
#9673=EDGE_CURVE('',#7691,#7690,#4921,.T.);
#9674=EDGE_CURVE('',#7690,#7684,#4922,.T.);
#9675=EDGE_CURVE('',#7691,#7686,#4923,.T.);
#9676=EDGE_CURVE('',#7692,#7693,#4924,.T.);
#9677=EDGE_CURVE('',#7694,#7692,#4925,.T.);
#9678=EDGE_CURVE('',#7694,#7695,#4926,.T.);
#9679=EDGE_CURVE('',#7695,#7693,#4927,.T.);
#9680=EDGE_CURVE('',#7693,#7696,#4928,.T.);
#9681=EDGE_CURVE('',#7695,#7697,#4929,.T.);
#9682=EDGE_CURVE('',#7697,#7696,#4930,.T.);
#9683=EDGE_CURVE('',#7696,#7698,#4931,.T.);
#9684=EDGE_CURVE('',#7697,#7699,#4932,.T.);
#9685=EDGE_CURVE('',#7699,#7698,#4933,.T.);
#9686=EDGE_CURVE('',#7698,#7692,#4934,.T.);
#9687=EDGE_CURVE('',#7699,#7694,#4935,.T.);
#9688=EDGE_CURVE('',#7700,#7701,#4936,.T.);
#9689=EDGE_CURVE('',#7702,#7700,#4937,.T.);
#9690=EDGE_CURVE('',#7702,#7703,#4938,.T.);
#9691=EDGE_CURVE('',#7703,#7701,#4939,.T.);
#9692=EDGE_CURVE('',#7701,#7704,#4940,.T.);
#9693=EDGE_CURVE('',#7703,#7705,#4941,.T.);
#9694=EDGE_CURVE('',#7705,#7704,#4942,.T.);
#9695=EDGE_CURVE('',#7704,#7706,#4943,.T.);
#9696=EDGE_CURVE('',#7705,#7707,#4944,.T.);
#9697=EDGE_CURVE('',#7707,#7706,#4945,.T.);
#9698=EDGE_CURVE('',#7706,#7700,#4946,.T.);
#9699=EDGE_CURVE('',#7707,#7702,#4947,.T.);
#9700=EDGE_CURVE('',#7708,#7709,#4948,.T.);
#9701=EDGE_CURVE('',#7710,#7708,#4949,.T.);
#9702=EDGE_CURVE('',#7710,#7711,#4950,.T.);
#9703=EDGE_CURVE('',#7711,#7709,#4951,.T.);
#9704=EDGE_CURVE('',#7709,#7712,#4952,.T.);
#9705=EDGE_CURVE('',#7711,#7713,#4953,.T.);
#9706=EDGE_CURVE('',#7713,#7712,#4954,.T.);
#9707=EDGE_CURVE('',#7712,#7714,#4955,.T.);
#9708=EDGE_CURVE('',#7713,#7715,#4956,.T.);
#9709=EDGE_CURVE('',#7715,#7714,#4957,.T.);
#9710=EDGE_CURVE('',#7714,#7708,#4958,.T.);
#9711=EDGE_CURVE('',#7715,#7710,#4959,.T.);
#9712=EDGE_CURVE('',#7716,#7717,#4960,.T.);
#9713=EDGE_CURVE('',#7718,#7716,#4961,.T.);
#9714=EDGE_CURVE('',#7718,#7719,#4962,.T.);
#9715=EDGE_CURVE('',#7719,#7717,#4963,.T.);
#9716=EDGE_CURVE('',#7717,#7720,#4964,.T.);
#9717=EDGE_CURVE('',#7719,#7721,#4965,.T.);
#9718=EDGE_CURVE('',#7721,#7720,#4966,.T.);
#9719=EDGE_CURVE('',#7720,#7722,#4967,.T.);
#9720=EDGE_CURVE('',#7721,#7723,#4968,.T.);
#9721=EDGE_CURVE('',#7723,#7722,#4969,.T.);
#9722=EDGE_CURVE('',#7722,#7716,#4970,.T.);
#9723=EDGE_CURVE('',#7723,#7718,#4971,.T.);
#9724=EDGE_CURVE('',#7724,#7725,#4972,.T.);
#9725=EDGE_CURVE('',#7726,#7725,#4973,.T.);
#9726=EDGE_CURVE('',#7727,#7726,#4974,.T.);
#9727=EDGE_CURVE('',#7727,#7724,#4975,.T.);
#9728=EDGE_CURVE('',#7725,#7728,#4976,.T.);
#9729=EDGE_CURVE('',#7729,#7728,#4977,.T.);
#9730=EDGE_CURVE('',#7726,#7729,#4978,.T.);
#9731=EDGE_CURVE('',#7728,#7730,#4979,.T.);
#9732=EDGE_CURVE('',#7731,#7730,#4980,.T.);
#9733=EDGE_CURVE('',#7729,#7731,#4981,.T.);
#9734=EDGE_CURVE('',#7730,#7724,#4982,.T.);
#9735=EDGE_CURVE('',#7731,#7727,#4983,.T.);
#9736=EDGE_CURVE('',#7732,#7733,#4984,.T.);
#9737=EDGE_CURVE('',#7734,#7733,#4985,.T.);
#9738=EDGE_CURVE('',#7735,#7734,#4986,.T.);
#9739=EDGE_CURVE('',#7735,#7732,#4987,.T.);
#9740=EDGE_CURVE('',#7733,#7736,#4988,.T.);
#9741=EDGE_CURVE('',#7737,#7736,#4989,.T.);
#9742=EDGE_CURVE('',#7734,#7737,#4990,.T.);
#9743=EDGE_CURVE('',#7736,#7738,#4991,.T.);
#9744=EDGE_CURVE('',#7739,#7738,#4992,.T.);
#9745=EDGE_CURVE('',#7737,#7739,#4993,.T.);
#9746=EDGE_CURVE('',#7738,#7732,#4994,.T.);
#9747=EDGE_CURVE('',#7739,#7735,#4995,.T.);
#9748=EDGE_CURVE('',#7740,#7741,#4996,.T.);
#9749=EDGE_CURVE('',#7742,#7741,#4997,.T.);
#9750=EDGE_CURVE('',#7743,#7742,#4998,.T.);
#9751=EDGE_CURVE('',#7743,#7740,#4999,.T.);
#9752=EDGE_CURVE('',#7741,#7744,#5000,.T.);
#9753=EDGE_CURVE('',#7745,#7744,#5001,.T.);
#9754=EDGE_CURVE('',#7742,#7745,#5002,.T.);
#9755=EDGE_CURVE('',#7744,#7746,#5003,.T.);
#9756=EDGE_CURVE('',#7747,#7746,#5004,.T.);
#9757=EDGE_CURVE('',#7745,#7747,#5005,.T.);
#9758=EDGE_CURVE('',#7746,#7740,#5006,.T.);
#9759=EDGE_CURVE('',#7747,#7743,#5007,.T.);
#9760=EDGE_CURVE('',#7748,#7749,#5008,.T.);
#9761=EDGE_CURVE('',#7750,#7749,#5009,.T.);
#9762=EDGE_CURVE('',#7751,#7750,#5010,.T.);
#9763=EDGE_CURVE('',#7751,#7748,#5011,.T.);
#9764=EDGE_CURVE('',#7749,#7752,#5012,.T.);
#9765=EDGE_CURVE('',#7753,#7752,#5013,.T.);
#9766=EDGE_CURVE('',#7750,#7753,#5014,.T.);
#9767=EDGE_CURVE('',#7752,#7754,#5015,.T.);
#9768=EDGE_CURVE('',#7755,#7754,#5016,.T.);
#9769=EDGE_CURVE('',#7753,#7755,#5017,.T.);
#9770=EDGE_CURVE('',#7754,#7748,#5018,.T.);
#9771=EDGE_CURVE('',#7755,#7751,#5019,.T.);
#9772=EDGE_CURVE('',#7756,#7757,#5020,.T.);
#9773=EDGE_CURVE('',#7758,#7757,#5021,.T.);
#9774=EDGE_CURVE('',#7759,#7758,#5022,.T.);
#9775=EDGE_CURVE('',#7759,#7756,#5023,.T.);
#9776=EDGE_CURVE('',#7757,#7760,#5024,.T.);
#9777=EDGE_CURVE('',#7761,#7760,#5025,.T.);
#9778=EDGE_CURVE('',#7758,#7761,#5026,.T.);
#9779=EDGE_CURVE('',#7760,#7762,#5027,.T.);
#9780=EDGE_CURVE('',#7763,#7762,#5028,.T.);
#9781=EDGE_CURVE('',#7761,#7763,#5029,.T.);
#9782=EDGE_CURVE('',#7762,#7756,#5030,.T.);
#9783=EDGE_CURVE('',#7763,#7759,#5031,.T.);
#9784=EDGE_CURVE('',#7764,#7765,#5032,.T.);
#9785=EDGE_CURVE('',#7766,#7765,#5033,.T.);
#9786=EDGE_CURVE('',#7767,#7766,#5034,.T.);
#9787=EDGE_CURVE('',#7767,#7764,#5035,.T.);
#9788=EDGE_CURVE('',#7765,#7768,#5036,.T.);
#9789=EDGE_CURVE('',#7769,#7768,#5037,.T.);
#9790=EDGE_CURVE('',#7766,#7769,#5038,.T.);
#9791=EDGE_CURVE('',#7768,#7770,#5039,.T.);
#9792=EDGE_CURVE('',#7771,#7770,#5040,.T.);
#9793=EDGE_CURVE('',#7769,#7771,#5041,.T.);
#9794=EDGE_CURVE('',#7770,#7764,#5042,.T.);
#9795=EDGE_CURVE('',#7771,#7767,#5043,.T.);
#12121=ORIENTED_EDGE('',*,*,#8944,.T.);
#12122=ORIENTED_EDGE('',*,*,#8945,.F.);
#12123=ORIENTED_EDGE('',*,*,#8946,.F.);
#12124=ORIENTED_EDGE('',*,*,#8947,.T.);
#12125=ORIENTED_EDGE('',*,*,#8948,.T.);
#12126=ORIENTED_EDGE('',*,*,#8949,.F.);
#12127=ORIENTED_EDGE('',*,*,#8950,.F.);
#12128=ORIENTED_EDGE('',*,*,#8945,.T.);
#12129=ORIENTED_EDGE('',*,*,#8951,.T.);
#12130=ORIENTED_EDGE('',*,*,#8952,.F.);
#12131=ORIENTED_EDGE('',*,*,#8953,.F.);
#12132=ORIENTED_EDGE('',*,*,#8949,.T.);
#12133=ORIENTED_EDGE('',*,*,#8954,.T.);
#12134=ORIENTED_EDGE('',*,*,#8947,.F.);
#12135=ORIENTED_EDGE('',*,*,#8955,.F.);
#12136=ORIENTED_EDGE('',*,*,#8952,.T.);
#12137=ORIENTED_EDGE('',*,*,#8946,.T.);
#12138=ORIENTED_EDGE('',*,*,#8950,.T.);
#12139=ORIENTED_EDGE('',*,*,#8953,.T.);
#12140=ORIENTED_EDGE('',*,*,#8955,.T.);
#12141=ORIENTED_EDGE('',*,*,#8944,.F.);
#12142=ORIENTED_EDGE('',*,*,#8954,.F.);
#12143=ORIENTED_EDGE('',*,*,#8951,.F.);
#12144=ORIENTED_EDGE('',*,*,#8948,.F.);
#12145=ORIENTED_EDGE('',*,*,#8956,.T.);
#12146=ORIENTED_EDGE('',*,*,#8957,.T.);
#12147=ORIENTED_EDGE('',*,*,#8958,.F.);
#12148=ORIENTED_EDGE('',*,*,#8957,.F.);
#12149=ORIENTED_EDGE('',*,*,#8959,.T.);
#12150=ORIENTED_EDGE('',*,*,#8960,.T.);
#12151=ORIENTED_EDGE('',*,*,#8961,.T.);
#12152=ORIENTED_EDGE('',*,*,#8962,.T.);
#12153=ORIENTED_EDGE('',*,*,#8963,.T.);
#12154=ORIENTED_EDGE('',*,*,#8964,.T.);
#12155=ORIENTED_EDGE('',*,*,#8956,.F.);
#12156=ORIENTED_EDGE('',*,*,#8965,.F.);
#12157=ORIENTED_EDGE('',*,*,#8966,.F.);
#12158=ORIENTED_EDGE('',*,*,#8967,.F.);
#12159=ORIENTED_EDGE('',*,*,#8968,.F.);
#12160=ORIENTED_EDGE('',*,*,#8969,.F.);
#12161=ORIENTED_EDGE('',*,*,#8970,.F.);
#12162=ORIENTED_EDGE('',*,*,#8958,.T.);
#12163=ORIENTED_EDGE('',*,*,#8965,.T.);
#12164=ORIENTED_EDGE('',*,*,#8971,.F.);
#12165=ORIENTED_EDGE('',*,*,#8959,.F.);
#12166=ORIENTED_EDGE('',*,*,#8972,.T.);
#12167=ORIENTED_EDGE('',*,*,#8970,.T.);
#12168=ORIENTED_EDGE('',*,*,#8973,.F.);
#12169=ORIENTED_EDGE('',*,*,#8960,.F.);
#12170=ORIENTED_EDGE('',*,*,#8971,.T.);
#12171=ORIENTED_EDGE('',*,*,#8969,.T.);
#12172=ORIENTED_EDGE('',*,*,#8974,.F.);
#12173=ORIENTED_EDGE('',*,*,#8961,.F.);
#12174=ORIENTED_EDGE('',*,*,#8973,.T.);
#12175=ORIENTED_EDGE('',*,*,#8968,.T.);
#12176=ORIENTED_EDGE('',*,*,#8975,.F.);
#12177=ORIENTED_EDGE('',*,*,#8962,.F.);
#12178=ORIENTED_EDGE('',*,*,#8974,.T.);
#12179=ORIENTED_EDGE('',*,*,#8967,.T.);
#12180=ORIENTED_EDGE('',*,*,#8976,.F.);
#12181=ORIENTED_EDGE('',*,*,#8963,.F.);
#12182=ORIENTED_EDGE('',*,*,#8975,.T.);
#12183=ORIENTED_EDGE('',*,*,#8966,.T.);
#12184=ORIENTED_EDGE('',*,*,#8972,.F.);
#12185=ORIENTED_EDGE('',*,*,#8964,.F.);
#12186=ORIENTED_EDGE('',*,*,#8976,.T.);
#12187=ORIENTED_EDGE('',*,*,#8977,.F.);
#12188=ORIENTED_EDGE('',*,*,#8978,.T.);
#12189=ORIENTED_EDGE('',*,*,#8979,.T.);
#12190=ORIENTED_EDGE('',*,*,#8978,.F.);
#12191=ORIENTED_EDGE('',*,*,#8980,.F.);
#12192=ORIENTED_EDGE('',*,*,#8981,.F.);
#12193=ORIENTED_EDGE('',*,*,#8982,.F.);
#12194=ORIENTED_EDGE('',*,*,#8983,.F.);
#12195=ORIENTED_EDGE('',*,*,#8984,.F.);
#12196=ORIENTED_EDGE('',*,*,#8985,.F.);
#12197=ORIENTED_EDGE('',*,*,#8977,.T.);
#12198=ORIENTED_EDGE('',*,*,#8986,.T.);
#12199=ORIENTED_EDGE('',*,*,#8987,.T.);
#12200=ORIENTED_EDGE('',*,*,#8988,.T.);
#12201=ORIENTED_EDGE('',*,*,#8989,.T.);
#12202=ORIENTED_EDGE('',*,*,#8990,.T.);
#12203=ORIENTED_EDGE('',*,*,#8991,.T.);
#12204=ORIENTED_EDGE('',*,*,#8979,.F.);
#12205=ORIENTED_EDGE('',*,*,#8986,.F.);
#12206=ORIENTED_EDGE('',*,*,#8992,.F.);
#12207=ORIENTED_EDGE('',*,*,#8980,.T.);
#12208=ORIENTED_EDGE('',*,*,#8993,.T.);
#12209=ORIENTED_EDGE('',*,*,#8987,.F.);
#12210=ORIENTED_EDGE('',*,*,#8993,.F.);
#12211=ORIENTED_EDGE('',*,*,#8985,.T.);
#12212=ORIENTED_EDGE('',*,*,#8994,.T.);
#12213=ORIENTED_EDGE('',*,*,#8988,.F.);
#12214=ORIENTED_EDGE('',*,*,#8994,.F.);
#12215=ORIENTED_EDGE('',*,*,#8984,.T.);
#12216=ORIENTED_EDGE('',*,*,#8995,.T.);
#12217=ORIENTED_EDGE('',*,*,#8989,.F.);
#12218=ORIENTED_EDGE('',*,*,#8995,.F.);
#12219=ORIENTED_EDGE('',*,*,#8983,.T.);
#12220=ORIENTED_EDGE('',*,*,#8996,.T.);
#12221=ORIENTED_EDGE('',*,*,#8990,.F.);
#12222=ORIENTED_EDGE('',*,*,#8996,.F.);
#12223=ORIENTED_EDGE('',*,*,#8982,.T.);
#12224=ORIENTED_EDGE('',*,*,#8997,.T.);
#12225=ORIENTED_EDGE('',*,*,#8991,.F.);
#12226=ORIENTED_EDGE('',*,*,#8997,.F.);
#12227=ORIENTED_EDGE('',*,*,#8981,.T.);
#12228=ORIENTED_EDGE('',*,*,#8992,.T.);
#12229=ORIENTED_EDGE('',*,*,#8998,.T.);
#12230=ORIENTED_EDGE('',*,*,#8999,.T.);
#12231=ORIENTED_EDGE('',*,*,#9000,.F.);
#12232=ORIENTED_EDGE('',*,*,#8999,.F.);
#12233=ORIENTED_EDGE('',*,*,#9001,.T.);
#12234=ORIENTED_EDGE('',*,*,#9002,.T.);
#12235=ORIENTED_EDGE('',*,*,#9003,.F.);
#12236=ORIENTED_EDGE('',*,*,#9002,.F.);
#12237=ORIENTED_EDGE('',*,*,#9004,.T.);
#12238=ORIENTED_EDGE('',*,*,#9005,.T.);
#12239=ORIENTED_EDGE('',*,*,#9006,.F.);
#12240=ORIENTED_EDGE('',*,*,#9005,.F.);
#12241=ORIENTED_EDGE('',*,*,#9007,.T.);
#12242=ORIENTED_EDGE('',*,*,#9008,.T.);
#12243=ORIENTED_EDGE('',*,*,#9009,.F.);
#12244=ORIENTED_EDGE('',*,*,#9008,.F.);
#12245=ORIENTED_EDGE('',*,*,#9010,.T.);
#12246=ORIENTED_EDGE('',*,*,#9011,.T.);
#12247=ORIENTED_EDGE('',*,*,#9012,.F.);
#12248=ORIENTED_EDGE('',*,*,#9011,.F.);
#12249=ORIENTED_EDGE('',*,*,#9013,.T.);
#12250=ORIENTED_EDGE('',*,*,#9014,.T.);
#12251=ORIENTED_EDGE('',*,*,#9015,.T.);
#12252=ORIENTED_EDGE('',*,*,#9016,.T.);
#12253=ORIENTED_EDGE('',*,*,#9017,.T.);
#12254=ORIENTED_EDGE('',*,*,#9018,.T.);
#12255=ORIENTED_EDGE('',*,*,#9019,.T.);
#12256=ORIENTED_EDGE('',*,*,#9020,.T.);
#12257=ORIENTED_EDGE('',*,*,#9010,.F.);
#12258=ORIENTED_EDGE('',*,*,#9007,.F.);
#12259=ORIENTED_EDGE('',*,*,#9004,.F.);
#12260=ORIENTED_EDGE('',*,*,#9001,.F.);
#12261=ORIENTED_EDGE('',*,*,#8998,.F.);
#12262=ORIENTED_EDGE('',*,*,#9021,.F.);
#12263=ORIENTED_EDGE('',*,*,#9022,.F.);
#12264=ORIENTED_EDGE('',*,*,#9023,.F.);
#12265=ORIENTED_EDGE('',*,*,#9024,.F.);
#12266=ORIENTED_EDGE('',*,*,#9025,.F.);
#12267=ORIENTED_EDGE('',*,*,#9026,.F.);
#12268=ORIENTED_EDGE('',*,*,#9027,.F.);
#12269=ORIENTED_EDGE('',*,*,#9028,.F.);
#12270=ORIENTED_EDGE('',*,*,#9012,.T.);
#12271=ORIENTED_EDGE('',*,*,#9006,.T.);
#12272=ORIENTED_EDGE('',*,*,#9000,.T.);
#12273=ORIENTED_EDGE('',*,*,#9003,.T.);
#12274=ORIENTED_EDGE('',*,*,#9009,.T.);
#12275=ORIENTED_EDGE('',*,*,#9021,.T.);
#12276=ORIENTED_EDGE('',*,*,#9029,.F.);
#12277=ORIENTED_EDGE('',*,*,#9013,.F.);
#12278=ORIENTED_EDGE('',*,*,#9030,.T.);
#12279=ORIENTED_EDGE('',*,*,#9028,.T.);
#12280=ORIENTED_EDGE('',*,*,#9031,.F.);
#12281=ORIENTED_EDGE('',*,*,#9014,.F.);
#12282=ORIENTED_EDGE('',*,*,#9029,.T.);
#12283=ORIENTED_EDGE('',*,*,#9027,.T.);
#12284=ORIENTED_EDGE('',*,*,#9032,.F.);
#12285=ORIENTED_EDGE('',*,*,#9015,.F.);
#12286=ORIENTED_EDGE('',*,*,#9031,.T.);
#12287=ORIENTED_EDGE('',*,*,#9026,.T.);
#12288=ORIENTED_EDGE('',*,*,#9033,.F.);
#12289=ORIENTED_EDGE('',*,*,#9016,.F.);
#12290=ORIENTED_EDGE('',*,*,#9032,.T.);
#12291=ORIENTED_EDGE('',*,*,#9025,.T.);
#12292=ORIENTED_EDGE('',*,*,#9034,.F.);
#12293=ORIENTED_EDGE('',*,*,#9017,.F.);
#12294=ORIENTED_EDGE('',*,*,#9033,.T.);
#12295=ORIENTED_EDGE('',*,*,#9024,.T.);
#12296=ORIENTED_EDGE('',*,*,#9035,.F.);
#12297=ORIENTED_EDGE('',*,*,#9018,.F.);
#12298=ORIENTED_EDGE('',*,*,#9034,.T.);
#12299=ORIENTED_EDGE('',*,*,#9023,.T.);
#12300=ORIENTED_EDGE('',*,*,#9036,.F.);
#12301=ORIENTED_EDGE('',*,*,#9019,.F.);
#12302=ORIENTED_EDGE('',*,*,#9035,.T.);
#12303=ORIENTED_EDGE('',*,*,#9022,.T.);
#12304=ORIENTED_EDGE('',*,*,#9030,.F.);
#12305=ORIENTED_EDGE('',*,*,#9020,.F.);
#12306=ORIENTED_EDGE('',*,*,#9036,.T.);
#12307=ORIENTED_EDGE('',*,*,#9037,.T.);
#12308=ORIENTED_EDGE('',*,*,#9038,.F.);
#12309=ORIENTED_EDGE('',*,*,#9039,.F.);
#12310=ORIENTED_EDGE('',*,*,#9040,.T.);
#12311=ORIENTED_EDGE('',*,*,#9041,.T.);
#12312=ORIENTED_EDGE('',*,*,#9042,.F.);
#12313=ORIENTED_EDGE('',*,*,#9043,.F.);
#12314=ORIENTED_EDGE('',*,*,#9038,.T.);
#12315=ORIENTED_EDGE('',*,*,#9044,.T.);
#12316=ORIENTED_EDGE('',*,*,#9045,.F.);
#12317=ORIENTED_EDGE('',*,*,#9046,.F.);
#12318=ORIENTED_EDGE('',*,*,#9042,.T.);
#12319=ORIENTED_EDGE('',*,*,#9047,.T.);
#12320=ORIENTED_EDGE('',*,*,#9040,.F.);
#12321=ORIENTED_EDGE('',*,*,#9048,.F.);
#12322=ORIENTED_EDGE('',*,*,#9045,.T.);
#12323=ORIENTED_EDGE('',*,*,#9039,.T.);
#12324=ORIENTED_EDGE('',*,*,#9043,.T.);
#12325=ORIENTED_EDGE('',*,*,#9046,.T.);
#12326=ORIENTED_EDGE('',*,*,#9048,.T.);
#12327=ORIENTED_EDGE('',*,*,#9037,.F.);
#12328=ORIENTED_EDGE('',*,*,#9047,.F.);
#12329=ORIENTED_EDGE('',*,*,#9044,.F.);
#12330=ORIENTED_EDGE('',*,*,#9041,.F.);
#12331=ORIENTED_EDGE('',*,*,#9049,.T.);
#12332=ORIENTED_EDGE('',*,*,#9050,.F.);
#12333=ORIENTED_EDGE('',*,*,#9051,.F.);
#12334=ORIENTED_EDGE('',*,*,#9052,.T.);
#12335=ORIENTED_EDGE('',*,*,#9053,.T.);
#12336=ORIENTED_EDGE('',*,*,#9054,.F.);
#12337=ORIENTED_EDGE('',*,*,#9055,.F.);
#12338=ORIENTED_EDGE('',*,*,#9050,.T.);
#12339=ORIENTED_EDGE('',*,*,#9056,.T.);
#12340=ORIENTED_EDGE('',*,*,#9057,.F.);
#12341=ORIENTED_EDGE('',*,*,#9058,.F.);
#12342=ORIENTED_EDGE('',*,*,#9054,.T.);
#12343=ORIENTED_EDGE('',*,*,#9059,.T.);
#12344=ORIENTED_EDGE('',*,*,#9052,.F.);
#12345=ORIENTED_EDGE('',*,*,#9060,.F.);
#12346=ORIENTED_EDGE('',*,*,#9057,.T.);
#12347=ORIENTED_EDGE('',*,*,#9051,.T.);
#12348=ORIENTED_EDGE('',*,*,#9055,.T.);
#12349=ORIENTED_EDGE('',*,*,#9058,.T.);
#12350=ORIENTED_EDGE('',*,*,#9060,.T.);
#12351=ORIENTED_EDGE('',*,*,#9049,.F.);
#12352=ORIENTED_EDGE('',*,*,#9059,.F.);
#12353=ORIENTED_EDGE('',*,*,#9056,.F.);
#12354=ORIENTED_EDGE('',*,*,#9053,.F.);
#12355=ORIENTED_EDGE('',*,*,#9061,.T.);
#12356=ORIENTED_EDGE('',*,*,#9062,.F.);
#12357=ORIENTED_EDGE('',*,*,#9063,.F.);
#12358=ORIENTED_EDGE('',*,*,#9064,.T.);
#12359=ORIENTED_EDGE('',*,*,#9065,.T.);
#12360=ORIENTED_EDGE('',*,*,#9066,.F.);
#12361=ORIENTED_EDGE('',*,*,#9067,.F.);
#12362=ORIENTED_EDGE('',*,*,#9062,.T.);
#12363=ORIENTED_EDGE('',*,*,#9068,.T.);
#12364=ORIENTED_EDGE('',*,*,#9069,.F.);
#12365=ORIENTED_EDGE('',*,*,#9070,.F.);
#12366=ORIENTED_EDGE('',*,*,#9066,.T.);
#12367=ORIENTED_EDGE('',*,*,#9071,.T.);
#12368=ORIENTED_EDGE('',*,*,#9072,.F.);
#12369=ORIENTED_EDGE('',*,*,#9073,.F.);
#12370=ORIENTED_EDGE('',*,*,#9069,.T.);
#12371=ORIENTED_EDGE('',*,*,#9074,.T.);
#12372=ORIENTED_EDGE('',*,*,#9075,.F.);
#12373=ORIENTED_EDGE('',*,*,#9076,.F.);
#12374=ORIENTED_EDGE('',*,*,#9072,.T.);
#12375=ORIENTED_EDGE('',*,*,#9077,.T.);
#12376=ORIENTED_EDGE('',*,*,#9064,.F.);
#12377=ORIENTED_EDGE('',*,*,#9078,.F.);
#12378=ORIENTED_EDGE('',*,*,#9075,.T.);
#12379=ORIENTED_EDGE('',*,*,#9063,.T.);
#12380=ORIENTED_EDGE('',*,*,#9067,.T.);
#12381=ORIENTED_EDGE('',*,*,#9070,.T.);
#12382=ORIENTED_EDGE('',*,*,#9073,.T.);
#12383=ORIENTED_EDGE('',*,*,#9076,.T.);
#12384=ORIENTED_EDGE('',*,*,#9078,.T.);
#12385=ORIENTED_EDGE('',*,*,#9061,.F.);
#12386=ORIENTED_EDGE('',*,*,#9077,.F.);
#12387=ORIENTED_EDGE('',*,*,#9074,.F.);
#12388=ORIENTED_EDGE('',*,*,#9071,.F.);
#12389=ORIENTED_EDGE('',*,*,#9068,.F.);
#12390=ORIENTED_EDGE('',*,*,#9065,.F.);
#12391=ORIENTED_EDGE('',*,*,#9079,.T.);
#12392=ORIENTED_EDGE('',*,*,#9080,.T.);
#12393=ORIENTED_EDGE('',*,*,#9081,.F.);
#12394=ORIENTED_EDGE('',*,*,#9080,.F.);
#12395=ORIENTED_EDGE('',*,*,#9082,.T.);
#12396=ORIENTED_EDGE('',*,*,#9083,.T.);
#12397=ORIENTED_EDGE('',*,*,#9084,.F.);
#12398=ORIENTED_EDGE('',*,*,#9083,.F.);
#12399=ORIENTED_EDGE('',*,*,#9085,.T.);
#12400=ORIENTED_EDGE('',*,*,#9086,.T.);
#12401=ORIENTED_EDGE('',*,*,#9087,.F.);
#12402=ORIENTED_EDGE('',*,*,#9086,.F.);
#12403=ORIENTED_EDGE('',*,*,#9088,.T.);
#12404=ORIENTED_EDGE('',*,*,#9089,.T.);
#12405=ORIENTED_EDGE('',*,*,#9090,.T.);
#12406=ORIENTED_EDGE('',*,*,#9091,.T.);
#12407=ORIENTED_EDGE('',*,*,#9085,.F.);
#12408=ORIENTED_EDGE('',*,*,#9079,.F.);
#12409=ORIENTED_EDGE('',*,*,#9082,.F.);
#12410=ORIENTED_EDGE('',*,*,#9092,.F.);
#12411=ORIENTED_EDGE('',*,*,#9093,.F.);
#12412=ORIENTED_EDGE('',*,*,#9094,.F.);
#12413=ORIENTED_EDGE('',*,*,#9095,.F.);
#12414=ORIENTED_EDGE('',*,*,#9087,.T.);
#12415=ORIENTED_EDGE('',*,*,#9084,.T.);
#12416=ORIENTED_EDGE('',*,*,#9081,.T.);
#12417=ORIENTED_EDGE('',*,*,#9092,.T.);
#12418=ORIENTED_EDGE('',*,*,#9096,.F.);
#12419=ORIENTED_EDGE('',*,*,#9088,.F.);
#12420=ORIENTED_EDGE('',*,*,#9097,.T.);
#12421=ORIENTED_EDGE('',*,*,#9095,.T.);
#12422=ORIENTED_EDGE('',*,*,#9098,.F.);
#12423=ORIENTED_EDGE('',*,*,#9089,.F.);
#12424=ORIENTED_EDGE('',*,*,#9096,.T.);
#12425=ORIENTED_EDGE('',*,*,#9094,.T.);
#12426=ORIENTED_EDGE('',*,*,#9099,.F.);
#12427=ORIENTED_EDGE('',*,*,#9090,.F.);
#12428=ORIENTED_EDGE('',*,*,#9098,.T.);
#12429=ORIENTED_EDGE('',*,*,#9093,.T.);
#12430=ORIENTED_EDGE('',*,*,#9097,.F.);
#12431=ORIENTED_EDGE('',*,*,#9091,.F.);
#12432=ORIENTED_EDGE('',*,*,#9099,.T.);
#12433=ORIENTED_EDGE('',*,*,#9100,.T.);
#12434=ORIENTED_EDGE('',*,*,#9101,.T.);
#12435=ORIENTED_EDGE('',*,*,#9102,.F.);
#12436=ORIENTED_EDGE('',*,*,#9101,.F.);
#12437=ORIENTED_EDGE('',*,*,#9103,.T.);
#12438=ORIENTED_EDGE('',*,*,#9104,.T.);
#12439=ORIENTED_EDGE('',*,*,#9105,.F.);
#12440=ORIENTED_EDGE('',*,*,#9104,.F.);
#12441=ORIENTED_EDGE('',*,*,#9106,.T.);
#12442=ORIENTED_EDGE('',*,*,#9107,.T.);
#12443=ORIENTED_EDGE('',*,*,#9108,.F.);
#12444=ORIENTED_EDGE('',*,*,#9107,.F.);
#12445=ORIENTED_EDGE('',*,*,#9109,.T.);
#12446=ORIENTED_EDGE('',*,*,#9110,.T.);
#12447=ORIENTED_EDGE('',*,*,#9111,.T.);
#12448=ORIENTED_EDGE('',*,*,#9112,.T.);
#12449=ORIENTED_EDGE('',*,*,#9106,.F.);
#12450=ORIENTED_EDGE('',*,*,#9100,.F.);
#12451=ORIENTED_EDGE('',*,*,#9103,.F.);
#12452=ORIENTED_EDGE('',*,*,#9113,.F.);
#12453=ORIENTED_EDGE('',*,*,#9114,.F.);
#12454=ORIENTED_EDGE('',*,*,#9115,.F.);
#12455=ORIENTED_EDGE('',*,*,#9116,.F.);
#12456=ORIENTED_EDGE('',*,*,#9108,.T.);
#12457=ORIENTED_EDGE('',*,*,#9105,.T.);
#12458=ORIENTED_EDGE('',*,*,#9102,.T.);
#12459=ORIENTED_EDGE('',*,*,#9113,.T.);
#12460=ORIENTED_EDGE('',*,*,#9117,.F.);
#12461=ORIENTED_EDGE('',*,*,#9109,.F.);
#12462=ORIENTED_EDGE('',*,*,#9118,.T.);
#12463=ORIENTED_EDGE('',*,*,#9116,.T.);
#12464=ORIENTED_EDGE('',*,*,#9119,.F.);
#12465=ORIENTED_EDGE('',*,*,#9110,.F.);
#12466=ORIENTED_EDGE('',*,*,#9117,.T.);
#12467=ORIENTED_EDGE('',*,*,#9115,.T.);
#12468=ORIENTED_EDGE('',*,*,#9120,.F.);
#12469=ORIENTED_EDGE('',*,*,#9111,.F.);
#12470=ORIENTED_EDGE('',*,*,#9119,.T.);
#12471=ORIENTED_EDGE('',*,*,#9114,.T.);
#12472=ORIENTED_EDGE('',*,*,#9118,.F.);
#12473=ORIENTED_EDGE('',*,*,#9112,.F.);
#12474=ORIENTED_EDGE('',*,*,#9120,.T.);
#12475=ORIENTED_EDGE('',*,*,#9121,.T.);
#12476=ORIENTED_EDGE('',*,*,#9122,.T.);
#12477=ORIENTED_EDGE('',*,*,#9123,.F.);
#12478=ORIENTED_EDGE('',*,*,#9122,.F.);
#12479=ORIENTED_EDGE('',*,*,#9124,.T.);
#12480=ORIENTED_EDGE('',*,*,#9125,.T.);
#12481=ORIENTED_EDGE('',*,*,#9126,.F.);
#12482=ORIENTED_EDGE('',*,*,#9125,.F.);
#12483=ORIENTED_EDGE('',*,*,#9127,.T.);
#12484=ORIENTED_EDGE('',*,*,#9128,.T.);
#12485=ORIENTED_EDGE('',*,*,#9129,.F.);
#12486=ORIENTED_EDGE('',*,*,#9128,.F.);
#12487=ORIENTED_EDGE('',*,*,#9130,.T.);
#12488=ORIENTED_EDGE('',*,*,#9131,.T.);
#12489=ORIENTED_EDGE('',*,*,#9132,.T.);
#12490=ORIENTED_EDGE('',*,*,#9133,.T.);
#12491=ORIENTED_EDGE('',*,*,#9127,.F.);
#12492=ORIENTED_EDGE('',*,*,#9121,.F.);
#12493=ORIENTED_EDGE('',*,*,#9124,.F.);
#12494=ORIENTED_EDGE('',*,*,#9134,.F.);
#12495=ORIENTED_EDGE('',*,*,#9135,.F.);
#12496=ORIENTED_EDGE('',*,*,#9136,.F.);
#12497=ORIENTED_EDGE('',*,*,#9137,.F.);
#12498=ORIENTED_EDGE('',*,*,#9129,.T.);
#12499=ORIENTED_EDGE('',*,*,#9126,.T.);
#12500=ORIENTED_EDGE('',*,*,#9123,.T.);
#12501=ORIENTED_EDGE('',*,*,#9134,.T.);
#12502=ORIENTED_EDGE('',*,*,#9138,.F.);
#12503=ORIENTED_EDGE('',*,*,#9130,.F.);
#12504=ORIENTED_EDGE('',*,*,#9139,.T.);
#12505=ORIENTED_EDGE('',*,*,#9137,.T.);
#12506=ORIENTED_EDGE('',*,*,#9140,.F.);
#12507=ORIENTED_EDGE('',*,*,#9131,.F.);
#12508=ORIENTED_EDGE('',*,*,#9138,.T.);
#12509=ORIENTED_EDGE('',*,*,#9136,.T.);
#12510=ORIENTED_EDGE('',*,*,#9141,.F.);
#12511=ORIENTED_EDGE('',*,*,#9132,.F.);
#12512=ORIENTED_EDGE('',*,*,#9140,.T.);
#12513=ORIENTED_EDGE('',*,*,#9135,.T.);
#12514=ORIENTED_EDGE('',*,*,#9139,.F.);
#12515=ORIENTED_EDGE('',*,*,#9133,.F.);
#12516=ORIENTED_EDGE('',*,*,#9141,.T.);
#12517=ORIENTED_EDGE('',*,*,#9142,.T.);
#12518=ORIENTED_EDGE('',*,*,#9143,.T.);
#12519=ORIENTED_EDGE('',*,*,#9144,.F.);
#12520=ORIENTED_EDGE('',*,*,#9143,.F.);
#12521=ORIENTED_EDGE('',*,*,#9145,.T.);
#12522=ORIENTED_EDGE('',*,*,#9146,.T.);
#12523=ORIENTED_EDGE('',*,*,#9147,.F.);
#12524=ORIENTED_EDGE('',*,*,#9146,.F.);
#12525=ORIENTED_EDGE('',*,*,#9148,.T.);
#12526=ORIENTED_EDGE('',*,*,#9149,.T.);
#12527=ORIENTED_EDGE('',*,*,#9150,.F.);
#12528=ORIENTED_EDGE('',*,*,#9149,.F.);
#12529=ORIENTED_EDGE('',*,*,#9151,.T.);
#12530=ORIENTED_EDGE('',*,*,#9152,.T.);
#12531=ORIENTED_EDGE('',*,*,#9153,.T.);
#12532=ORIENTED_EDGE('',*,*,#9154,.T.);
#12533=ORIENTED_EDGE('',*,*,#9148,.F.);
#12534=ORIENTED_EDGE('',*,*,#9142,.F.);
#12535=ORIENTED_EDGE('',*,*,#9145,.F.);
#12536=ORIENTED_EDGE('',*,*,#9155,.F.);
#12537=ORIENTED_EDGE('',*,*,#9156,.F.);
#12538=ORIENTED_EDGE('',*,*,#9157,.F.);
#12539=ORIENTED_EDGE('',*,*,#9158,.F.);
#12540=ORIENTED_EDGE('',*,*,#9150,.T.);
#12541=ORIENTED_EDGE('',*,*,#9147,.T.);
#12542=ORIENTED_EDGE('',*,*,#9144,.T.);
#12543=ORIENTED_EDGE('',*,*,#9155,.T.);
#12544=ORIENTED_EDGE('',*,*,#9159,.F.);
#12545=ORIENTED_EDGE('',*,*,#9151,.F.);
#12546=ORIENTED_EDGE('',*,*,#9160,.T.);
#12547=ORIENTED_EDGE('',*,*,#9158,.T.);
#12548=ORIENTED_EDGE('',*,*,#9161,.F.);
#12549=ORIENTED_EDGE('',*,*,#9152,.F.);
#12550=ORIENTED_EDGE('',*,*,#9159,.T.);
#12551=ORIENTED_EDGE('',*,*,#9157,.T.);
#12552=ORIENTED_EDGE('',*,*,#9162,.F.);
#12553=ORIENTED_EDGE('',*,*,#9153,.F.);
#12554=ORIENTED_EDGE('',*,*,#9161,.T.);
#12555=ORIENTED_EDGE('',*,*,#9156,.T.);
#12556=ORIENTED_EDGE('',*,*,#9160,.F.);
#12557=ORIENTED_EDGE('',*,*,#9154,.F.);
#12558=ORIENTED_EDGE('',*,*,#9162,.T.);
#12559=ORIENTED_EDGE('',*,*,#9163,.F.);
#12560=ORIENTED_EDGE('',*,*,#9164,.F.);
#12561=ORIENTED_EDGE('',*,*,#9165,.T.);
#12562=ORIENTED_EDGE('',*,*,#9166,.T.);
#12563=ORIENTED_EDGE('',*,*,#9167,.F.);
#12564=ORIENTED_EDGE('',*,*,#9166,.F.);
#12565=ORIENTED_EDGE('',*,*,#9168,.T.);
#12566=ORIENTED_EDGE('',*,*,#9169,.T.);
#12567=ORIENTED_EDGE('',*,*,#9170,.F.);
#12568=ORIENTED_EDGE('',*,*,#9169,.F.);
#12569=ORIENTED_EDGE('',*,*,#9171,.T.);
#12570=ORIENTED_EDGE('',*,*,#9172,.T.);
#12571=ORIENTED_EDGE('',*,*,#9173,.F.);
#12572=ORIENTED_EDGE('',*,*,#9172,.F.);
#12573=ORIENTED_EDGE('',*,*,#9174,.T.);
#12574=ORIENTED_EDGE('',*,*,#9164,.T.);
#12575=ORIENTED_EDGE('',*,*,#9165,.F.);
#12576=ORIENTED_EDGE('',*,*,#9174,.F.);
#12577=ORIENTED_EDGE('',*,*,#9171,.F.);
#12578=ORIENTED_EDGE('',*,*,#9168,.F.);
#12579=ORIENTED_EDGE('',*,*,#9163,.T.);
#12580=ORIENTED_EDGE('',*,*,#9167,.T.);
#12581=ORIENTED_EDGE('',*,*,#9170,.T.);
#12582=ORIENTED_EDGE('',*,*,#9173,.T.);
#12583=ORIENTED_EDGE('',*,*,#9175,.F.);
#12584=ORIENTED_EDGE('',*,*,#9176,.F.);
#12585=ORIENTED_EDGE('',*,*,#9177,.T.);
#12586=ORIENTED_EDGE('',*,*,#9178,.T.);
#12587=ORIENTED_EDGE('',*,*,#9179,.F.);
#12588=ORIENTED_EDGE('',*,*,#9178,.F.);
#12589=ORIENTED_EDGE('',*,*,#9180,.T.);
#12590=ORIENTED_EDGE('',*,*,#9181,.T.);
#12591=ORIENTED_EDGE('',*,*,#9182,.F.);
#12592=ORIENTED_EDGE('',*,*,#9181,.F.);
#12593=ORIENTED_EDGE('',*,*,#9183,.T.);
#12594=ORIENTED_EDGE('',*,*,#9184,.T.);
#12595=ORIENTED_EDGE('',*,*,#9185,.F.);
#12596=ORIENTED_EDGE('',*,*,#9184,.F.);
#12597=ORIENTED_EDGE('',*,*,#9186,.T.);
#12598=ORIENTED_EDGE('',*,*,#9176,.T.);
#12599=ORIENTED_EDGE('',*,*,#9177,.F.);
#12600=ORIENTED_EDGE('',*,*,#9186,.F.);
#12601=ORIENTED_EDGE('',*,*,#9183,.F.);
#12602=ORIENTED_EDGE('',*,*,#9180,.F.);
#12603=ORIENTED_EDGE('',*,*,#9175,.T.);
#12604=ORIENTED_EDGE('',*,*,#9179,.T.);
#12605=ORIENTED_EDGE('',*,*,#9182,.T.);
#12606=ORIENTED_EDGE('',*,*,#9185,.T.);
#12607=ORIENTED_EDGE('',*,*,#9187,.F.);
#12608=ORIENTED_EDGE('',*,*,#9188,.F.);
#12609=ORIENTED_EDGE('',*,*,#9189,.T.);
#12610=ORIENTED_EDGE('',*,*,#9190,.T.);
#12611=ORIENTED_EDGE('',*,*,#9191,.F.);
#12612=ORIENTED_EDGE('',*,*,#9192,.F.);
#12613=ORIENTED_EDGE('',*,*,#9193,.T.);
#12614=ORIENTED_EDGE('',*,*,#9188,.T.);
#12615=ORIENTED_EDGE('',*,*,#9194,.F.);
#12616=ORIENTED_EDGE('',*,*,#9195,.F.);
#12617=ORIENTED_EDGE('',*,*,#9196,.T.);
#12618=ORIENTED_EDGE('',*,*,#9192,.T.);
#12619=ORIENTED_EDGE('',*,*,#9197,.F.);
#12620=ORIENTED_EDGE('',*,*,#9190,.F.);
#12621=ORIENTED_EDGE('',*,*,#9198,.T.);
#12622=ORIENTED_EDGE('',*,*,#9195,.T.);
#12623=ORIENTED_EDGE('',*,*,#9189,.F.);
#12624=ORIENTED_EDGE('',*,*,#9193,.F.);
#12625=ORIENTED_EDGE('',*,*,#9196,.F.);
#12626=ORIENTED_EDGE('',*,*,#9198,.F.);
#12627=ORIENTED_EDGE('',*,*,#9187,.T.);
#12628=ORIENTED_EDGE('',*,*,#9197,.T.);
#12629=ORIENTED_EDGE('',*,*,#9194,.T.);
#12630=ORIENTED_EDGE('',*,*,#9191,.T.);
#12631=ORIENTED_EDGE('',*,*,#9199,.F.);
#12632=ORIENTED_EDGE('',*,*,#9200,.F.);
#12633=ORIENTED_EDGE('',*,*,#9201,.T.);
#12634=ORIENTED_EDGE('',*,*,#9202,.T.);
#12635=ORIENTED_EDGE('',*,*,#9203,.F.);
#12636=ORIENTED_EDGE('',*,*,#9204,.F.);
#12637=ORIENTED_EDGE('',*,*,#9205,.T.);
#12638=ORIENTED_EDGE('',*,*,#9200,.T.);
#12639=ORIENTED_EDGE('',*,*,#9206,.F.);
#12640=ORIENTED_EDGE('',*,*,#9207,.F.);
#12641=ORIENTED_EDGE('',*,*,#9208,.T.);
#12642=ORIENTED_EDGE('',*,*,#9204,.T.);
#12643=ORIENTED_EDGE('',*,*,#9209,.F.);
#12644=ORIENTED_EDGE('',*,*,#9202,.F.);
#12645=ORIENTED_EDGE('',*,*,#9210,.T.);
#12646=ORIENTED_EDGE('',*,*,#9207,.T.);
#12647=ORIENTED_EDGE('',*,*,#9201,.F.);
#12648=ORIENTED_EDGE('',*,*,#9205,.F.);
#12649=ORIENTED_EDGE('',*,*,#9208,.F.);
#12650=ORIENTED_EDGE('',*,*,#9210,.F.);
#12651=ORIENTED_EDGE('',*,*,#9199,.T.);
#12652=ORIENTED_EDGE('',*,*,#9209,.T.);
#12653=ORIENTED_EDGE('',*,*,#9206,.T.);
#12654=ORIENTED_EDGE('',*,*,#9203,.T.);
#12655=ORIENTED_EDGE('',*,*,#9211,.T.);
#12656=ORIENTED_EDGE('',*,*,#9212,.F.);
#12657=ORIENTED_EDGE('',*,*,#9213,.F.);
#12658=ORIENTED_EDGE('',*,*,#9214,.T.);
#12659=ORIENTED_EDGE('',*,*,#9215,.T.);
#12660=ORIENTED_EDGE('',*,*,#9214,.F.);
#12661=ORIENTED_EDGE('',*,*,#9216,.F.);
#12662=ORIENTED_EDGE('',*,*,#9217,.T.);
#12663=ORIENTED_EDGE('',*,*,#9218,.T.);
#12664=ORIENTED_EDGE('',*,*,#9217,.F.);
#12665=ORIENTED_EDGE('',*,*,#9219,.F.);
#12666=ORIENTED_EDGE('',*,*,#9220,.T.);
#12667=ORIENTED_EDGE('',*,*,#9221,.T.);
#12668=ORIENTED_EDGE('',*,*,#9220,.F.);
#12669=ORIENTED_EDGE('',*,*,#9222,.F.);
#12670=ORIENTED_EDGE('',*,*,#9212,.T.);
#12671=ORIENTED_EDGE('',*,*,#9213,.T.);
#12672=ORIENTED_EDGE('',*,*,#9222,.T.);
#12673=ORIENTED_EDGE('',*,*,#9219,.T.);
#12674=ORIENTED_EDGE('',*,*,#9216,.T.);
#12675=ORIENTED_EDGE('',*,*,#9211,.F.);
#12676=ORIENTED_EDGE('',*,*,#9215,.F.);
#12677=ORIENTED_EDGE('',*,*,#9218,.F.);
#12678=ORIENTED_EDGE('',*,*,#9221,.F.);
#12679=ORIENTED_EDGE('',*,*,#9223,.T.);
#12680=ORIENTED_EDGE('',*,*,#9224,.T.);
#12681=ORIENTED_EDGE('',*,*,#9225,.F.);
#12682=ORIENTED_EDGE('',*,*,#9224,.F.);
#12683=ORIENTED_EDGE('',*,*,#9226,.T.);
#12684=ORIENTED_EDGE('',*,*,#9227,.T.);
#12685=ORIENTED_EDGE('',*,*,#9228,.F.);
#12686=ORIENTED_EDGE('',*,*,#9227,.F.);
#12687=ORIENTED_EDGE('',*,*,#9229,.T.);
#12688=ORIENTED_EDGE('',*,*,#9230,.T.);
#12689=ORIENTED_EDGE('',*,*,#9231,.F.);
#12690=ORIENTED_EDGE('',*,*,#9230,.F.);
#12691=ORIENTED_EDGE('',*,*,#9232,.T.);
#12692=ORIENTED_EDGE('',*,*,#9233,.T.);
#12693=ORIENTED_EDGE('',*,*,#9234,.F.);
#12694=ORIENTED_EDGE('',*,*,#9233,.F.);
#12695=ORIENTED_EDGE('',*,*,#9235,.T.);
#12696=ORIENTED_EDGE('',*,*,#9236,.T.);
#12697=ORIENTED_EDGE('',*,*,#9237,.T.);
#12698=ORIENTED_EDGE('',*,*,#9238,.T.);
#12699=ORIENTED_EDGE('',*,*,#9232,.F.);
#12700=ORIENTED_EDGE('',*,*,#9229,.F.);
#12701=ORIENTED_EDGE('',*,*,#9226,.F.);
#12702=ORIENTED_EDGE('',*,*,#9223,.F.);
#12703=ORIENTED_EDGE('',*,*,#9239,.F.);
#12704=ORIENTED_EDGE('',*,*,#9240,.F.);
#12705=ORIENTED_EDGE('',*,*,#9241,.F.);
#12706=ORIENTED_EDGE('',*,*,#9242,.F.);
#12707=ORIENTED_EDGE('',*,*,#9231,.T.);
#12708=ORIENTED_EDGE('',*,*,#9225,.T.);
#12709=ORIENTED_EDGE('',*,*,#9228,.T.);
#12710=ORIENTED_EDGE('',*,*,#9234,.T.);
#12711=ORIENTED_EDGE('',*,*,#9239,.T.);
#12712=ORIENTED_EDGE('',*,*,#9243,.F.);
#12713=ORIENTED_EDGE('',*,*,#9235,.F.);
#12714=ORIENTED_EDGE('',*,*,#9244,.T.);
#12715=ORIENTED_EDGE('',*,*,#9242,.T.);
#12716=ORIENTED_EDGE('',*,*,#9245,.F.);
#12717=ORIENTED_EDGE('',*,*,#9236,.F.);
#12718=ORIENTED_EDGE('',*,*,#9243,.T.);
#12719=ORIENTED_EDGE('',*,*,#9241,.T.);
#12720=ORIENTED_EDGE('',*,*,#9246,.F.);
#12721=ORIENTED_EDGE('',*,*,#9237,.F.);
#12722=ORIENTED_EDGE('',*,*,#9245,.T.);
#12723=ORIENTED_EDGE('',*,*,#9240,.T.);
#12724=ORIENTED_EDGE('',*,*,#9244,.F.);
#12725=ORIENTED_EDGE('',*,*,#9238,.F.);
#12726=ORIENTED_EDGE('',*,*,#9246,.T.);
#12727=ORIENTED_EDGE('',*,*,#9247,.F.);
#12728=ORIENTED_EDGE('',*,*,#9248,.T.);
#12729=ORIENTED_EDGE('',*,*,#9249,.T.);
#12730=ORIENTED_EDGE('',*,*,#9248,.F.);
#12731=ORIENTED_EDGE('',*,*,#9250,.F.);
#12732=ORIENTED_EDGE('',*,*,#9251,.T.);
#12733=ORIENTED_EDGE('',*,*,#9252,.T.);
#12734=ORIENTED_EDGE('',*,*,#9251,.F.);
#12735=ORIENTED_EDGE('',*,*,#9253,.F.);
#12736=ORIENTED_EDGE('',*,*,#9254,.T.);
#12737=ORIENTED_EDGE('',*,*,#9255,.T.);
#12738=ORIENTED_EDGE('',*,*,#9254,.F.);
#12739=ORIENTED_EDGE('',*,*,#9256,.F.);
#12740=ORIENTED_EDGE('',*,*,#9257,.T.);
#12741=ORIENTED_EDGE('',*,*,#9258,.T.);
#12742=ORIENTED_EDGE('',*,*,#9257,.F.);
#12743=ORIENTED_EDGE('',*,*,#9259,.F.);
#12744=ORIENTED_EDGE('',*,*,#9260,.T.);
#12745=ORIENTED_EDGE('',*,*,#9261,.T.);
#12746=ORIENTED_EDGE('',*,*,#9260,.F.);
#12747=ORIENTED_EDGE('',*,*,#9262,.F.);
#12748=ORIENTED_EDGE('',*,*,#9263,.T.);
#12749=ORIENTED_EDGE('',*,*,#9264,.T.);
#12750=ORIENTED_EDGE('',*,*,#9263,.F.);
#12751=ORIENTED_EDGE('',*,*,#9265,.F.);
#12752=ORIENTED_EDGE('',*,*,#9266,.F.);
#12753=ORIENTED_EDGE('',*,*,#9267,.T.);
#12754=ORIENTED_EDGE('',*,*,#9268,.T.);
#12755=ORIENTED_EDGE('',*,*,#9269,.F.);
#12756=ORIENTED_EDGE('',*,*,#9270,.F.);
#12757=ORIENTED_EDGE('',*,*,#9271,.T.);
#12758=ORIENTED_EDGE('',*,*,#9266,.T.);
#12759=ORIENTED_EDGE('',*,*,#9272,.F.);
#12760=ORIENTED_EDGE('',*,*,#9273,.F.);
#12761=ORIENTED_EDGE('',*,*,#9274,.T.);
#12762=ORIENTED_EDGE('',*,*,#9270,.T.);
#12763=ORIENTED_EDGE('',*,*,#9275,.F.);
#12764=ORIENTED_EDGE('',*,*,#9268,.F.);
#12765=ORIENTED_EDGE('',*,*,#9276,.T.);
#12766=ORIENTED_EDGE('',*,*,#9273,.T.);
#12767=ORIENTED_EDGE('',*,*,#9267,.F.);
#12768=ORIENTED_EDGE('',*,*,#9271,.F.);
#12769=ORIENTED_EDGE('',*,*,#9274,.F.);
#12770=ORIENTED_EDGE('',*,*,#9276,.F.);
#12771=ORIENTED_EDGE('',*,*,#9247,.T.);
#12772=ORIENTED_EDGE('',*,*,#9250,.T.);
#12773=ORIENTED_EDGE('',*,*,#9253,.T.);
#12774=ORIENTED_EDGE('',*,*,#9256,.T.);
#12775=ORIENTED_EDGE('',*,*,#9259,.T.);
#12776=ORIENTED_EDGE('',*,*,#9262,.T.);
#12777=ORIENTED_EDGE('',*,*,#9265,.T.);
#12778=ORIENTED_EDGE('',*,*,#9275,.T.);
#12779=ORIENTED_EDGE('',*,*,#9272,.T.);
#12780=ORIENTED_EDGE('',*,*,#9269,.T.);
#12781=ORIENTED_EDGE('',*,*,#9249,.F.);
#12782=ORIENTED_EDGE('',*,*,#9252,.F.);
#12783=ORIENTED_EDGE('',*,*,#9255,.F.);
#12784=ORIENTED_EDGE('',*,*,#9258,.F.);
#12785=ORIENTED_EDGE('',*,*,#9261,.F.);
#12786=ORIENTED_EDGE('',*,*,#9264,.F.);
#12787=ORIENTED_EDGE('',*,*,#9277,.T.);
#12788=ORIENTED_EDGE('',*,*,#9278,.F.);
#12789=ORIENTED_EDGE('',*,*,#9279,.F.);
#12790=ORIENTED_EDGE('',*,*,#9280,.T.);
#12791=ORIENTED_EDGE('',*,*,#9281,.T.);
#12792=ORIENTED_EDGE('',*,*,#9282,.F.);
#12793=ORIENTED_EDGE('',*,*,#9283,.F.);
#12794=ORIENTED_EDGE('',*,*,#9278,.T.);
#12795=ORIENTED_EDGE('',*,*,#9284,.T.);
#12796=ORIENTED_EDGE('',*,*,#9285,.F.);
#12797=ORIENTED_EDGE('',*,*,#9286,.F.);
#12798=ORIENTED_EDGE('',*,*,#9282,.T.);
#12799=ORIENTED_EDGE('',*,*,#9287,.T.);
#12800=ORIENTED_EDGE('',*,*,#9288,.F.);
#12801=ORIENTED_EDGE('',*,*,#9289,.F.);
#12802=ORIENTED_EDGE('',*,*,#9285,.T.);
#12803=ORIENTED_EDGE('',*,*,#9290,.T.);
#12804=ORIENTED_EDGE('',*,*,#9291,.F.);
#12805=ORIENTED_EDGE('',*,*,#9292,.F.);
#12806=ORIENTED_EDGE('',*,*,#9288,.T.);
#12807=ORIENTED_EDGE('',*,*,#9293,.T.);
#12808=ORIENTED_EDGE('',*,*,#9294,.F.);
#12809=ORIENTED_EDGE('',*,*,#9295,.F.);
#12810=ORIENTED_EDGE('',*,*,#9291,.T.);
#12811=ORIENTED_EDGE('',*,*,#9296,.T.);
#12812=ORIENTED_EDGE('',*,*,#9280,.F.);
#12813=ORIENTED_EDGE('',*,*,#9297,.F.);
#12814=ORIENTED_EDGE('',*,*,#9294,.T.);
#12815=ORIENTED_EDGE('',*,*,#9279,.T.);
#12816=ORIENTED_EDGE('',*,*,#9283,.T.);
#12817=ORIENTED_EDGE('',*,*,#9286,.T.);
#12818=ORIENTED_EDGE('',*,*,#9289,.T.);
#12819=ORIENTED_EDGE('',*,*,#9292,.T.);
#12820=ORIENTED_EDGE('',*,*,#9295,.T.);
#12821=ORIENTED_EDGE('',*,*,#9297,.T.);
#12822=ORIENTED_EDGE('',*,*,#9277,.F.);
#12823=ORIENTED_EDGE('',*,*,#9296,.F.);
#12824=ORIENTED_EDGE('',*,*,#9293,.F.);
#12825=ORIENTED_EDGE('',*,*,#9290,.F.);
#12826=ORIENTED_EDGE('',*,*,#9287,.F.);
#12827=ORIENTED_EDGE('',*,*,#9284,.F.);
#12828=ORIENTED_EDGE('',*,*,#9281,.F.);
#12829=ORIENTED_EDGE('',*,*,#9298,.T.);
#12830=ORIENTED_EDGE('',*,*,#9299,.F.);
#12831=ORIENTED_EDGE('',*,*,#9300,.F.);
#12832=ORIENTED_EDGE('',*,*,#9301,.T.);
#12833=ORIENTED_EDGE('',*,*,#9302,.T.);
#12834=ORIENTED_EDGE('',*,*,#9303,.F.);
#12835=ORIENTED_EDGE('',*,*,#9304,.F.);
#12836=ORIENTED_EDGE('',*,*,#9299,.T.);
#12837=ORIENTED_EDGE('',*,*,#9305,.T.);
#12838=ORIENTED_EDGE('',*,*,#9306,.F.);
#12839=ORIENTED_EDGE('',*,*,#9307,.F.);
#12840=ORIENTED_EDGE('',*,*,#9303,.T.);
#12841=ORIENTED_EDGE('',*,*,#9308,.T.);
#12842=ORIENTED_EDGE('',*,*,#9309,.F.);
#12843=ORIENTED_EDGE('',*,*,#9310,.F.);
#12844=ORIENTED_EDGE('',*,*,#9306,.T.);
#12845=ORIENTED_EDGE('',*,*,#9311,.T.);
#12846=ORIENTED_EDGE('',*,*,#9312,.F.);
#12847=ORIENTED_EDGE('',*,*,#9313,.F.);
#12848=ORIENTED_EDGE('',*,*,#9309,.T.);
#12849=ORIENTED_EDGE('',*,*,#9314,.T.);
#12850=ORIENTED_EDGE('',*,*,#9315,.F.);
#12851=ORIENTED_EDGE('',*,*,#9316,.F.);
#12852=ORIENTED_EDGE('',*,*,#9312,.T.);
#12853=ORIENTED_EDGE('',*,*,#9317,.T.);
#12854=ORIENTED_EDGE('',*,*,#9301,.F.);
#12855=ORIENTED_EDGE('',*,*,#9318,.F.);
#12856=ORIENTED_EDGE('',*,*,#9315,.T.);
#12857=ORIENTED_EDGE('',*,*,#9300,.T.);
#12858=ORIENTED_EDGE('',*,*,#9304,.T.);
#12859=ORIENTED_EDGE('',*,*,#9307,.T.);
#12860=ORIENTED_EDGE('',*,*,#9310,.T.);
#12861=ORIENTED_EDGE('',*,*,#9313,.T.);
#12862=ORIENTED_EDGE('',*,*,#9316,.T.);
#12863=ORIENTED_EDGE('',*,*,#9318,.T.);
#12864=ORIENTED_EDGE('',*,*,#9298,.F.);
#12865=ORIENTED_EDGE('',*,*,#9317,.F.);
#12866=ORIENTED_EDGE('',*,*,#9314,.F.);
#12867=ORIENTED_EDGE('',*,*,#9311,.F.);
#12868=ORIENTED_EDGE('',*,*,#9308,.F.);
#12869=ORIENTED_EDGE('',*,*,#9305,.F.);
#12870=ORIENTED_EDGE('',*,*,#9302,.F.);
#12871=ORIENTED_EDGE('',*,*,#9319,.T.);
#12872=ORIENTED_EDGE('',*,*,#9320,.F.);
#12873=ORIENTED_EDGE('',*,*,#9321,.F.);
#12874=ORIENTED_EDGE('',*,*,#9322,.T.);
#12875=ORIENTED_EDGE('',*,*,#9323,.T.);
#12876=ORIENTED_EDGE('',*,*,#9324,.F.);
#12877=ORIENTED_EDGE('',*,*,#9325,.F.);
#12878=ORIENTED_EDGE('',*,*,#9320,.T.);
#12879=ORIENTED_EDGE('',*,*,#9326,.T.);
#12880=ORIENTED_EDGE('',*,*,#9327,.F.);
#12881=ORIENTED_EDGE('',*,*,#9328,.F.);
#12882=ORIENTED_EDGE('',*,*,#9324,.T.);
#12883=ORIENTED_EDGE('',*,*,#9329,.T.);
#12884=ORIENTED_EDGE('',*,*,#9330,.F.);
#12885=ORIENTED_EDGE('',*,*,#9331,.F.);
#12886=ORIENTED_EDGE('',*,*,#9327,.T.);
#12887=ORIENTED_EDGE('',*,*,#9332,.T.);
#12888=ORIENTED_EDGE('',*,*,#9333,.F.);
#12889=ORIENTED_EDGE('',*,*,#9334,.F.);
#12890=ORIENTED_EDGE('',*,*,#9330,.T.);
#12891=ORIENTED_EDGE('',*,*,#9335,.T.);
#12892=ORIENTED_EDGE('',*,*,#9336,.F.);
#12893=ORIENTED_EDGE('',*,*,#9337,.F.);
#12894=ORIENTED_EDGE('',*,*,#9333,.T.);
#12895=ORIENTED_EDGE('',*,*,#9338,.T.);
#12896=ORIENTED_EDGE('',*,*,#9322,.F.);
#12897=ORIENTED_EDGE('',*,*,#9339,.F.);
#12898=ORIENTED_EDGE('',*,*,#9336,.T.);
#12899=ORIENTED_EDGE('',*,*,#9321,.T.);
#12900=ORIENTED_EDGE('',*,*,#9325,.T.);
#12901=ORIENTED_EDGE('',*,*,#9328,.T.);
#12902=ORIENTED_EDGE('',*,*,#9331,.T.);
#12903=ORIENTED_EDGE('',*,*,#9334,.T.);
#12904=ORIENTED_EDGE('',*,*,#9337,.T.);
#12905=ORIENTED_EDGE('',*,*,#9339,.T.);
#12906=ORIENTED_EDGE('',*,*,#9319,.F.);
#12907=ORIENTED_EDGE('',*,*,#9338,.F.);
#12908=ORIENTED_EDGE('',*,*,#9335,.F.);
#12909=ORIENTED_EDGE('',*,*,#9332,.F.);
#12910=ORIENTED_EDGE('',*,*,#9329,.F.);
#12911=ORIENTED_EDGE('',*,*,#9326,.F.);
#12912=ORIENTED_EDGE('',*,*,#9323,.F.);
#12913=ORIENTED_EDGE('',*,*,#9340,.F.);
#12914=ORIENTED_EDGE('',*,*,#9341,.F.);
#12915=ORIENTED_EDGE('',*,*,#9342,.T.);
#12916=ORIENTED_EDGE('',*,*,#9343,.T.);
#12917=ORIENTED_EDGE('',*,*,#9344,.F.);
#12918=ORIENTED_EDGE('',*,*,#9345,.F.);
#12919=ORIENTED_EDGE('',*,*,#9346,.T.);
#12920=ORIENTED_EDGE('',*,*,#9341,.T.);
#12921=ORIENTED_EDGE('',*,*,#9347,.F.);
#12922=ORIENTED_EDGE('',*,*,#9348,.F.);
#12923=ORIENTED_EDGE('',*,*,#9349,.T.);
#12924=ORIENTED_EDGE('',*,*,#9345,.T.);
#12925=ORIENTED_EDGE('',*,*,#9350,.F.);
#12926=ORIENTED_EDGE('',*,*,#9351,.F.);
#12927=ORIENTED_EDGE('',*,*,#9352,.T.);
#12928=ORIENTED_EDGE('',*,*,#9348,.T.);
#12929=ORIENTED_EDGE('',*,*,#9353,.F.);
#12930=ORIENTED_EDGE('',*,*,#9354,.F.);
#12931=ORIENTED_EDGE('',*,*,#9355,.T.);
#12932=ORIENTED_EDGE('',*,*,#9351,.T.);
#12933=ORIENTED_EDGE('',*,*,#9356,.F.);
#12934=ORIENTED_EDGE('',*,*,#9357,.F.);
#12935=ORIENTED_EDGE('',*,*,#9358,.T.);
#12936=ORIENTED_EDGE('',*,*,#9354,.T.);
#12937=ORIENTED_EDGE('',*,*,#9359,.F.);
#12938=ORIENTED_EDGE('',*,*,#9343,.F.);
#12939=ORIENTED_EDGE('',*,*,#9360,.T.);
#12940=ORIENTED_EDGE('',*,*,#9357,.T.);
#12941=ORIENTED_EDGE('',*,*,#9342,.F.);
#12942=ORIENTED_EDGE('',*,*,#9346,.F.);
#12943=ORIENTED_EDGE('',*,*,#9349,.F.);
#12944=ORIENTED_EDGE('',*,*,#9352,.F.);
#12945=ORIENTED_EDGE('',*,*,#9355,.F.);
#12946=ORIENTED_EDGE('',*,*,#9358,.F.);
#12947=ORIENTED_EDGE('',*,*,#9360,.F.);
#12948=ORIENTED_EDGE('',*,*,#9340,.T.);
#12949=ORIENTED_EDGE('',*,*,#9359,.T.);
#12950=ORIENTED_EDGE('',*,*,#9356,.T.);
#12951=ORIENTED_EDGE('',*,*,#9353,.T.);
#12952=ORIENTED_EDGE('',*,*,#9350,.T.);
#12953=ORIENTED_EDGE('',*,*,#9347,.T.);
#12954=ORIENTED_EDGE('',*,*,#9344,.T.);
#12955=ORIENTED_EDGE('',*,*,#9361,.F.);
#12956=ORIENTED_EDGE('',*,*,#9362,.F.);
#12957=ORIENTED_EDGE('',*,*,#9363,.T.);
#12958=ORIENTED_EDGE('',*,*,#9364,.T.);
#12959=ORIENTED_EDGE('',*,*,#9365,.F.);
#12960=ORIENTED_EDGE('',*,*,#9366,.F.);
#12961=ORIENTED_EDGE('',*,*,#9367,.T.);
#12962=ORIENTED_EDGE('',*,*,#9362,.T.);
#12963=ORIENTED_EDGE('',*,*,#9368,.F.);
#12964=ORIENTED_EDGE('',*,*,#9369,.F.);
#12965=ORIENTED_EDGE('',*,*,#9370,.T.);
#12966=ORIENTED_EDGE('',*,*,#9366,.T.);
#12967=ORIENTED_EDGE('',*,*,#9371,.F.);
#12968=ORIENTED_EDGE('',*,*,#9372,.F.);
#12969=ORIENTED_EDGE('',*,*,#9373,.T.);
#12970=ORIENTED_EDGE('',*,*,#9369,.T.);
#12971=ORIENTED_EDGE('',*,*,#9374,.F.);
#12972=ORIENTED_EDGE('',*,*,#9375,.F.);
#12973=ORIENTED_EDGE('',*,*,#9376,.T.);
#12974=ORIENTED_EDGE('',*,*,#9372,.T.);
#12975=ORIENTED_EDGE('',*,*,#9377,.F.);
#12976=ORIENTED_EDGE('',*,*,#9378,.F.);
#12977=ORIENTED_EDGE('',*,*,#9379,.T.);
#12978=ORIENTED_EDGE('',*,*,#9375,.T.);
#12979=ORIENTED_EDGE('',*,*,#9380,.F.);
#12980=ORIENTED_EDGE('',*,*,#9364,.F.);
#12981=ORIENTED_EDGE('',*,*,#9381,.T.);
#12982=ORIENTED_EDGE('',*,*,#9378,.T.);
#12983=ORIENTED_EDGE('',*,*,#9363,.F.);
#12984=ORIENTED_EDGE('',*,*,#9367,.F.);
#12985=ORIENTED_EDGE('',*,*,#9370,.F.);
#12986=ORIENTED_EDGE('',*,*,#9373,.F.);
#12987=ORIENTED_EDGE('',*,*,#9376,.F.);
#12988=ORIENTED_EDGE('',*,*,#9379,.F.);
#12989=ORIENTED_EDGE('',*,*,#9381,.F.);
#12990=ORIENTED_EDGE('',*,*,#9361,.T.);
#12991=ORIENTED_EDGE('',*,*,#9380,.T.);
#12992=ORIENTED_EDGE('',*,*,#9377,.T.);
#12993=ORIENTED_EDGE('',*,*,#9374,.T.);
#12994=ORIENTED_EDGE('',*,*,#9371,.T.);
#12995=ORIENTED_EDGE('',*,*,#9368,.T.);
#12996=ORIENTED_EDGE('',*,*,#9365,.T.);
#12997=ORIENTED_EDGE('',*,*,#9382,.F.);
#12998=ORIENTED_EDGE('',*,*,#9383,.F.);
#12999=ORIENTED_EDGE('',*,*,#9384,.T.);
#13000=ORIENTED_EDGE('',*,*,#9385,.T.);
#13001=ORIENTED_EDGE('',*,*,#9386,.F.);
#13002=ORIENTED_EDGE('',*,*,#9387,.F.);
#13003=ORIENTED_EDGE('',*,*,#9388,.T.);
#13004=ORIENTED_EDGE('',*,*,#9383,.T.);
#13005=ORIENTED_EDGE('',*,*,#9389,.F.);
#13006=ORIENTED_EDGE('',*,*,#9390,.F.);
#13007=ORIENTED_EDGE('',*,*,#9391,.T.);
#13008=ORIENTED_EDGE('',*,*,#9387,.T.);
#13009=ORIENTED_EDGE('',*,*,#9392,.F.);
#13010=ORIENTED_EDGE('',*,*,#9393,.F.);
#13011=ORIENTED_EDGE('',*,*,#9394,.T.);
#13012=ORIENTED_EDGE('',*,*,#9390,.T.);
#13013=ORIENTED_EDGE('',*,*,#9395,.F.);
#13014=ORIENTED_EDGE('',*,*,#9396,.F.);
#13015=ORIENTED_EDGE('',*,*,#9397,.T.);
#13016=ORIENTED_EDGE('',*,*,#9393,.T.);
#13017=ORIENTED_EDGE('',*,*,#9398,.F.);
#13018=ORIENTED_EDGE('',*,*,#9399,.F.);
#13019=ORIENTED_EDGE('',*,*,#9400,.T.);
#13020=ORIENTED_EDGE('',*,*,#9396,.T.);
#13021=ORIENTED_EDGE('',*,*,#9401,.F.);
#13022=ORIENTED_EDGE('',*,*,#9385,.F.);
#13023=ORIENTED_EDGE('',*,*,#9402,.T.);
#13024=ORIENTED_EDGE('',*,*,#9399,.T.);
#13025=ORIENTED_EDGE('',*,*,#9384,.F.);
#13026=ORIENTED_EDGE('',*,*,#9388,.F.);
#13027=ORIENTED_EDGE('',*,*,#9391,.F.);
#13028=ORIENTED_EDGE('',*,*,#9394,.F.);
#13029=ORIENTED_EDGE('',*,*,#9397,.F.);
#13030=ORIENTED_EDGE('',*,*,#9400,.F.);
#13031=ORIENTED_EDGE('',*,*,#9402,.F.);
#13032=ORIENTED_EDGE('',*,*,#9382,.T.);
#13033=ORIENTED_EDGE('',*,*,#9401,.T.);
#13034=ORIENTED_EDGE('',*,*,#9398,.T.);
#13035=ORIENTED_EDGE('',*,*,#9395,.T.);
#13036=ORIENTED_EDGE('',*,*,#9392,.T.);
#13037=ORIENTED_EDGE('',*,*,#9389,.T.);
#13038=ORIENTED_EDGE('',*,*,#9386,.T.);
#13039=ORIENTED_EDGE('',*,*,#9403,.T.);
#13040=ORIENTED_EDGE('',*,*,#9404,.F.);
#13041=ORIENTED_EDGE('',*,*,#9405,.F.);
#13042=ORIENTED_EDGE('',*,*,#9406,.T.);
#13043=ORIENTED_EDGE('',*,*,#9407,.T.);
#13044=ORIENTED_EDGE('',*,*,#9406,.F.);
#13045=ORIENTED_EDGE('',*,*,#9408,.F.);
#13046=ORIENTED_EDGE('',*,*,#9409,.T.);
#13047=ORIENTED_EDGE('',*,*,#9410,.T.);
#13048=ORIENTED_EDGE('',*,*,#9409,.F.);
#13049=ORIENTED_EDGE('',*,*,#9411,.F.);
#13050=ORIENTED_EDGE('',*,*,#9412,.T.);
#13051=ORIENTED_EDGE('',*,*,#9413,.T.);
#13052=ORIENTED_EDGE('',*,*,#9412,.F.);
#13053=ORIENTED_EDGE('',*,*,#9414,.F.);
#13054=ORIENTED_EDGE('',*,*,#9415,.T.);
#13055=ORIENTED_EDGE('',*,*,#9416,.T.);
#13056=ORIENTED_EDGE('',*,*,#9415,.F.);
#13057=ORIENTED_EDGE('',*,*,#9417,.F.);
#13058=ORIENTED_EDGE('',*,*,#9418,.T.);
#13059=ORIENTED_EDGE('',*,*,#9419,.T.);
#13060=ORIENTED_EDGE('',*,*,#9418,.F.);
#13061=ORIENTED_EDGE('',*,*,#9420,.F.);
#13062=ORIENTED_EDGE('',*,*,#9421,.T.);
#13063=ORIENTED_EDGE('',*,*,#9422,.T.);
#13064=ORIENTED_EDGE('',*,*,#9421,.F.);
#13065=ORIENTED_EDGE('',*,*,#9423,.F.);
#13066=ORIENTED_EDGE('',*,*,#9404,.T.);
#13067=ORIENTED_EDGE('',*,*,#9405,.T.);
#13068=ORIENTED_EDGE('',*,*,#9423,.T.);
#13069=ORIENTED_EDGE('',*,*,#9420,.T.);
#13070=ORIENTED_EDGE('',*,*,#9417,.T.);
#13071=ORIENTED_EDGE('',*,*,#9414,.T.);
#13072=ORIENTED_EDGE('',*,*,#9411,.T.);
#13073=ORIENTED_EDGE('',*,*,#9408,.T.);
#13074=ORIENTED_EDGE('',*,*,#9403,.F.);
#13075=ORIENTED_EDGE('',*,*,#9407,.F.);
#13076=ORIENTED_EDGE('',*,*,#9410,.F.);
#13077=ORIENTED_EDGE('',*,*,#9413,.F.);
#13078=ORIENTED_EDGE('',*,*,#9416,.F.);
#13079=ORIENTED_EDGE('',*,*,#9419,.F.);
#13080=ORIENTED_EDGE('',*,*,#9422,.F.);
#13081=ORIENTED_EDGE('',*,*,#9424,.T.);
#13082=ORIENTED_EDGE('',*,*,#9425,.F.);
#13083=ORIENTED_EDGE('',*,*,#9426,.F.);
#13084=ORIENTED_EDGE('',*,*,#9427,.T.);
#13085=ORIENTED_EDGE('',*,*,#9428,.T.);
#13086=ORIENTED_EDGE('',*,*,#9427,.F.);
#13087=ORIENTED_EDGE('',*,*,#9429,.F.);
#13088=ORIENTED_EDGE('',*,*,#9430,.T.);
#13089=ORIENTED_EDGE('',*,*,#9431,.T.);
#13090=ORIENTED_EDGE('',*,*,#9430,.F.);
#13091=ORIENTED_EDGE('',*,*,#9432,.F.);
#13092=ORIENTED_EDGE('',*,*,#9433,.T.);
#13093=ORIENTED_EDGE('',*,*,#9434,.T.);
#13094=ORIENTED_EDGE('',*,*,#9433,.F.);
#13095=ORIENTED_EDGE('',*,*,#9435,.F.);
#13096=ORIENTED_EDGE('',*,*,#9436,.T.);
#13097=ORIENTED_EDGE('',*,*,#9437,.T.);
#13098=ORIENTED_EDGE('',*,*,#9436,.F.);
#13099=ORIENTED_EDGE('',*,*,#9438,.F.);
#13100=ORIENTED_EDGE('',*,*,#9439,.T.);
#13101=ORIENTED_EDGE('',*,*,#9440,.T.);
#13102=ORIENTED_EDGE('',*,*,#9439,.F.);
#13103=ORIENTED_EDGE('',*,*,#9441,.F.);
#13104=ORIENTED_EDGE('',*,*,#9442,.T.);
#13105=ORIENTED_EDGE('',*,*,#9443,.T.);
#13106=ORIENTED_EDGE('',*,*,#9442,.F.);
#13107=ORIENTED_EDGE('',*,*,#9444,.F.);
#13108=ORIENTED_EDGE('',*,*,#9425,.T.);
#13109=ORIENTED_EDGE('',*,*,#9426,.T.);
#13110=ORIENTED_EDGE('',*,*,#9444,.T.);
#13111=ORIENTED_EDGE('',*,*,#9441,.T.);
#13112=ORIENTED_EDGE('',*,*,#9438,.T.);
#13113=ORIENTED_EDGE('',*,*,#9435,.T.);
#13114=ORIENTED_EDGE('',*,*,#9432,.T.);
#13115=ORIENTED_EDGE('',*,*,#9429,.T.);
#13116=ORIENTED_EDGE('',*,*,#9424,.F.);
#13117=ORIENTED_EDGE('',*,*,#9428,.F.);
#13118=ORIENTED_EDGE('',*,*,#9431,.F.);
#13119=ORIENTED_EDGE('',*,*,#9434,.F.);
#13120=ORIENTED_EDGE('',*,*,#9437,.F.);
#13121=ORIENTED_EDGE('',*,*,#9440,.F.);
#13122=ORIENTED_EDGE('',*,*,#9443,.F.);
#13123=ORIENTED_EDGE('',*,*,#9445,.F.);
#13124=ORIENTED_EDGE('',*,*,#9446,.F.);
#13125=ORIENTED_EDGE('',*,*,#9447,.T.);
#13126=ORIENTED_EDGE('',*,*,#9448,.T.);
#13127=ORIENTED_EDGE('',*,*,#9449,.F.);
#13128=ORIENTED_EDGE('',*,*,#9448,.F.);
#13129=ORIENTED_EDGE('',*,*,#9450,.T.);
#13130=ORIENTED_EDGE('',*,*,#9451,.T.);
#13131=ORIENTED_EDGE('',*,*,#9452,.F.);
#13132=ORIENTED_EDGE('',*,*,#9451,.F.);
#13133=ORIENTED_EDGE('',*,*,#9453,.T.);
#13134=ORIENTED_EDGE('',*,*,#9454,.T.);
#13135=ORIENTED_EDGE('',*,*,#9455,.F.);
#13136=ORIENTED_EDGE('',*,*,#9454,.F.);
#13137=ORIENTED_EDGE('',*,*,#9456,.T.);
#13138=ORIENTED_EDGE('',*,*,#9457,.T.);
#13139=ORIENTED_EDGE('',*,*,#9458,.F.);
#13140=ORIENTED_EDGE('',*,*,#9457,.F.);
#13141=ORIENTED_EDGE('',*,*,#9459,.T.);
#13142=ORIENTED_EDGE('',*,*,#9460,.T.);
#13143=ORIENTED_EDGE('',*,*,#9461,.F.);
#13144=ORIENTED_EDGE('',*,*,#9460,.F.);
#13145=ORIENTED_EDGE('',*,*,#9462,.T.);
#13146=ORIENTED_EDGE('',*,*,#9463,.T.);
#13147=ORIENTED_EDGE('',*,*,#9464,.F.);
#13148=ORIENTED_EDGE('',*,*,#9463,.F.);
#13149=ORIENTED_EDGE('',*,*,#9465,.T.);
#13150=ORIENTED_EDGE('',*,*,#9446,.T.);
#13151=ORIENTED_EDGE('',*,*,#9447,.F.);
#13152=ORIENTED_EDGE('',*,*,#9465,.F.);
#13153=ORIENTED_EDGE('',*,*,#9462,.F.);
#13154=ORIENTED_EDGE('',*,*,#9459,.F.);
#13155=ORIENTED_EDGE('',*,*,#9456,.F.);
#13156=ORIENTED_EDGE('',*,*,#9453,.F.);
#13157=ORIENTED_EDGE('',*,*,#9450,.F.);
#13158=ORIENTED_EDGE('',*,*,#9445,.T.);
#13159=ORIENTED_EDGE('',*,*,#9449,.T.);
#13160=ORIENTED_EDGE('',*,*,#9452,.T.);
#13161=ORIENTED_EDGE('',*,*,#9455,.T.);
#13162=ORIENTED_EDGE('',*,*,#9458,.T.);
#13163=ORIENTED_EDGE('',*,*,#9461,.T.);
#13164=ORIENTED_EDGE('',*,*,#9464,.T.);
#13165=ORIENTED_EDGE('',*,*,#9466,.F.);
#13166=ORIENTED_EDGE('',*,*,#9467,.F.);
#13167=ORIENTED_EDGE('',*,*,#9468,.T.);
#13168=ORIENTED_EDGE('',*,*,#9469,.T.);
#13169=ORIENTED_EDGE('',*,*,#9470,.F.);
#13170=ORIENTED_EDGE('',*,*,#9469,.F.);
#13171=ORIENTED_EDGE('',*,*,#9471,.T.);
#13172=ORIENTED_EDGE('',*,*,#9472,.T.);
#13173=ORIENTED_EDGE('',*,*,#9473,.F.);
#13174=ORIENTED_EDGE('',*,*,#9472,.F.);
#13175=ORIENTED_EDGE('',*,*,#9474,.T.);
#13176=ORIENTED_EDGE('',*,*,#9475,.T.);
#13177=ORIENTED_EDGE('',*,*,#9476,.F.);
#13178=ORIENTED_EDGE('',*,*,#9475,.F.);
#13179=ORIENTED_EDGE('',*,*,#9477,.T.);
#13180=ORIENTED_EDGE('',*,*,#9478,.T.);
#13181=ORIENTED_EDGE('',*,*,#9479,.F.);
#13182=ORIENTED_EDGE('',*,*,#9478,.F.);
#13183=ORIENTED_EDGE('',*,*,#9480,.T.);
#13184=ORIENTED_EDGE('',*,*,#9481,.T.);
#13185=ORIENTED_EDGE('',*,*,#9482,.F.);
#13186=ORIENTED_EDGE('',*,*,#9481,.F.);
#13187=ORIENTED_EDGE('',*,*,#9483,.T.);
#13188=ORIENTED_EDGE('',*,*,#9484,.T.);
#13189=ORIENTED_EDGE('',*,*,#9485,.F.);
#13190=ORIENTED_EDGE('',*,*,#9484,.F.);
#13191=ORIENTED_EDGE('',*,*,#9486,.T.);
#13192=ORIENTED_EDGE('',*,*,#9467,.T.);
#13193=ORIENTED_EDGE('',*,*,#9468,.F.);
#13194=ORIENTED_EDGE('',*,*,#9486,.F.);
#13195=ORIENTED_EDGE('',*,*,#9483,.F.);
#13196=ORIENTED_EDGE('',*,*,#9480,.F.);
#13197=ORIENTED_EDGE('',*,*,#9477,.F.);
#13198=ORIENTED_EDGE('',*,*,#9474,.F.);
#13199=ORIENTED_EDGE('',*,*,#9471,.F.);
#13200=ORIENTED_EDGE('',*,*,#9466,.T.);
#13201=ORIENTED_EDGE('',*,*,#9470,.T.);
#13202=ORIENTED_EDGE('',*,*,#9473,.T.);
#13203=ORIENTED_EDGE('',*,*,#9476,.T.);
#13204=ORIENTED_EDGE('',*,*,#9479,.T.);
#13205=ORIENTED_EDGE('',*,*,#9482,.T.);
#13206=ORIENTED_EDGE('',*,*,#9485,.T.);
#13207=ORIENTED_EDGE('',*,*,#9487,.F.);
#13208=ORIENTED_EDGE('',*,*,#9488,.F.);
#13209=ORIENTED_EDGE('',*,*,#9489,.T.);
#13210=ORIENTED_EDGE('',*,*,#9490,.T.);
#13211=ORIENTED_EDGE('',*,*,#9491,.F.);
#13212=ORIENTED_EDGE('',*,*,#9490,.F.);
#13213=ORIENTED_EDGE('',*,*,#9492,.T.);
#13214=ORIENTED_EDGE('',*,*,#9493,.T.);
#13215=ORIENTED_EDGE('',*,*,#9494,.F.);
#13216=ORIENTED_EDGE('',*,*,#9493,.F.);
#13217=ORIENTED_EDGE('',*,*,#9495,.T.);
#13218=ORIENTED_EDGE('',*,*,#9496,.T.);
#13219=ORIENTED_EDGE('',*,*,#9497,.F.);
#13220=ORIENTED_EDGE('',*,*,#9496,.F.);
#13221=ORIENTED_EDGE('',*,*,#9498,.T.);
#13222=ORIENTED_EDGE('',*,*,#9499,.T.);
#13223=ORIENTED_EDGE('',*,*,#9500,.F.);
#13224=ORIENTED_EDGE('',*,*,#9499,.F.);
#13225=ORIENTED_EDGE('',*,*,#9501,.T.);
#13226=ORIENTED_EDGE('',*,*,#9502,.T.);
#13227=ORIENTED_EDGE('',*,*,#9503,.F.);
#13228=ORIENTED_EDGE('',*,*,#9502,.F.);
#13229=ORIENTED_EDGE('',*,*,#9504,.T.);
#13230=ORIENTED_EDGE('',*,*,#9505,.T.);
#13231=ORIENTED_EDGE('',*,*,#9506,.F.);
#13232=ORIENTED_EDGE('',*,*,#9505,.F.);
#13233=ORIENTED_EDGE('',*,*,#9507,.T.);
#13234=ORIENTED_EDGE('',*,*,#9488,.T.);
#13235=ORIENTED_EDGE('',*,*,#9489,.F.);
#13236=ORIENTED_EDGE('',*,*,#9507,.F.);
#13237=ORIENTED_EDGE('',*,*,#9504,.F.);
#13238=ORIENTED_EDGE('',*,*,#9501,.F.);
#13239=ORIENTED_EDGE('',*,*,#9498,.F.);
#13240=ORIENTED_EDGE('',*,*,#9495,.F.);
#13241=ORIENTED_EDGE('',*,*,#9492,.F.);
#13242=ORIENTED_EDGE('',*,*,#9487,.T.);
#13243=ORIENTED_EDGE('',*,*,#9491,.T.);
#13244=ORIENTED_EDGE('',*,*,#9494,.T.);
#13245=ORIENTED_EDGE('',*,*,#9497,.T.);
#13246=ORIENTED_EDGE('',*,*,#9500,.T.);
#13247=ORIENTED_EDGE('',*,*,#9503,.T.);
#13248=ORIENTED_EDGE('',*,*,#9506,.T.);
#13249=ORIENTED_EDGE('',*,*,#9508,.F.);
#13250=ORIENTED_EDGE('',*,*,#9509,.T.);
#13251=ORIENTED_EDGE('',*,*,#9510,.T.);
#13252=ORIENTED_EDGE('',*,*,#9509,.F.);
#13253=ORIENTED_EDGE('',*,*,#9511,.F.);
#13254=ORIENTED_EDGE('',*,*,#9512,.T.);
#13255=ORIENTED_EDGE('',*,*,#9513,.T.);
#13256=ORIENTED_EDGE('',*,*,#9512,.F.);
#13257=ORIENTED_EDGE('',*,*,#9514,.F.);
#13258=ORIENTED_EDGE('',*,*,#9515,.T.);
#13259=ORIENTED_EDGE('',*,*,#9516,.T.);
#13260=ORIENTED_EDGE('',*,*,#9515,.F.);
#13261=ORIENTED_EDGE('',*,*,#9517,.F.);
#13262=ORIENTED_EDGE('',*,*,#9518,.T.);
#13263=ORIENTED_EDGE('',*,*,#9519,.T.);
#13264=ORIENTED_EDGE('',*,*,#9518,.F.);
#13265=ORIENTED_EDGE('',*,*,#9520,.F.);
#13266=ORIENTED_EDGE('',*,*,#9521,.F.);
#13267=ORIENTED_EDGE('',*,*,#9522,.F.);
#13268=ORIENTED_EDGE('',*,*,#9523,.F.);
#13269=ORIENTED_EDGE('',*,*,#9517,.T.);
#13270=ORIENTED_EDGE('',*,*,#9514,.T.);
#13271=ORIENTED_EDGE('',*,*,#9511,.T.);
#13272=ORIENTED_EDGE('',*,*,#9508,.T.);
#13273=ORIENTED_EDGE('',*,*,#9524,.T.);
#13274=ORIENTED_EDGE('',*,*,#9525,.T.);
#13275=ORIENTED_EDGE('',*,*,#9526,.T.);
#13276=ORIENTED_EDGE('',*,*,#9527,.T.);
#13277=ORIENTED_EDGE('',*,*,#9516,.F.);
#13278=ORIENTED_EDGE('',*,*,#9510,.F.);
#13279=ORIENTED_EDGE('',*,*,#9513,.F.);
#13280=ORIENTED_EDGE('',*,*,#9519,.F.);
#13281=ORIENTED_EDGE('',*,*,#9524,.F.);
#13282=ORIENTED_EDGE('',*,*,#9528,.F.);
#13283=ORIENTED_EDGE('',*,*,#9520,.T.);
#13284=ORIENTED_EDGE('',*,*,#9529,.T.);
#13285=ORIENTED_EDGE('',*,*,#9525,.F.);
#13286=ORIENTED_EDGE('',*,*,#9529,.F.);
#13287=ORIENTED_EDGE('',*,*,#9523,.T.);
#13288=ORIENTED_EDGE('',*,*,#9530,.T.);
#13289=ORIENTED_EDGE('',*,*,#9526,.F.);
#13290=ORIENTED_EDGE('',*,*,#9530,.F.);
#13291=ORIENTED_EDGE('',*,*,#9522,.T.);
#13292=ORIENTED_EDGE('',*,*,#9531,.T.);
#13293=ORIENTED_EDGE('',*,*,#9527,.F.);
#13294=ORIENTED_EDGE('',*,*,#9531,.F.);
#13295=ORIENTED_EDGE('',*,*,#9521,.T.);
#13296=ORIENTED_EDGE('',*,*,#9528,.T.);
#13297=ORIENTED_EDGE('',*,*,#9532,.T.);
#13298=ORIENTED_EDGE('',*,*,#9533,.F.);
#13299=ORIENTED_EDGE('',*,*,#9534,.F.);
#13300=ORIENTED_EDGE('',*,*,#9535,.T.);
#13301=ORIENTED_EDGE('',*,*,#9536,.T.);
#13302=ORIENTED_EDGE('',*,*,#9537,.F.);
#13303=ORIENTED_EDGE('',*,*,#9538,.F.);
#13304=ORIENTED_EDGE('',*,*,#9533,.T.);
#13305=ORIENTED_EDGE('',*,*,#9539,.T.);
#13306=ORIENTED_EDGE('',*,*,#9540,.F.);
#13307=ORIENTED_EDGE('',*,*,#9541,.F.);
#13308=ORIENTED_EDGE('',*,*,#9537,.T.);
#13309=ORIENTED_EDGE('',*,*,#9542,.T.);
#13310=ORIENTED_EDGE('',*,*,#9535,.F.);
#13311=ORIENTED_EDGE('',*,*,#9543,.F.);
#13312=ORIENTED_EDGE('',*,*,#9540,.T.);
#13313=ORIENTED_EDGE('',*,*,#9534,.T.);
#13314=ORIENTED_EDGE('',*,*,#9538,.T.);
#13315=ORIENTED_EDGE('',*,*,#9541,.T.);
#13316=ORIENTED_EDGE('',*,*,#9543,.T.);
#13317=ORIENTED_EDGE('',*,*,#9532,.F.);
#13318=ORIENTED_EDGE('',*,*,#9542,.F.);
#13319=ORIENTED_EDGE('',*,*,#9539,.F.);
#13320=ORIENTED_EDGE('',*,*,#9536,.F.);
#13321=ORIENTED_EDGE('',*,*,#9544,.T.);
#13322=ORIENTED_EDGE('',*,*,#9545,.F.);
#13323=ORIENTED_EDGE('',*,*,#9546,.F.);
#13324=ORIENTED_EDGE('',*,*,#9547,.T.);
#13325=ORIENTED_EDGE('',*,*,#9548,.T.);
#13326=ORIENTED_EDGE('',*,*,#9549,.F.);
#13327=ORIENTED_EDGE('',*,*,#9550,.F.);
#13328=ORIENTED_EDGE('',*,*,#9545,.T.);
#13329=ORIENTED_EDGE('',*,*,#9551,.T.);
#13330=ORIENTED_EDGE('',*,*,#9552,.F.);
#13331=ORIENTED_EDGE('',*,*,#9553,.F.);
#13332=ORIENTED_EDGE('',*,*,#9549,.T.);
#13333=ORIENTED_EDGE('',*,*,#9554,.T.);
#13334=ORIENTED_EDGE('',*,*,#9547,.F.);
#13335=ORIENTED_EDGE('',*,*,#9555,.F.);
#13336=ORIENTED_EDGE('',*,*,#9552,.T.);
#13337=ORIENTED_EDGE('',*,*,#9546,.T.);
#13338=ORIENTED_EDGE('',*,*,#9550,.T.);
#13339=ORIENTED_EDGE('',*,*,#9553,.T.);
#13340=ORIENTED_EDGE('',*,*,#9555,.T.);
#13341=ORIENTED_EDGE('',*,*,#9544,.F.);
#13342=ORIENTED_EDGE('',*,*,#9554,.F.);
#13343=ORIENTED_EDGE('',*,*,#9551,.F.);
#13344=ORIENTED_EDGE('',*,*,#9548,.F.);
#13345=ORIENTED_EDGE('',*,*,#9556,.T.);
#13346=ORIENTED_EDGE('',*,*,#9557,.F.);
#13347=ORIENTED_EDGE('',*,*,#9558,.F.);
#13348=ORIENTED_EDGE('',*,*,#9559,.T.);
#13349=ORIENTED_EDGE('',*,*,#9560,.T.);
#13350=ORIENTED_EDGE('',*,*,#9561,.F.);
#13351=ORIENTED_EDGE('',*,*,#9562,.F.);
#13352=ORIENTED_EDGE('',*,*,#9557,.T.);
#13353=ORIENTED_EDGE('',*,*,#9563,.T.);
#13354=ORIENTED_EDGE('',*,*,#9564,.F.);
#13355=ORIENTED_EDGE('',*,*,#9565,.F.);
#13356=ORIENTED_EDGE('',*,*,#9561,.T.);
#13357=ORIENTED_EDGE('',*,*,#9566,.T.);
#13358=ORIENTED_EDGE('',*,*,#9559,.F.);
#13359=ORIENTED_EDGE('',*,*,#9567,.F.);
#13360=ORIENTED_EDGE('',*,*,#9564,.T.);
#13361=ORIENTED_EDGE('',*,*,#9558,.T.);
#13362=ORIENTED_EDGE('',*,*,#9562,.T.);
#13363=ORIENTED_EDGE('',*,*,#9565,.T.);
#13364=ORIENTED_EDGE('',*,*,#9567,.T.);
#13365=ORIENTED_EDGE('',*,*,#9556,.F.);
#13366=ORIENTED_EDGE('',*,*,#9566,.F.);
#13367=ORIENTED_EDGE('',*,*,#9563,.F.);
#13368=ORIENTED_EDGE('',*,*,#9560,.F.);
#13369=ORIENTED_EDGE('',*,*,#9568,.T.);
#13370=ORIENTED_EDGE('',*,*,#9569,.F.);
#13371=ORIENTED_EDGE('',*,*,#9570,.F.);
#13372=ORIENTED_EDGE('',*,*,#9571,.T.);
#13373=ORIENTED_EDGE('',*,*,#9572,.T.);
#13374=ORIENTED_EDGE('',*,*,#9573,.F.);
#13375=ORIENTED_EDGE('',*,*,#9574,.F.);
#13376=ORIENTED_EDGE('',*,*,#9569,.T.);
#13377=ORIENTED_EDGE('',*,*,#9575,.T.);
#13378=ORIENTED_EDGE('',*,*,#9576,.F.);
#13379=ORIENTED_EDGE('',*,*,#9577,.F.);
#13380=ORIENTED_EDGE('',*,*,#9573,.T.);
#13381=ORIENTED_EDGE('',*,*,#9578,.T.);
#13382=ORIENTED_EDGE('',*,*,#9571,.F.);
#13383=ORIENTED_EDGE('',*,*,#9579,.F.);
#13384=ORIENTED_EDGE('',*,*,#9576,.T.);
#13385=ORIENTED_EDGE('',*,*,#9570,.T.);
#13386=ORIENTED_EDGE('',*,*,#9574,.T.);
#13387=ORIENTED_EDGE('',*,*,#9577,.T.);
#13388=ORIENTED_EDGE('',*,*,#9579,.T.);
#13389=ORIENTED_EDGE('',*,*,#9568,.F.);
#13390=ORIENTED_EDGE('',*,*,#9578,.F.);
#13391=ORIENTED_EDGE('',*,*,#9575,.F.);
#13392=ORIENTED_EDGE('',*,*,#9572,.F.);
#13393=ORIENTED_EDGE('',*,*,#9580,.T.);
#13394=ORIENTED_EDGE('',*,*,#9581,.F.);
#13395=ORIENTED_EDGE('',*,*,#9582,.F.);
#13396=ORIENTED_EDGE('',*,*,#9583,.T.);
#13397=ORIENTED_EDGE('',*,*,#9584,.T.);
#13398=ORIENTED_EDGE('',*,*,#9585,.F.);
#13399=ORIENTED_EDGE('',*,*,#9586,.F.);
#13400=ORIENTED_EDGE('',*,*,#9581,.T.);
#13401=ORIENTED_EDGE('',*,*,#9587,.T.);
#13402=ORIENTED_EDGE('',*,*,#9588,.F.);
#13403=ORIENTED_EDGE('',*,*,#9589,.F.);
#13404=ORIENTED_EDGE('',*,*,#9585,.T.);
#13405=ORIENTED_EDGE('',*,*,#9590,.T.);
#13406=ORIENTED_EDGE('',*,*,#9583,.F.);
#13407=ORIENTED_EDGE('',*,*,#9591,.F.);
#13408=ORIENTED_EDGE('',*,*,#9588,.T.);
#13409=ORIENTED_EDGE('',*,*,#9582,.T.);
#13410=ORIENTED_EDGE('',*,*,#9586,.T.);
#13411=ORIENTED_EDGE('',*,*,#9589,.T.);
#13412=ORIENTED_EDGE('',*,*,#9591,.T.);
#13413=ORIENTED_EDGE('',*,*,#9580,.F.);
#13414=ORIENTED_EDGE('',*,*,#9590,.F.);
#13415=ORIENTED_EDGE('',*,*,#9587,.F.);
#13416=ORIENTED_EDGE('',*,*,#9584,.F.);
#13417=ORIENTED_EDGE('',*,*,#9592,.T.);
#13418=ORIENTED_EDGE('',*,*,#9593,.F.);
#13419=ORIENTED_EDGE('',*,*,#9594,.F.);
#13420=ORIENTED_EDGE('',*,*,#9595,.T.);
#13421=ORIENTED_EDGE('',*,*,#9596,.T.);
#13422=ORIENTED_EDGE('',*,*,#9597,.F.);
#13423=ORIENTED_EDGE('',*,*,#9598,.F.);
#13424=ORIENTED_EDGE('',*,*,#9593,.T.);
#13425=ORIENTED_EDGE('',*,*,#9599,.T.);
#13426=ORIENTED_EDGE('',*,*,#9600,.F.);
#13427=ORIENTED_EDGE('',*,*,#9601,.F.);
#13428=ORIENTED_EDGE('',*,*,#9597,.T.);
#13429=ORIENTED_EDGE('',*,*,#9602,.T.);
#13430=ORIENTED_EDGE('',*,*,#9595,.F.);
#13431=ORIENTED_EDGE('',*,*,#9603,.F.);
#13432=ORIENTED_EDGE('',*,*,#9600,.T.);
#13433=ORIENTED_EDGE('',*,*,#9594,.T.);
#13434=ORIENTED_EDGE('',*,*,#9598,.T.);
#13435=ORIENTED_EDGE('',*,*,#9601,.T.);
#13436=ORIENTED_EDGE('',*,*,#9603,.T.);
#13437=ORIENTED_EDGE('',*,*,#9592,.F.);
#13438=ORIENTED_EDGE('',*,*,#9602,.F.);
#13439=ORIENTED_EDGE('',*,*,#9599,.F.);
#13440=ORIENTED_EDGE('',*,*,#9596,.F.);
#13441=ORIENTED_EDGE('',*,*,#9604,.T.);
#13442=ORIENTED_EDGE('',*,*,#9605,.F.);
#13443=ORIENTED_EDGE('',*,*,#9606,.F.);
#13444=ORIENTED_EDGE('',*,*,#9607,.T.);
#13445=ORIENTED_EDGE('',*,*,#9608,.T.);
#13446=ORIENTED_EDGE('',*,*,#9609,.F.);
#13447=ORIENTED_EDGE('',*,*,#9610,.F.);
#13448=ORIENTED_EDGE('',*,*,#9605,.T.);
#13449=ORIENTED_EDGE('',*,*,#9611,.T.);
#13450=ORIENTED_EDGE('',*,*,#9612,.F.);
#13451=ORIENTED_EDGE('',*,*,#9613,.F.);
#13452=ORIENTED_EDGE('',*,*,#9609,.T.);
#13453=ORIENTED_EDGE('',*,*,#9614,.T.);
#13454=ORIENTED_EDGE('',*,*,#9607,.F.);
#13455=ORIENTED_EDGE('',*,*,#9615,.F.);
#13456=ORIENTED_EDGE('',*,*,#9612,.T.);
#13457=ORIENTED_EDGE('',*,*,#9606,.T.);
#13458=ORIENTED_EDGE('',*,*,#9610,.T.);
#13459=ORIENTED_EDGE('',*,*,#9613,.T.);
#13460=ORIENTED_EDGE('',*,*,#9615,.T.);
#13461=ORIENTED_EDGE('',*,*,#9604,.F.);
#13462=ORIENTED_EDGE('',*,*,#9614,.F.);
#13463=ORIENTED_EDGE('',*,*,#9611,.F.);
#13464=ORIENTED_EDGE('',*,*,#9608,.F.);
#13465=ORIENTED_EDGE('',*,*,#9616,.T.);
#13466=ORIENTED_EDGE('',*,*,#9617,.F.);
#13467=ORIENTED_EDGE('',*,*,#9618,.F.);
#13468=ORIENTED_EDGE('',*,*,#9619,.T.);
#13469=ORIENTED_EDGE('',*,*,#9620,.T.);
#13470=ORIENTED_EDGE('',*,*,#9621,.F.);
#13471=ORIENTED_EDGE('',*,*,#9622,.F.);
#13472=ORIENTED_EDGE('',*,*,#9617,.T.);
#13473=ORIENTED_EDGE('',*,*,#9623,.T.);
#13474=ORIENTED_EDGE('',*,*,#9624,.F.);
#13475=ORIENTED_EDGE('',*,*,#9625,.F.);
#13476=ORIENTED_EDGE('',*,*,#9621,.T.);
#13477=ORIENTED_EDGE('',*,*,#9626,.T.);
#13478=ORIENTED_EDGE('',*,*,#9619,.F.);
#13479=ORIENTED_EDGE('',*,*,#9627,.F.);
#13480=ORIENTED_EDGE('',*,*,#9624,.T.);
#13481=ORIENTED_EDGE('',*,*,#9618,.T.);
#13482=ORIENTED_EDGE('',*,*,#9622,.T.);
#13483=ORIENTED_EDGE('',*,*,#9625,.T.);
#13484=ORIENTED_EDGE('',*,*,#9627,.T.);
#13485=ORIENTED_EDGE('',*,*,#9616,.F.);
#13486=ORIENTED_EDGE('',*,*,#9626,.F.);
#13487=ORIENTED_EDGE('',*,*,#9623,.F.);
#13488=ORIENTED_EDGE('',*,*,#9620,.F.);
#13489=ORIENTED_EDGE('',*,*,#9628,.T.);
#13490=ORIENTED_EDGE('',*,*,#9629,.F.);
#13491=ORIENTED_EDGE('',*,*,#9630,.F.);
#13492=ORIENTED_EDGE('',*,*,#9631,.T.);
#13493=ORIENTED_EDGE('',*,*,#9632,.T.);
#13494=ORIENTED_EDGE('',*,*,#9633,.F.);
#13495=ORIENTED_EDGE('',*,*,#9634,.F.);
#13496=ORIENTED_EDGE('',*,*,#9629,.T.);
#13497=ORIENTED_EDGE('',*,*,#9635,.T.);
#13498=ORIENTED_EDGE('',*,*,#9636,.F.);
#13499=ORIENTED_EDGE('',*,*,#9637,.F.);
#13500=ORIENTED_EDGE('',*,*,#9633,.T.);
#13501=ORIENTED_EDGE('',*,*,#9638,.T.);
#13502=ORIENTED_EDGE('',*,*,#9631,.F.);
#13503=ORIENTED_EDGE('',*,*,#9639,.F.);
#13504=ORIENTED_EDGE('',*,*,#9636,.T.);
#13505=ORIENTED_EDGE('',*,*,#9630,.T.);
#13506=ORIENTED_EDGE('',*,*,#9634,.T.);
#13507=ORIENTED_EDGE('',*,*,#9637,.T.);
#13508=ORIENTED_EDGE('',*,*,#9639,.T.);
#13509=ORIENTED_EDGE('',*,*,#9628,.F.);
#13510=ORIENTED_EDGE('',*,*,#9638,.F.);
#13511=ORIENTED_EDGE('',*,*,#9635,.F.);
#13512=ORIENTED_EDGE('',*,*,#9632,.F.);
#13513=ORIENTED_EDGE('',*,*,#9640,.T.);
#13514=ORIENTED_EDGE('',*,*,#9641,.F.);
#13515=ORIENTED_EDGE('',*,*,#9642,.F.);
#13516=ORIENTED_EDGE('',*,*,#9643,.T.);
#13517=ORIENTED_EDGE('',*,*,#9644,.T.);
#13518=ORIENTED_EDGE('',*,*,#9645,.F.);
#13519=ORIENTED_EDGE('',*,*,#9646,.F.);
#13520=ORIENTED_EDGE('',*,*,#9641,.T.);
#13521=ORIENTED_EDGE('',*,*,#9647,.T.);
#13522=ORIENTED_EDGE('',*,*,#9648,.F.);
#13523=ORIENTED_EDGE('',*,*,#9649,.F.);
#13524=ORIENTED_EDGE('',*,*,#9645,.T.);
#13525=ORIENTED_EDGE('',*,*,#9650,.T.);
#13526=ORIENTED_EDGE('',*,*,#9643,.F.);
#13527=ORIENTED_EDGE('',*,*,#9651,.F.);
#13528=ORIENTED_EDGE('',*,*,#9648,.T.);
#13529=ORIENTED_EDGE('',*,*,#9642,.T.);
#13530=ORIENTED_EDGE('',*,*,#9646,.T.);
#13531=ORIENTED_EDGE('',*,*,#9649,.T.);
#13532=ORIENTED_EDGE('',*,*,#9651,.T.);
#13533=ORIENTED_EDGE('',*,*,#9640,.F.);
#13534=ORIENTED_EDGE('',*,*,#9650,.F.);
#13535=ORIENTED_EDGE('',*,*,#9647,.F.);
#13536=ORIENTED_EDGE('',*,*,#9644,.F.);
#13537=ORIENTED_EDGE('',*,*,#9652,.T.);
#13538=ORIENTED_EDGE('',*,*,#9653,.F.);
#13539=ORIENTED_EDGE('',*,*,#9654,.F.);
#13540=ORIENTED_EDGE('',*,*,#9655,.T.);
#13541=ORIENTED_EDGE('',*,*,#9656,.T.);
#13542=ORIENTED_EDGE('',*,*,#9657,.F.);
#13543=ORIENTED_EDGE('',*,*,#9658,.F.);
#13544=ORIENTED_EDGE('',*,*,#9653,.T.);
#13545=ORIENTED_EDGE('',*,*,#9659,.T.);
#13546=ORIENTED_EDGE('',*,*,#9660,.F.);
#13547=ORIENTED_EDGE('',*,*,#9661,.F.);
#13548=ORIENTED_EDGE('',*,*,#9657,.T.);
#13549=ORIENTED_EDGE('',*,*,#9662,.T.);
#13550=ORIENTED_EDGE('',*,*,#9655,.F.);
#13551=ORIENTED_EDGE('',*,*,#9663,.F.);
#13552=ORIENTED_EDGE('',*,*,#9660,.T.);
#13553=ORIENTED_EDGE('',*,*,#9654,.T.);
#13554=ORIENTED_EDGE('',*,*,#9658,.T.);
#13555=ORIENTED_EDGE('',*,*,#9661,.T.);
#13556=ORIENTED_EDGE('',*,*,#9663,.T.);
#13557=ORIENTED_EDGE('',*,*,#9652,.F.);
#13558=ORIENTED_EDGE('',*,*,#9662,.F.);
#13559=ORIENTED_EDGE('',*,*,#9659,.F.);
#13560=ORIENTED_EDGE('',*,*,#9656,.F.);
#13561=ORIENTED_EDGE('',*,*,#9664,.F.);
#13562=ORIENTED_EDGE('',*,*,#9665,.F.);
#13563=ORIENTED_EDGE('',*,*,#9666,.T.);
#13564=ORIENTED_EDGE('',*,*,#9667,.T.);
#13565=ORIENTED_EDGE('',*,*,#9668,.F.);
#13566=ORIENTED_EDGE('',*,*,#9667,.F.);
#13567=ORIENTED_EDGE('',*,*,#9669,.T.);
#13568=ORIENTED_EDGE('',*,*,#9670,.T.);
#13569=ORIENTED_EDGE('',*,*,#9671,.F.);
#13570=ORIENTED_EDGE('',*,*,#9670,.F.);
#13571=ORIENTED_EDGE('',*,*,#9672,.T.);
#13572=ORIENTED_EDGE('',*,*,#9673,.T.);
#13573=ORIENTED_EDGE('',*,*,#9674,.F.);
#13574=ORIENTED_EDGE('',*,*,#9673,.F.);
#13575=ORIENTED_EDGE('',*,*,#9675,.T.);
#13576=ORIENTED_EDGE('',*,*,#9665,.T.);
#13577=ORIENTED_EDGE('',*,*,#9666,.F.);
#13578=ORIENTED_EDGE('',*,*,#9675,.F.);
#13579=ORIENTED_EDGE('',*,*,#9672,.F.);
#13580=ORIENTED_EDGE('',*,*,#9669,.F.);
#13581=ORIENTED_EDGE('',*,*,#9664,.T.);
#13582=ORIENTED_EDGE('',*,*,#9668,.T.);
#13583=ORIENTED_EDGE('',*,*,#9671,.T.);
#13584=ORIENTED_EDGE('',*,*,#9674,.T.);
#13585=ORIENTED_EDGE('',*,*,#9676,.F.);
#13586=ORIENTED_EDGE('',*,*,#9677,.F.);
#13587=ORIENTED_EDGE('',*,*,#9678,.T.);
#13588=ORIENTED_EDGE('',*,*,#9679,.T.);
#13589=ORIENTED_EDGE('',*,*,#9680,.F.);
#13590=ORIENTED_EDGE('',*,*,#9679,.F.);
#13591=ORIENTED_EDGE('',*,*,#9681,.T.);
#13592=ORIENTED_EDGE('',*,*,#9682,.T.);
#13593=ORIENTED_EDGE('',*,*,#9683,.F.);
#13594=ORIENTED_EDGE('',*,*,#9682,.F.);
#13595=ORIENTED_EDGE('',*,*,#9684,.T.);
#13596=ORIENTED_EDGE('',*,*,#9685,.T.);
#13597=ORIENTED_EDGE('',*,*,#9686,.F.);
#13598=ORIENTED_EDGE('',*,*,#9685,.F.);
#13599=ORIENTED_EDGE('',*,*,#9687,.T.);
#13600=ORIENTED_EDGE('',*,*,#9677,.T.);
#13601=ORIENTED_EDGE('',*,*,#9678,.F.);
#13602=ORIENTED_EDGE('',*,*,#9687,.F.);
#13603=ORIENTED_EDGE('',*,*,#9684,.F.);
#13604=ORIENTED_EDGE('',*,*,#9681,.F.);
#13605=ORIENTED_EDGE('',*,*,#9676,.T.);
#13606=ORIENTED_EDGE('',*,*,#9680,.T.);
#13607=ORIENTED_EDGE('',*,*,#9683,.T.);
#13608=ORIENTED_EDGE('',*,*,#9686,.T.);
#13609=ORIENTED_EDGE('',*,*,#9688,.F.);
#13610=ORIENTED_EDGE('',*,*,#9689,.F.);
#13611=ORIENTED_EDGE('',*,*,#9690,.T.);
#13612=ORIENTED_EDGE('',*,*,#9691,.T.);
#13613=ORIENTED_EDGE('',*,*,#9692,.F.);
#13614=ORIENTED_EDGE('',*,*,#9691,.F.);
#13615=ORIENTED_EDGE('',*,*,#9693,.T.);
#13616=ORIENTED_EDGE('',*,*,#9694,.T.);
#13617=ORIENTED_EDGE('',*,*,#9695,.F.);
#13618=ORIENTED_EDGE('',*,*,#9694,.F.);
#13619=ORIENTED_EDGE('',*,*,#9696,.T.);
#13620=ORIENTED_EDGE('',*,*,#9697,.T.);
#13621=ORIENTED_EDGE('',*,*,#9698,.F.);
#13622=ORIENTED_EDGE('',*,*,#9697,.F.);
#13623=ORIENTED_EDGE('',*,*,#9699,.T.);
#13624=ORIENTED_EDGE('',*,*,#9689,.T.);
#13625=ORIENTED_EDGE('',*,*,#9690,.F.);
#13626=ORIENTED_EDGE('',*,*,#9699,.F.);
#13627=ORIENTED_EDGE('',*,*,#9696,.F.);
#13628=ORIENTED_EDGE('',*,*,#9693,.F.);
#13629=ORIENTED_EDGE('',*,*,#9688,.T.);
#13630=ORIENTED_EDGE('',*,*,#9692,.T.);
#13631=ORIENTED_EDGE('',*,*,#9695,.T.);
#13632=ORIENTED_EDGE('',*,*,#9698,.T.);
#13633=ORIENTED_EDGE('',*,*,#9700,.F.);
#13634=ORIENTED_EDGE('',*,*,#9701,.F.);
#13635=ORIENTED_EDGE('',*,*,#9702,.T.);
#13636=ORIENTED_EDGE('',*,*,#9703,.T.);
#13637=ORIENTED_EDGE('',*,*,#9704,.F.);
#13638=ORIENTED_EDGE('',*,*,#9703,.F.);
#13639=ORIENTED_EDGE('',*,*,#9705,.T.);
#13640=ORIENTED_EDGE('',*,*,#9706,.T.);
#13641=ORIENTED_EDGE('',*,*,#9707,.F.);
#13642=ORIENTED_EDGE('',*,*,#9706,.F.);
#13643=ORIENTED_EDGE('',*,*,#9708,.T.);
#13644=ORIENTED_EDGE('',*,*,#9709,.T.);
#13645=ORIENTED_EDGE('',*,*,#9710,.F.);
#13646=ORIENTED_EDGE('',*,*,#9709,.F.);
#13647=ORIENTED_EDGE('',*,*,#9711,.T.);
#13648=ORIENTED_EDGE('',*,*,#9701,.T.);
#13649=ORIENTED_EDGE('',*,*,#9702,.F.);
#13650=ORIENTED_EDGE('',*,*,#9711,.F.);
#13651=ORIENTED_EDGE('',*,*,#9708,.F.);
#13652=ORIENTED_EDGE('',*,*,#9705,.F.);
#13653=ORIENTED_EDGE('',*,*,#9700,.T.);
#13654=ORIENTED_EDGE('',*,*,#9704,.T.);
#13655=ORIENTED_EDGE('',*,*,#9707,.T.);
#13656=ORIENTED_EDGE('',*,*,#9710,.T.);
#13657=ORIENTED_EDGE('',*,*,#9712,.F.);
#13658=ORIENTED_EDGE('',*,*,#9713,.F.);
#13659=ORIENTED_EDGE('',*,*,#9714,.T.);
#13660=ORIENTED_EDGE('',*,*,#9715,.T.);
#13661=ORIENTED_EDGE('',*,*,#9716,.F.);
#13662=ORIENTED_EDGE('',*,*,#9715,.F.);
#13663=ORIENTED_EDGE('',*,*,#9717,.T.);
#13664=ORIENTED_EDGE('',*,*,#9718,.T.);
#13665=ORIENTED_EDGE('',*,*,#9719,.F.);
#13666=ORIENTED_EDGE('',*,*,#9718,.F.);
#13667=ORIENTED_EDGE('',*,*,#9720,.T.);
#13668=ORIENTED_EDGE('',*,*,#9721,.T.);
#13669=ORIENTED_EDGE('',*,*,#9722,.F.);
#13670=ORIENTED_EDGE('',*,*,#9721,.F.);
#13671=ORIENTED_EDGE('',*,*,#9723,.T.);
#13672=ORIENTED_EDGE('',*,*,#9713,.T.);
#13673=ORIENTED_EDGE('',*,*,#9714,.F.);
#13674=ORIENTED_EDGE('',*,*,#9723,.F.);
#13675=ORIENTED_EDGE('',*,*,#9720,.F.);
#13676=ORIENTED_EDGE('',*,*,#9717,.F.);
#13677=ORIENTED_EDGE('',*,*,#9712,.T.);
#13678=ORIENTED_EDGE('',*,*,#9716,.T.);
#13679=ORIENTED_EDGE('',*,*,#9719,.T.);
#13680=ORIENTED_EDGE('',*,*,#9722,.T.);
#13681=ORIENTED_EDGE('',*,*,#9724,.T.);
#13682=ORIENTED_EDGE('',*,*,#9725,.F.);
#13683=ORIENTED_EDGE('',*,*,#9726,.F.);
#13684=ORIENTED_EDGE('',*,*,#9727,.T.);
#13685=ORIENTED_EDGE('',*,*,#9728,.T.);
#13686=ORIENTED_EDGE('',*,*,#9729,.F.);
#13687=ORIENTED_EDGE('',*,*,#9730,.F.);
#13688=ORIENTED_EDGE('',*,*,#9725,.T.);
#13689=ORIENTED_EDGE('',*,*,#9731,.T.);
#13690=ORIENTED_EDGE('',*,*,#9732,.F.);
#13691=ORIENTED_EDGE('',*,*,#9733,.F.);
#13692=ORIENTED_EDGE('',*,*,#9729,.T.);
#13693=ORIENTED_EDGE('',*,*,#9734,.T.);
#13694=ORIENTED_EDGE('',*,*,#9727,.F.);
#13695=ORIENTED_EDGE('',*,*,#9735,.F.);
#13696=ORIENTED_EDGE('',*,*,#9732,.T.);
#13697=ORIENTED_EDGE('',*,*,#9726,.T.);
#13698=ORIENTED_EDGE('',*,*,#9730,.T.);
#13699=ORIENTED_EDGE('',*,*,#9733,.T.);
#13700=ORIENTED_EDGE('',*,*,#9735,.T.);
#13701=ORIENTED_EDGE('',*,*,#9724,.F.);
#13702=ORIENTED_EDGE('',*,*,#9734,.F.);
#13703=ORIENTED_EDGE('',*,*,#9731,.F.);
#13704=ORIENTED_EDGE('',*,*,#9728,.F.);
#13705=ORIENTED_EDGE('',*,*,#9736,.T.);
#13706=ORIENTED_EDGE('',*,*,#9737,.F.);
#13707=ORIENTED_EDGE('',*,*,#9738,.F.);
#13708=ORIENTED_EDGE('',*,*,#9739,.T.);
#13709=ORIENTED_EDGE('',*,*,#9740,.T.);
#13710=ORIENTED_EDGE('',*,*,#9741,.F.);
#13711=ORIENTED_EDGE('',*,*,#9742,.F.);
#13712=ORIENTED_EDGE('',*,*,#9737,.T.);
#13713=ORIENTED_EDGE('',*,*,#9743,.T.);
#13714=ORIENTED_EDGE('',*,*,#9744,.F.);
#13715=ORIENTED_EDGE('',*,*,#9745,.F.);
#13716=ORIENTED_EDGE('',*,*,#9741,.T.);
#13717=ORIENTED_EDGE('',*,*,#9746,.T.);
#13718=ORIENTED_EDGE('',*,*,#9739,.F.);
#13719=ORIENTED_EDGE('',*,*,#9747,.F.);
#13720=ORIENTED_EDGE('',*,*,#9744,.T.);
#13721=ORIENTED_EDGE('',*,*,#9738,.T.);
#13722=ORIENTED_EDGE('',*,*,#9742,.T.);
#13723=ORIENTED_EDGE('',*,*,#9745,.T.);
#13724=ORIENTED_EDGE('',*,*,#9747,.T.);
#13725=ORIENTED_EDGE('',*,*,#9736,.F.);
#13726=ORIENTED_EDGE('',*,*,#9746,.F.);
#13727=ORIENTED_EDGE('',*,*,#9743,.F.);
#13728=ORIENTED_EDGE('',*,*,#9740,.F.);
#13729=ORIENTED_EDGE('',*,*,#9748,.T.);
#13730=ORIENTED_EDGE('',*,*,#9749,.F.);
#13731=ORIENTED_EDGE('',*,*,#9750,.F.);
#13732=ORIENTED_EDGE('',*,*,#9751,.T.);
#13733=ORIENTED_EDGE('',*,*,#9752,.T.);
#13734=ORIENTED_EDGE('',*,*,#9753,.F.);
#13735=ORIENTED_EDGE('',*,*,#9754,.F.);
#13736=ORIENTED_EDGE('',*,*,#9749,.T.);
#13737=ORIENTED_EDGE('',*,*,#9755,.T.);
#13738=ORIENTED_EDGE('',*,*,#9756,.F.);
#13739=ORIENTED_EDGE('',*,*,#9757,.F.);
#13740=ORIENTED_EDGE('',*,*,#9753,.T.);
#13741=ORIENTED_EDGE('',*,*,#9758,.T.);
#13742=ORIENTED_EDGE('',*,*,#9751,.F.);
#13743=ORIENTED_EDGE('',*,*,#9759,.F.);
#13744=ORIENTED_EDGE('',*,*,#9756,.T.);
#13745=ORIENTED_EDGE('',*,*,#9750,.T.);
#13746=ORIENTED_EDGE('',*,*,#9754,.T.);
#13747=ORIENTED_EDGE('',*,*,#9757,.T.);
#13748=ORIENTED_EDGE('',*,*,#9759,.T.);
#13749=ORIENTED_EDGE('',*,*,#9748,.F.);
#13750=ORIENTED_EDGE('',*,*,#9758,.F.);
#13751=ORIENTED_EDGE('',*,*,#9755,.F.);
#13752=ORIENTED_EDGE('',*,*,#9752,.F.);
#13753=ORIENTED_EDGE('',*,*,#9760,.T.);
#13754=ORIENTED_EDGE('',*,*,#9761,.F.);
#13755=ORIENTED_EDGE('',*,*,#9762,.F.);
#13756=ORIENTED_EDGE('',*,*,#9763,.T.);
#13757=ORIENTED_EDGE('',*,*,#9764,.T.);
#13758=ORIENTED_EDGE('',*,*,#9765,.F.);
#13759=ORIENTED_EDGE('',*,*,#9766,.F.);
#13760=ORIENTED_EDGE('',*,*,#9761,.T.);
#13761=ORIENTED_EDGE('',*,*,#9767,.T.);
#13762=ORIENTED_EDGE('',*,*,#9768,.F.);
#13763=ORIENTED_EDGE('',*,*,#9769,.F.);
#13764=ORIENTED_EDGE('',*,*,#9765,.T.);
#13765=ORIENTED_EDGE('',*,*,#9770,.T.);
#13766=ORIENTED_EDGE('',*,*,#9763,.F.);
#13767=ORIENTED_EDGE('',*,*,#9771,.F.);
#13768=ORIENTED_EDGE('',*,*,#9768,.T.);
#13769=ORIENTED_EDGE('',*,*,#9762,.T.);
#13770=ORIENTED_EDGE('',*,*,#9766,.T.);
#13771=ORIENTED_EDGE('',*,*,#9769,.T.);
#13772=ORIENTED_EDGE('',*,*,#9771,.T.);
#13773=ORIENTED_EDGE('',*,*,#9760,.F.);
#13774=ORIENTED_EDGE('',*,*,#9770,.F.);
#13775=ORIENTED_EDGE('',*,*,#9767,.F.);
#13776=ORIENTED_EDGE('',*,*,#9764,.F.);
#13777=ORIENTED_EDGE('',*,*,#9772,.T.);
#13778=ORIENTED_EDGE('',*,*,#9773,.F.);
#13779=ORIENTED_EDGE('',*,*,#9774,.F.);
#13780=ORIENTED_EDGE('',*,*,#9775,.T.);
#13781=ORIENTED_EDGE('',*,*,#9776,.T.);
#13782=ORIENTED_EDGE('',*,*,#9777,.F.);
#13783=ORIENTED_EDGE('',*,*,#9778,.F.);
#13784=ORIENTED_EDGE('',*,*,#9773,.T.);
#13785=ORIENTED_EDGE('',*,*,#9779,.T.);
#13786=ORIENTED_EDGE('',*,*,#9780,.F.);
#13787=ORIENTED_EDGE('',*,*,#9781,.F.);
#13788=ORIENTED_EDGE('',*,*,#9777,.T.);
#13789=ORIENTED_EDGE('',*,*,#9782,.T.);
#13790=ORIENTED_EDGE('',*,*,#9775,.F.);
#13791=ORIENTED_EDGE('',*,*,#9783,.F.);
#13792=ORIENTED_EDGE('',*,*,#9780,.T.);
#13793=ORIENTED_EDGE('',*,*,#9774,.T.);
#13794=ORIENTED_EDGE('',*,*,#9778,.T.);
#13795=ORIENTED_EDGE('',*,*,#9781,.T.);
#13796=ORIENTED_EDGE('',*,*,#9783,.T.);
#13797=ORIENTED_EDGE('',*,*,#9772,.F.);
#13798=ORIENTED_EDGE('',*,*,#9782,.F.);
#13799=ORIENTED_EDGE('',*,*,#9779,.F.);
#13800=ORIENTED_EDGE('',*,*,#9776,.F.);
#13801=ORIENTED_EDGE('',*,*,#9784,.T.);
#13802=ORIENTED_EDGE('',*,*,#9785,.F.);
#13803=ORIENTED_EDGE('',*,*,#9786,.F.);
#13804=ORIENTED_EDGE('',*,*,#9787,.T.);
#13805=ORIENTED_EDGE('',*,*,#9788,.T.);
#13806=ORIENTED_EDGE('',*,*,#9789,.F.);
#13807=ORIENTED_EDGE('',*,*,#9790,.F.);
#13808=ORIENTED_EDGE('',*,*,#9785,.T.);
#13809=ORIENTED_EDGE('',*,*,#9791,.T.);
#13810=ORIENTED_EDGE('',*,*,#9792,.F.);
#13811=ORIENTED_EDGE('',*,*,#9793,.F.);
#13812=ORIENTED_EDGE('',*,*,#9789,.T.);
#13813=ORIENTED_EDGE('',*,*,#9794,.T.);
#13814=ORIENTED_EDGE('',*,*,#9787,.F.);
#13815=ORIENTED_EDGE('',*,*,#9795,.F.);
#13816=ORIENTED_EDGE('',*,*,#9792,.T.);
#13817=ORIENTED_EDGE('',*,*,#9786,.T.);
#13818=ORIENTED_EDGE('',*,*,#9790,.T.);
#13819=ORIENTED_EDGE('',*,*,#9793,.T.);
#13820=ORIENTED_EDGE('',*,*,#9795,.T.);
#13821=ORIENTED_EDGE('',*,*,#9784,.F.);
#13822=ORIENTED_EDGE('',*,*,#9794,.F.);
#13823=ORIENTED_EDGE('',*,*,#9791,.F.);
#13824=ORIENTED_EDGE('',*,*,#9788,.F.);
#14266=PLANE('',#16549);
#14267=PLANE('',#16550);
#14268=PLANE('',#16551);
#14269=PLANE('',#16552);
#14270=PLANE('',#16553);
#14271=PLANE('',#16554);
#14272=PLANE('',#16558);
#14273=PLANE('',#16560);
#14274=PLANE('',#16562);
#14275=PLANE('',#16563);
#14276=PLANE('',#16564);
#14277=PLANE('',#16565);
#14278=PLANE('',#16567);
#14279=PLANE('',#16571);
#14280=PLANE('',#16573);
#14281=PLANE('',#16575);
#14282=PLANE('',#16576);
#14283=PLANE('',#16577);
#14284=PLANE('',#16578);
#14285=PLANE('',#16580);
#14286=PLANE('',#16596);
#14287=PLANE('',#16597);
#14288=PLANE('',#16598);
#14289=PLANE('',#16599);
#14290=PLANE('',#16600);
#14291=PLANE('',#16601);
#14292=PLANE('',#16602);
#14293=PLANE('',#16603);
#14294=PLANE('',#16604);
#14295=PLANE('',#16605);
#14296=PLANE('',#16606);
#14297=PLANE('',#16607);
#14298=PLANE('',#16608);
#14299=PLANE('',#16609);
#14300=PLANE('',#16610);
#14301=PLANE('',#16611);
#14302=PLANE('',#16612);
#14303=PLANE('',#16613);
#14304=PLANE('',#16614);
#14305=PLANE('',#16615);
#14306=PLANE('',#16616);
#14307=PLANE('',#16617);
#14308=PLANE('',#16618);
#14309=PLANE('',#16619);
#14310=PLANE('',#16620);
#14311=PLANE('',#16621);
#14312=PLANE('',#16622);
#14313=PLANE('',#16623);
#14314=PLANE('',#16624);
#14315=PLANE('',#16625);
#14316=PLANE('',#16635);
#14317=PLANE('',#16636);
#14318=PLANE('',#16637);
#14319=PLANE('',#16638);
#14320=PLANE('',#16639);
#14321=PLANE('',#16640);
#14322=PLANE('',#16650);
#14323=PLANE('',#16651);
#14324=PLANE('',#16652);
#14325=PLANE('',#16653);
#14326=PLANE('',#16654);
#14327=PLANE('',#16655);
#14328=PLANE('',#16665);
#14329=PLANE('',#16666);
#14330=PLANE('',#16667);
#14331=PLANE('',#16668);
#14332=PLANE('',#16669);
#14333=PLANE('',#16670);
#14334=PLANE('',#16680);
#14335=PLANE('',#16681);
#14336=PLANE('',#16682);
#14337=PLANE('',#16683);
#14338=PLANE('',#16684);
#14339=PLANE('',#16685);
#14340=PLANE('',#16686);
#14341=PLANE('',#16687);
#14342=PLANE('',#16688);
#14343=PLANE('',#16689);
#14344=PLANE('',#16690);
#14345=PLANE('',#16691);
#14346=PLANE('',#16692);
#14347=PLANE('',#16693);
#14348=PLANE('',#16694);
#14349=PLANE('',#16695);
#14350=PLANE('',#16696);
#14351=PLANE('',#16697);
#14352=PLANE('',#16698);
#14353=PLANE('',#16699);
#14354=PLANE('',#16700);
#14355=PLANE('',#16701);
#14356=PLANE('',#16702);
#14357=PLANE('',#16703);
#14358=PLANE('',#16704);
#14359=PLANE('',#16705);
#14360=PLANE('',#16706);
#14361=PLANE('',#16707);
#14362=PLANE('',#16708);
#14363=PLANE('',#16709);
#14364=PLANE('',#16710);
#14365=PLANE('',#16711);
#14366=PLANE('',#16712);
#14367=PLANE('',#16713);
#14368=PLANE('',#16714);
#14369=PLANE('',#16715);
#14370=PLANE('',#16728);
#14371=PLANE('',#16729);
#14372=PLANE('',#16730);
#14373=PLANE('',#16731);
#14374=PLANE('',#16732);
#14375=PLANE('',#16733);
#14376=PLANE('',#16752);
#14377=PLANE('',#16753);
#14378=PLANE('',#16754);
#14379=PLANE('',#16755);
#14380=PLANE('',#16756);
#14381=PLANE('',#16757);
#14382=PLANE('',#16758);
#14383=PLANE('',#16759);
#14384=PLANE('',#16760);
#14385=PLANE('',#16761);
#14386=PLANE('',#16762);
#14387=PLANE('',#16763);
#14388=PLANE('',#16764);
#14389=PLANE('',#16765);
#14390=PLANE('',#16766);
#14391=PLANE('',#16767);
#14392=PLANE('',#16768);
#14393=PLANE('',#16769);
#14394=PLANE('',#16770);
#14395=PLANE('',#16771);
#14396=PLANE('',#16772);
#14397=PLANE('',#16773);
#14398=PLANE('',#16774);
#14399=PLANE('',#16775);
#14400=PLANE('',#16776);
#14401=PLANE('',#16777);
#14402=PLANE('',#16778);
#14403=PLANE('',#16779);
#14404=PLANE('',#16780);
#14405=PLANE('',#16781);
#14406=PLANE('',#16782);
#14407=PLANE('',#16783);
#14408=PLANE('',#16784);
#14409=PLANE('',#16785);
#14410=PLANE('',#16786);
#14411=PLANE('',#16787);
#14412=PLANE('',#16788);
#14413=PLANE('',#16789);
#14414=PLANE('',#16790);
#14415=PLANE('',#16791);
#14416=PLANE('',#16792);
#14417=PLANE('',#16793);
#14418=PLANE('',#16794);
#14419=PLANE('',#16795);
#14420=PLANE('',#16796);
#14421=PLANE('',#16797);
#14422=PLANE('',#16798);
#14423=PLANE('',#16799);
#14424=PLANE('',#16800);
#14425=PLANE('',#16801);
#14426=PLANE('',#16802);
#14427=PLANE('',#16803);
#14428=PLANE('',#16804);
#14429=PLANE('',#16805);
#14430=PLANE('',#16806);
#14431=PLANE('',#16807);
#14432=PLANE('',#16808);
#14433=PLANE('',#16809);
#14434=PLANE('',#16810);
#14435=PLANE('',#16811);
#14436=PLANE('',#16812);
#14437=PLANE('',#16813);
#14438=PLANE('',#16814);
#14439=PLANE('',#16815);
#14440=PLANE('',#16816);
#14441=PLANE('',#16817);
#14442=PLANE('',#16818);
#14443=PLANE('',#16819);
#14444=PLANE('',#16820);
#14445=PLANE('',#16821);
#14446=PLANE('',#16822);
#14447=PLANE('',#16823);
#14448=PLANE('',#16824);
#14449=PLANE('',#16825);
#14450=PLANE('',#16826);
#14451=PLANE('',#16827);
#14452=PLANE('',#16828);
#14453=PLANE('',#16829);
#14454=PLANE('',#16830);
#14455=PLANE('',#16831);
#14456=PLANE('',#16832);
#14457=PLANE('',#16833);
#14458=PLANE('',#16834);
#14459=PLANE('',#16835);
#14460=PLANE('',#16836);
#14461=PLANE('',#16837);
#14462=PLANE('',#16838);
#14463=PLANE('',#16839);
#14464=PLANE('',#16840);
#14465=PLANE('',#16841);
#14466=PLANE('',#16842);
#14467=PLANE('',#16843);
#14468=PLANE('',#16844);
#14469=PLANE('',#16845);
#14470=PLANE('',#16846);
#14471=PLANE('',#16847);
#14472=PLANE('',#16848);
#14473=PLANE('',#16849);
#14474=PLANE('',#16850);
#14475=PLANE('',#16851);
#14476=PLANE('',#16852);
#14477=PLANE('',#16853);
#14478=PLANE('',#16854);
#14479=PLANE('',#16855);
#14480=PLANE('',#16856);
#14481=PLANE('',#16869);
#14482=PLANE('',#16870);
#14483=PLANE('',#16871);
#14484=PLANE('',#16872);
#14485=PLANE('',#16873);
#14486=PLANE('',#16874);
#14487=PLANE('',#16875);
#14488=PLANE('',#16876);
#14489=PLANE('',#16877);
#14490=PLANE('',#16878);
#14491=PLANE('',#16879);
#14492=PLANE('',#16880);
#14493=PLANE('',#16881);
#14494=PLANE('',#16882);
#14495=PLANE('',#16883);
#14496=PLANE('',#16884);
#14497=PLANE('',#16885);
#14498=PLANE('',#16886);
#14499=PLANE('',#16887);
#14500=PLANE('',#16888);
#14501=PLANE('',#16889);
#14502=PLANE('',#16890);
#14503=PLANE('',#16891);
#14504=PLANE('',#16892);
#14505=PLANE('',#16893);
#14506=PLANE('',#16894);
#14507=PLANE('',#16895);
#14508=PLANE('',#16896);
#14509=PLANE('',#16897);
#14510=PLANE('',#16898);
#14511=PLANE('',#16899);
#14512=PLANE('',#16900);
#14513=PLANE('',#16901);
#14514=PLANE('',#16902);
#14515=PLANE('',#16903);
#14516=PLANE('',#16904);
#14517=PLANE('',#16905);
#14518=PLANE('',#16906);
#14519=PLANE('',#16907);
#14520=PLANE('',#16908);
#14521=PLANE('',#16909);
#14522=PLANE('',#16910);
#14523=PLANE('',#16911);
#14524=PLANE('',#16912);
#14525=PLANE('',#16913);
#14526=PLANE('',#16914);
#14527=PLANE('',#16915);
#14528=PLANE('',#16916);
#14529=PLANE('',#16917);
#14530=PLANE('',#16918);
#14531=PLANE('',#16919);
#14532=PLANE('',#16920);
#14533=PLANE('',#16921);
#14534=PLANE('',#16922);
#14535=PLANE('',#16923);
#14536=PLANE('',#16924);
#14537=PLANE('',#16925);
#14538=PLANE('',#16926);
#14539=PLANE('',#16927);
#14540=PLANE('',#16928);
#14541=PLANE('',#16929);
#14542=PLANE('',#16930);
#14543=PLANE('',#16931);
#14544=PLANE('',#16932);
#14545=PLANE('',#16933);
#14546=PLANE('',#16934);
#14547=PLANE('',#16935);
#14548=PLANE('',#16936);
#14549=PLANE('',#16937);
#14550=PLANE('',#16938);
#14551=PLANE('',#16939);
#14552=PLANE('',#16940);
#14553=PLANE('',#16941);
#14554=PLANE('',#16942);
#14555=PLANE('',#16943);
#14556=PLANE('',#16944);
#14557=PLANE('',#16945);
#14558=PLANE('',#16946);
#14559=PLANE('',#16947);
#14560=PLANE('',#16948);
#14561=PLANE('',#16949);
#14562=PLANE('',#16950);
#14563=PLANE('',#16951);
#14564=PLANE('',#16952);
#14565=PLANE('',#16953);
#14566=PLANE('',#16954);
#14567=PLANE('',#16955);
#14568=PLANE('',#16956);
#14569=PLANE('',#16957);
#14570=PLANE('',#16958);
#14571=PLANE('',#16959);
#14572=PLANE('',#16960);
#14573=PLANE('',#16961);
#14574=PLANE('',#16962);
#14575=PLANE('',#16963);
#14576=PLANE('',#16964);
#14577=PLANE('',#16965);
#14578=PLANE('',#16966);
#14579=PLANE('',#16967);
#14580=PLANE('',#16968);
#14581=PLANE('',#16969);
#14582=PLANE('',#16970);
#14583=PLANE('',#16971);
#14584=PLANE('',#16972);
#14585=PLANE('',#16973);
#14586=PLANE('',#16974);
#14587=PLANE('',#16975);
#14588=PLANE('',#16976);
#14589=PLANE('',#16977);
#14590=PLANE('',#16978);
#14591=PLANE('',#16979);
#14592=PLANE('',#16980);
#14593=PLANE('',#16981);
#14594=PLANE('',#16982);
#14595=PLANE('',#16983);
#14596=PLANE('',#16984);
#14597=PLANE('',#16985);
#14598=PLANE('',#16986);
#14599=PLANE('',#16987);
#14600=PLANE('',#16988);
#14601=PLANE('',#16989);
#14602=PLANE('',#16990);
#14603=PLANE('',#16991);
#14604=PLANE('',#16992);
#14605=PLANE('',#16993);
#14606=PLANE('',#16994);
#14607=PLANE('',#16995);
#14608=PLANE('',#16996);
#14609=PLANE('',#16997);
#14610=PLANE('',#16998);
#14611=PLANE('',#16999);
#14612=PLANE('',#17000);
#14613=PLANE('',#17001);
#14614=PLANE('',#17002);
#14615=PLANE('',#17003);
#14616=PLANE('',#17004);
#14617=PLANE('',#17005);
#14618=PLANE('',#17006);
#15098=ADVANCED_FACE('',(#2130),#14266,.F.);
#15099=ADVANCED_FACE('',(#2131),#14267,.F.);
#15100=ADVANCED_FACE('',(#2132),#14268,.F.);
#15101=ADVANCED_FACE('',(#2133),#14269,.F.);
#15102=ADVANCED_FACE('',(#2134),#14270,.F.);
#15103=ADVANCED_FACE('',(#2135),#14271,.T.);
#15104=ADVANCED_FACE('',(#2136),#1250,.F.);
#15105=ADVANCED_FACE('',(#2137,#1605),#14272,.T.);
#15106=ADVANCED_FACE('',(#2138,#1606),#14273,.F.);
#15107=ADVANCED_FACE('',(#2139),#14274,.F.);
#15108=ADVANCED_FACE('',(#2140),#14275,.F.);
#15109=ADVANCED_FACE('',(#2141),#14276,.F.);
#15110=ADVANCED_FACE('',(#2142),#14277,.F.);
#15111=ADVANCED_FACE('',(#2143),#1251,.F.);
#15112=ADVANCED_FACE('',(#2144),#14278,.F.);
#15113=ADVANCED_FACE('',(#2145),#1252,.F.);
#15114=ADVANCED_FACE('',(#2146,#1607),#14279,.T.);
#15115=ADVANCED_FACE('',(#2147,#1608),#14280,.F.);
#15116=ADVANCED_FACE('',(#2148),#14281,.F.);
#15117=ADVANCED_FACE('',(#2149),#14282,.F.);
#15118=ADVANCED_FACE('',(#2150),#14283,.F.);
#15119=ADVANCED_FACE('',(#2151),#14284,.F.);
#15120=ADVANCED_FACE('',(#2152),#1253,.F.);
#15121=ADVANCED_FACE('',(#2153),#14285,.F.);
#15122=ADVANCED_FACE('',(#2154),#1254,.F.);
#15123=ADVANCED_FACE('',(#2155),#1255,.F.);
#15124=ADVANCED_FACE('',(#2156),#1256,.F.);
#15125=ADVANCED_FACE('',(#2157),#1257,.F.);
#15126=ADVANCED_FACE('',(#2158),#1258,.F.);
#15127=ADVANCED_FACE('',(#2159,#1609,#1610,#1611,#1612,#1613),#14286,.F.);
#15128=ADVANCED_FACE('',(#2160,#1614,#1615,#1616,#1617,#1618),#14287,.T.);
#15129=ADVANCED_FACE('',(#2161),#14288,.F.);
#15130=ADVANCED_FACE('',(#2162),#14289,.F.);
#15131=ADVANCED_FACE('',(#2163),#14290,.F.);
#15132=ADVANCED_FACE('',(#2164),#14291,.F.);
#15133=ADVANCED_FACE('',(#2165),#14292,.F.);
#15134=ADVANCED_FACE('',(#2166),#14293,.F.);
#15135=ADVANCED_FACE('',(#2167),#14294,.F.);
#15136=ADVANCED_FACE('',(#2168),#14295,.F.);
#15137=ADVANCED_FACE('',(#2169),#14296,.F.);
#15138=ADVANCED_FACE('',(#2170),#14297,.F.);
#15139=ADVANCED_FACE('',(#2171),#14298,.F.);
#15140=ADVANCED_FACE('',(#2172),#14299,.F.);
#15141=ADVANCED_FACE('',(#2173),#14300,.F.);
#15142=ADVANCED_FACE('',(#2174),#14301,.T.);
#15143=ADVANCED_FACE('',(#2175),#14302,.F.);
#15144=ADVANCED_FACE('',(#2176),#14303,.F.);
#15145=ADVANCED_FACE('',(#2177),#14304,.F.);
#15146=ADVANCED_FACE('',(#2178),#14305,.F.);
#15147=ADVANCED_FACE('',(#2179),#14306,.T.);
#15148=ADVANCED_FACE('',(#2180),#14307,.F.);
#15149=ADVANCED_FACE('',(#2181),#14308,.F.);
#15150=ADVANCED_FACE('',(#2182),#14309,.F.);
#15151=ADVANCED_FACE('',(#2183),#14310,.F.);
#15152=ADVANCED_FACE('',(#2184),#14311,.F.);
#15153=ADVANCED_FACE('',(#2185),#14312,.F.);
#15154=ADVANCED_FACE('',(#2186),#14313,.F.);
#15155=ADVANCED_FACE('',(#2187),#14314,.T.);
#15156=ADVANCED_FACE('',(#2188),#14315,.F.);
#15157=ADVANCED_FACE('',(#2189),#1259,.F.);
#15158=ADVANCED_FACE('',(#2190),#1260,.F.);
#15159=ADVANCED_FACE('',(#2191),#1261,.F.);
#15160=ADVANCED_FACE('',(#2192,#1619,#1620,#1621),#14316,.T.);
#15161=ADVANCED_FACE('',(#2193,#1622,#1623,#1624),#14317,.F.);
#15162=ADVANCED_FACE('',(#2194),#14318,.F.);
#15163=ADVANCED_FACE('',(#2195),#14319,.F.);
#15164=ADVANCED_FACE('',(#2196),#14320,.F.);
#15165=ADVANCED_FACE('',(#2197),#14321,.F.);
#15166=ADVANCED_FACE('',(#2198),#1262,.F.);
#15167=ADVANCED_FACE('',(#2199),#1263,.F.);
#15168=ADVANCED_FACE('',(#2200),#1264,.F.);
#15169=ADVANCED_FACE('',(#2201,#1625,#1626,#1627),#14322,.T.);
#15170=ADVANCED_FACE('',(#2202,#1628,#1629,#1630),#14323,.F.);
#15171=ADVANCED_FACE('',(#2203),#14324,.F.);
#15172=ADVANCED_FACE('',(#2204),#14325,.F.);
#15173=ADVANCED_FACE('',(#2205),#14326,.F.);
#15174=ADVANCED_FACE('',(#2206),#14327,.F.);
#15175=ADVANCED_FACE('',(#2207),#1265,.F.);
#15176=ADVANCED_FACE('',(#2208),#1266,.F.);
#15177=ADVANCED_FACE('',(#2209),#1267,.F.);
#15178=ADVANCED_FACE('',(#2210,#1631,#1632,#1633),#14328,.T.);
#15179=ADVANCED_FACE('',(#2211,#1634,#1635,#1636),#14329,.F.);
#15180=ADVANCED_FACE('',(#2212),#14330,.F.);
#15181=ADVANCED_FACE('',(#2213),#14331,.F.);
#15182=ADVANCED_FACE('',(#2214),#14332,.F.);
#15183=ADVANCED_FACE('',(#2215),#14333,.F.);
#15184=ADVANCED_FACE('',(#2216),#1268,.F.);
#15185=ADVANCED_FACE('',(#2217),#1269,.F.);
#15186=ADVANCED_FACE('',(#2218),#1270,.F.);
#15187=ADVANCED_FACE('',(#2219,#1637,#1638,#1639),#14334,.T.);
#15188=ADVANCED_FACE('',(#2220,#1640,#1641,#1642),#14335,.F.);
#15189=ADVANCED_FACE('',(#2221),#14336,.F.);
#15190=ADVANCED_FACE('',(#2222),#14337,.F.);
#15191=ADVANCED_FACE('',(#2223),#14338,.F.);
#15192=ADVANCED_FACE('',(#2224),#14339,.F.);
#15193=ADVANCED_FACE('',(#2225),#14340,.F.);
#15194=ADVANCED_FACE('',(#2226),#14341,.F.);
#15195=ADVANCED_FACE('',(#2227),#14342,.F.);
#15196=ADVANCED_FACE('',(#2228),#14343,.F.);
#15197=ADVANCED_FACE('',(#2229),#14344,.F.);
#15198=ADVANCED_FACE('',(#2230),#14345,.T.);
#15199=ADVANCED_FACE('',(#2231),#14346,.F.);
#15200=ADVANCED_FACE('',(#2232),#14347,.F.);
#15201=ADVANCED_FACE('',(#2233),#14348,.F.);
#15202=ADVANCED_FACE('',(#2234),#14349,.F.);
#15203=ADVANCED_FACE('',(#2235),#14350,.T.);
#15204=ADVANCED_FACE('',(#2236),#14351,.F.);
#15205=ADVANCED_FACE('',(#2237),#14352,.T.);
#15206=ADVANCED_FACE('',(#2238),#14353,.T.);
#15207=ADVANCED_FACE('',(#2239),#14354,.T.);
#15208=ADVANCED_FACE('',(#2240),#14355,.T.);
#15209=ADVANCED_FACE('',(#2241),#14356,.F.);
#15210=ADVANCED_FACE('',(#2242),#14357,.T.);
#15211=ADVANCED_FACE('',(#2243),#14358,.T.);
#15212=ADVANCED_FACE('',(#2244),#14359,.T.);
#15213=ADVANCED_FACE('',(#2245),#14360,.T.);
#15214=ADVANCED_FACE('',(#2246),#14361,.T.);
#15215=ADVANCED_FACE('',(#2247),#14362,.F.);
#15216=ADVANCED_FACE('',(#2248),#14363,.T.);
#15217=ADVANCED_FACE('',(#2249),#14364,.T.);
#15218=ADVANCED_FACE('',(#2250),#14365,.T.);
#15219=ADVANCED_FACE('',(#2251),#14366,.T.);
#15220=ADVANCED_FACE('',(#2252),#14367,.T.);
#15221=ADVANCED_FACE('',(#2253),#14368,.F.);
#15222=ADVANCED_FACE('',(#2254),#14369,.T.);
#15223=ADVANCED_FACE('',(#2255),#1271,.F.);
#15224=ADVANCED_FACE('',(#2256),#1272,.F.);
#15225=ADVANCED_FACE('',(#2257),#1273,.F.);
#15226=ADVANCED_FACE('',(#2258),#1274,.F.);
#15227=ADVANCED_FACE('',(#2259,#1643,#1644,#1645,#1646),#14370,.F.);
#15228=ADVANCED_FACE('',(#2260,#1647,#1648,#1649,#1650),#14371,.T.);
#15229=ADVANCED_FACE('',(#2261),#14372,.F.);
#15230=ADVANCED_FACE('',(#2262),#14373,.F.);
#15231=ADVANCED_FACE('',(#2263),#14374,.F.);
#15232=ADVANCED_FACE('',(#2264),#14375,.F.);
#15233=ADVANCED_FACE('',(#2265),#1275,.F.);
#15234=ADVANCED_FACE('',(#2266),#1276,.F.);
#15235=ADVANCED_FACE('',(#2267),#1277,.F.);
#15236=ADVANCED_FACE('',(#2268),#1278,.F.);
#15237=ADVANCED_FACE('',(#2269),#1279,.F.);
#15238=ADVANCED_FACE('',(#2270),#1280,.F.);
#15239=ADVANCED_FACE('',(#2271),#14376,.T.);
#15240=ADVANCED_FACE('',(#2272),#14377,.T.);
#15241=ADVANCED_FACE('',(#2273),#14378,.T.);
#15242=ADVANCED_FACE('',(#2274),#14379,.T.);
#15243=ADVANCED_FACE('',(#2275,#1651,#1652,#1653,#1654,#1655,#1656),#14380,
 .F.);
#15244=ADVANCED_FACE('',(#2276,#1657,#1658,#1659,#1660,#1661,#1662),#14381,
 .T.);
#15245=ADVANCED_FACE('',(#2277),#14382,.F.);
#15246=ADVANCED_FACE('',(#2278),#14383,.F.);
#15247=ADVANCED_FACE('',(#2279),#14384,.F.);
#15248=ADVANCED_FACE('',(#2280),#14385,.F.);
#15249=ADVANCED_FACE('',(#2281),#14386,.F.);
#15250=ADVANCED_FACE('',(#2282),#14387,.F.);
#15251=ADVANCED_FACE('',(#2283),#14388,.F.);
#15252=ADVANCED_FACE('',(#2284),#14389,.F.);
#15253=ADVANCED_FACE('',(#2285),#14390,.T.);
#15254=ADVANCED_FACE('',(#2286),#14391,.F.);
#15255=ADVANCED_FACE('',(#2287),#14392,.F.);
#15256=ADVANCED_FACE('',(#2288),#14393,.F.);
#15257=ADVANCED_FACE('',(#2289),#14394,.F.);
#15258=ADVANCED_FACE('',(#2290),#14395,.F.);
#15259=ADVANCED_FACE('',(#2291),#14396,.F.);
#15260=ADVANCED_FACE('',(#2292),#14397,.F.);
#15261=ADVANCED_FACE('',(#2293),#14398,.F.);
#15262=ADVANCED_FACE('',(#2294),#14399,.T.);
#15263=ADVANCED_FACE('',(#2295),#14400,.F.);
#15264=ADVANCED_FACE('',(#2296),#14401,.F.);
#15265=ADVANCED_FACE('',(#2297),#14402,.F.);
#15266=ADVANCED_FACE('',(#2298),#14403,.F.);
#15267=ADVANCED_FACE('',(#2299),#14404,.F.);
#15268=ADVANCED_FACE('',(#2300),#14405,.F.);
#15269=ADVANCED_FACE('',(#2301),#14406,.F.);
#15270=ADVANCED_FACE('',(#2302),#14407,.F.);
#15271=ADVANCED_FACE('',(#2303),#14408,.T.);
#15272=ADVANCED_FACE('',(#2304),#14409,.T.);
#15273=ADVANCED_FACE('',(#2305),#14410,.T.);
#15274=ADVANCED_FACE('',(#2306),#14411,.T.);
#15275=ADVANCED_FACE('',(#2307),#14412,.T.);
#15276=ADVANCED_FACE('',(#2308),#14413,.T.);
#15277=ADVANCED_FACE('',(#2309),#14414,.T.);
#15278=ADVANCED_FACE('',(#2310),#14415,.T.);
#15279=ADVANCED_FACE('',(#2311),#14416,.T.);
#15280=ADVANCED_FACE('',(#2312),#14417,.F.);
#15281=ADVANCED_FACE('',(#2313),#14418,.T.);
#15282=ADVANCED_FACE('',(#2314),#14419,.T.);
#15283=ADVANCED_FACE('',(#2315),#14420,.T.);
#15284=ADVANCED_FACE('',(#2316),#14421,.T.);
#15285=ADVANCED_FACE('',(#2317),#14422,.T.);
#15286=ADVANCED_FACE('',(#2318),#14423,.T.);
#15287=ADVANCED_FACE('',(#2319),#14424,.T.);
#15288=ADVANCED_FACE('',(#2320),#14425,.T.);
#15289=ADVANCED_FACE('',(#2321),#14426,.F.);
#15290=ADVANCED_FACE('',(#2322),#14427,.T.);
#15291=ADVANCED_FACE('',(#2323),#14428,.T.);
#15292=ADVANCED_FACE('',(#2324),#14429,.T.);
#15293=ADVANCED_FACE('',(#2325),#14430,.T.);
#15294=ADVANCED_FACE('',(#2326),#14431,.T.);
#15295=ADVANCED_FACE('',(#2327),#14432,.T.);
#15296=ADVANCED_FACE('',(#2328),#14433,.T.);
#15297=ADVANCED_FACE('',(#2329),#14434,.T.);
#15298=ADVANCED_FACE('',(#2330),#14435,.F.);
#15299=ADVANCED_FACE('',(#2331),#14436,.T.);
#15300=ADVANCED_FACE('',(#2332),#14437,.T.);
#15301=ADVANCED_FACE('',(#2333),#14438,.T.);
#15302=ADVANCED_FACE('',(#2334),#14439,.T.);
#15303=ADVANCED_FACE('',(#2335),#14440,.T.);
#15304=ADVANCED_FACE('',(#2336),#14441,.T.);
#15305=ADVANCED_FACE('',(#2337),#14442,.T.);
#15306=ADVANCED_FACE('',(#2338),#14443,.T.);
#15307=ADVANCED_FACE('',(#2339),#14444,.F.);
#15308=ADVANCED_FACE('',(#2340),#14445,.T.);
#15309=ADVANCED_FACE('',(#2341),#14446,.T.);
#15310=ADVANCED_FACE('',(#2342),#14447,.T.);
#15311=ADVANCED_FACE('',(#2343),#14448,.T.);
#15312=ADVANCED_FACE('',(#2344),#14449,.T.);
#15313=ADVANCED_FACE('',(#2345),#14450,.T.);
#15314=ADVANCED_FACE('',(#2346),#14451,.T.);
#15315=ADVANCED_FACE('',(#2347),#14452,.T.);
#15316=ADVANCED_FACE('',(#2348),#14453,.F.);
#15317=ADVANCED_FACE('',(#2349),#14454,.F.);
#15318=ADVANCED_FACE('',(#2350),#14455,.F.);
#15319=ADVANCED_FACE('',(#2351),#14456,.F.);
#15320=ADVANCED_FACE('',(#2352),#14457,.F.);
#15321=ADVANCED_FACE('',(#2353),#14458,.F.);
#15322=ADVANCED_FACE('',(#2354),#14459,.F.);
#15323=ADVANCED_FACE('',(#2355),#14460,.F.);
#15324=ADVANCED_FACE('',(#2356),#14461,.F.);
#15325=ADVANCED_FACE('',(#2357),#14462,.T.);
#15326=ADVANCED_FACE('',(#2358),#14463,.F.);
#15327=ADVANCED_FACE('',(#2359),#14464,.F.);
#15328=ADVANCED_FACE('',(#2360),#14465,.F.);
#15329=ADVANCED_FACE('',(#2361),#14466,.F.);
#15330=ADVANCED_FACE('',(#2362),#14467,.F.);
#15331=ADVANCED_FACE('',(#2363),#14468,.F.);
#15332=ADVANCED_FACE('',(#2364),#14469,.F.);
#15333=ADVANCED_FACE('',(#2365),#14470,.F.);
#15334=ADVANCED_FACE('',(#2366),#14471,.T.);
#15335=ADVANCED_FACE('',(#2367),#14472,.F.);
#15336=ADVANCED_FACE('',(#2368),#14473,.F.);
#15337=ADVANCED_FACE('',(#2369),#14474,.F.);
#15338=ADVANCED_FACE('',(#2370),#14475,.F.);
#15339=ADVANCED_FACE('',(#2371),#14476,.F.);
#15340=ADVANCED_FACE('',(#2372),#14477,.F.);
#15341=ADVANCED_FACE('',(#2373),#14478,.F.);
#15342=ADVANCED_FACE('',(#2374),#14479,.F.);
#15343=ADVANCED_FACE('',(#2375),#14480,.T.);
#15344=ADVANCED_FACE('',(#2376),#1281,.F.);
#15345=ADVANCED_FACE('',(#2377),#1282,.F.);
#15346=ADVANCED_FACE('',(#2378),#1283,.F.);
#15347=ADVANCED_FACE('',(#2379),#1284,.F.);
#15348=ADVANCED_FACE('',(#2380,#1663,#1664,#1665,#1666),#14481,.F.);
#15349=ADVANCED_FACE('',(#2381,#1667,#1668,#1669,#1670),#14482,.T.);
#15350=ADVANCED_FACE('',(#2382),#14483,.F.);
#15351=ADVANCED_FACE('',(#2383),#14484,.F.);
#15352=ADVANCED_FACE('',(#2384),#14485,.F.);
#15353=ADVANCED_FACE('',(#2385),#14486,.F.);
#15354=ADVANCED_FACE('',(#2386),#14487,.F.);
#15355=ADVANCED_FACE('',(#2387),#14488,.F.);
#15356=ADVANCED_FACE('',(#2388),#14489,.F.);
#15357=ADVANCED_FACE('',(#2389),#14490,.F.);
#15358=ADVANCED_FACE('',(#2390),#14491,.T.);
#15359=ADVANCED_FACE('',(#2391),#14492,.F.);
#15360=ADVANCED_FACE('',(#2392),#14493,.F.);
#15361=ADVANCED_FACE('',(#2393),#14494,.F.);
#15362=ADVANCED_FACE('',(#2394),#14495,.F.);
#15363=ADVANCED_FACE('',(#2395),#14496,.F.);
#15364=ADVANCED_FACE('',(#2396),#14497,.T.);
#15365=ADVANCED_FACE('',(#2397),#14498,.F.);
#15366=ADVANCED_FACE('',(#2398),#14499,.F.);
#15367=ADVANCED_FACE('',(#2399),#14500,.F.);
#15368=ADVANCED_FACE('',(#2400),#14501,.F.);
#15369=ADVANCED_FACE('',(#2401),#14502,.F.);
#15370=ADVANCED_FACE('',(#2402),#14503,.T.);
#15371=ADVANCED_FACE('',(#2403),#14504,.F.);
#15372=ADVANCED_FACE('',(#2404),#14505,.F.);
#15373=ADVANCED_FACE('',(#2405),#14506,.F.);
#15374=ADVANCED_FACE('',(#2406),#14507,.F.);
#15375=ADVANCED_FACE('',(#2407),#14508,.F.);
#15376=ADVANCED_FACE('',(#2408),#14509,.T.);
#15377=ADVANCED_FACE('',(#2409),#14510,.F.);
#15378=ADVANCED_FACE('',(#2410),#14511,.F.);
#15379=ADVANCED_FACE('',(#2411),#14512,.F.);
#15380=ADVANCED_FACE('',(#2412),#14513,.F.);
#15381=ADVANCED_FACE('',(#2413),#14514,.F.);
#15382=ADVANCED_FACE('',(#2414),#14515,.T.);
#15383=ADVANCED_FACE('',(#2415),#14516,.F.);
#15384=ADVANCED_FACE('',(#2416),#14517,.F.);
#15385=ADVANCED_FACE('',(#2417),#14518,.F.);
#15386=ADVANCED_FACE('',(#2418),#14519,.F.);
#15387=ADVANCED_FACE('',(#2419),#14520,.F.);
#15388=ADVANCED_FACE('',(#2420),#14521,.T.);
#15389=ADVANCED_FACE('',(#2421),#14522,.F.);
#15390=ADVANCED_FACE('',(#2422),#14523,.F.);
#15391=ADVANCED_FACE('',(#2423),#14524,.F.);
#15392=ADVANCED_FACE('',(#2424),#14525,.F.);
#15393=ADVANCED_FACE('',(#2425),#14526,.F.);
#15394=ADVANCED_FACE('',(#2426),#14527,.T.);
#15395=ADVANCED_FACE('',(#2427),#14528,.F.);
#15396=ADVANCED_FACE('',(#2428),#14529,.F.);
#15397=ADVANCED_FACE('',(#2429),#14530,.F.);
#15398=ADVANCED_FACE('',(#2430),#14531,.F.);
#15399=ADVANCED_FACE('',(#2431),#14532,.F.);
#15400=ADVANCED_FACE('',(#2432),#14533,.T.);
#15401=ADVANCED_FACE('',(#2433),#14534,.F.);
#15402=ADVANCED_FACE('',(#2434),#14535,.F.);
#15403=ADVANCED_FACE('',(#2435),#14536,.F.);
#15404=ADVANCED_FACE('',(#2436),#14537,.F.);
#15405=ADVANCED_FACE('',(#2437),#14538,.F.);
#15406=ADVANCED_FACE('',(#2438),#14539,.T.);
#15407=ADVANCED_FACE('',(#2439),#14540,.F.);
#15408=ADVANCED_FACE('',(#2440),#14541,.F.);
#15409=ADVANCED_FACE('',(#2441),#14542,.F.);
#15410=ADVANCED_FACE('',(#2442),#14543,.F.);
#15411=ADVANCED_FACE('',(#2443),#14544,.F.);
#15412=ADVANCED_FACE('',(#2444),#14545,.T.);
#15413=ADVANCED_FACE('',(#2445),#14546,.F.);
#15414=ADVANCED_FACE('',(#2446),#14547,.F.);
#15415=ADVANCED_FACE('',(#2447),#14548,.F.);
#15416=ADVANCED_FACE('',(#2448),#14549,.F.);
#15417=ADVANCED_FACE('',(#2449),#14550,.F.);
#15418=ADVANCED_FACE('',(#2450),#14551,.T.);
#15419=ADVANCED_FACE('',(#2451),#14552,.F.);
#15420=ADVANCED_FACE('',(#2452),#14553,.F.);
#15421=ADVANCED_FACE('',(#2453),#14554,.F.);
#15422=ADVANCED_FACE('',(#2454),#14555,.F.);
#15423=ADVANCED_FACE('',(#2455),#14556,.F.);
#15424=ADVANCED_FACE('',(#2456),#14557,.T.);
#15425=ADVANCED_FACE('',(#2457),#14558,.F.);
#15426=ADVANCED_FACE('',(#2458),#14559,.F.);
#15427=ADVANCED_FACE('',(#2459),#14560,.F.);
#15428=ADVANCED_FACE('',(#2460),#14561,.F.);
#15429=ADVANCED_FACE('',(#2461),#14562,.F.);
#15430=ADVANCED_FACE('',(#2462),#14563,.T.);
#15431=ADVANCED_FACE('',(#2463),#14564,.F.);
#15432=ADVANCED_FACE('',(#2464),#14565,.F.);
#15433=ADVANCED_FACE('',(#2465),#14566,.F.);
#15434=ADVANCED_FACE('',(#2466),#14567,.F.);
#15435=ADVANCED_FACE('',(#2467),#14568,.F.);
#15436=ADVANCED_FACE('',(#2468),#14569,.T.);
#15437=ADVANCED_FACE('',(#2469),#14570,.F.);
#15438=ADVANCED_FACE('',(#2470),#14571,.F.);
#15439=ADVANCED_FACE('',(#2471),#14572,.F.);
#15440=ADVANCED_FACE('',(#2472),#14573,.F.);
#15441=ADVANCED_FACE('',(#2473),#14574,.F.);
#15442=ADVANCED_FACE('',(#2474),#14575,.T.);
#15443=ADVANCED_FACE('',(#2475),#14576,.F.);
#15444=ADVANCED_FACE('',(#2476),#14577,.F.);
#15445=ADVANCED_FACE('',(#2477),#14578,.F.);
#15446=ADVANCED_FACE('',(#2478),#14579,.F.);
#15447=ADVANCED_FACE('',(#2479),#14580,.F.);
#15448=ADVANCED_FACE('',(#2480),#14581,.T.);
#15449=ADVANCED_FACE('',(#2481),#14582,.F.);
#15450=ADVANCED_FACE('',(#2482),#14583,.F.);
#15451=ADVANCED_FACE('',(#2483),#14584,.F.);
#15452=ADVANCED_FACE('',(#2484),#14585,.F.);
#15453=ADVANCED_FACE('',(#2485),#14586,.F.);
#15454=ADVANCED_FACE('',(#2486),#14587,.T.);
#15455=ADVANCED_FACE('',(#2487),#14588,.F.);
#15456=ADVANCED_FACE('',(#2488),#14589,.F.);
#15457=ADVANCED_FACE('',(#2489),#14590,.F.);
#15458=ADVANCED_FACE('',(#2490),#14591,.F.);
#15459=ADVANCED_FACE('',(#2491),#14592,.F.);
#15460=ADVANCED_FACE('',(#2492),#14593,.T.);
#15461=ADVANCED_FACE('',(#2493),#14594,.F.);
#15462=ADVANCED_FACE('',(#2494),#14595,.F.);
#15463=ADVANCED_FACE('',(#2495),#14596,.F.);
#15464=ADVANCED_FACE('',(#2496),#14597,.F.);
#15465=ADVANCED_FACE('',(#2497),#14598,.F.);
#15466=ADVANCED_FACE('',(#2498),#14599,.F.);
#15467=ADVANCED_FACE('',(#2499),#14600,.T.);
#15468=ADVANCED_FACE('',(#2500),#14601,.F.);
#15469=ADVANCED_FACE('',(#2501),#14602,.F.);
#15470=ADVANCED_FACE('',(#2502),#14603,.F.);
#15471=ADVANCED_FACE('',(#2503),#14604,.F.);
#15472=ADVANCED_FACE('',(#2504),#14605,.F.);
#15473=ADVANCED_FACE('',(#2505),#14606,.T.);
#15474=ADVANCED_FACE('',(#2506),#14607,.F.);
#15475=ADVANCED_FACE('',(#2507),#14608,.F.);
#15476=ADVANCED_FACE('',(#2508),#14609,.F.);
#15477=ADVANCED_FACE('',(#2509),#14610,.F.);
#15478=ADVANCED_FACE('',(#2510),#14611,.T.);
#15479=ADVANCED_FACE('',(#2511),#14612,.F.);
#15480=ADVANCED_FACE('',(#2512),#14613,.F.);
#15481=ADVANCED_FACE('',(#2513),#14614,.F.);
#15482=ADVANCED_FACE('',(#2514),#14615,.F.);
#15483=ADVANCED_FACE('',(#2515),#14616,.F.);
#15484=ADVANCED_FACE('',(#2516),#14617,.T.);
#15485=ADVANCED_FACE('',(#2517),#14618,.F.);
#15573=CLOSED_SHELL('',(#15098,#15099,#15100,#15101,#15102,#15103));
#15574=CLOSED_SHELL('',(#15104,#15105,#15106,#15107,#15108,#15109,#15110,
#15111,#15112));
#15575=CLOSED_SHELL('',(#15113,#15114,#15115,#15116,#15117,#15118,#15119,
#15120,#15121));
#15576=CLOSED_SHELL('',(#15122,#15123,#15124,#15125,#15126,#15127,#15128,
#15129,#15130,#15131,#15132,#15133,#15134,#15135,#15136));
#15577=CLOSED_SHELL('',(#15137,#15138,#15139,#15140,#15141,#15142));
#15578=CLOSED_SHELL('',(#15143,#15144,#15145,#15146,#15147,#15148));
#15579=CLOSED_SHELL('',(#15149,#15150,#15151,#15152,#15153,#15154,#15155,
#15156));
#15580=CLOSED_SHELL('',(#15157,#15158,#15159,#15160,#15161,#15162,#15163,
#15164,#15165));
#15581=CLOSED_SHELL('',(#15166,#15167,#15168,#15169,#15170,#15171,#15172,
#15173,#15174));
#15582=CLOSED_SHELL('',(#15175,#15176,#15177,#15178,#15179,#15180,#15181,
#15182,#15183));
#15583=CLOSED_SHELL('',(#15184,#15185,#15186,#15187,#15188,#15189,#15190,
#15191,#15192));
#15584=CLOSED_SHELL('',(#15193,#15194,#15195,#15196,#15197,#15198));
#15585=CLOSED_SHELL('',(#15199,#15200,#15201,#15202,#15203,#15204));
#15586=CLOSED_SHELL('',(#15205,#15206,#15207,#15208,#15209,#15210));
#15587=CLOSED_SHELL('',(#15211,#15212,#15213,#15214,#15215,#15216));
#15588=CLOSED_SHELL('',(#15217,#15218,#15219,#15220,#15221,#15222));
#15589=CLOSED_SHELL('',(#15223,#15224,#15225,#15226,#15227,#15228,#15229,
#15230,#15231,#15232));
#15590=CLOSED_SHELL('',(#15233,#15234,#15235,#15236,#15237,#15238,#15239,
#15240,#15241,#15242,#15243,#15244));
#15591=CLOSED_SHELL('',(#15245,#15246,#15247,#15248,#15249,#15250,#15251,
#15252,#15253));
#15592=CLOSED_SHELL('',(#15254,#15255,#15256,#15257,#15258,#15259,#15260,
#15261,#15262));
#15593=CLOSED_SHELL('',(#15263,#15264,#15265,#15266,#15267,#15268,#15269,
#15270,#15271));
#15594=CLOSED_SHELL('',(#15272,#15273,#15274,#15275,#15276,#15277,#15278,
#15279,#15280));
#15595=CLOSED_SHELL('',(#15281,#15282,#15283,#15284,#15285,#15286,#15287,
#15288,#15289));
#15596=CLOSED_SHELL('',(#15290,#15291,#15292,#15293,#15294,#15295,#15296,
#15297,#15298));
#15597=CLOSED_SHELL('',(#15299,#15300,#15301,#15302,#15303,#15304,#15305,
#15306,#15307));
#15598=CLOSED_SHELL('',(#15308,#15309,#15310,#15311,#15312,#15313,#15314,
#15315,#15316));
#15599=CLOSED_SHELL('',(#15317,#15318,#15319,#15320,#15321,#15322,#15323,
#15324,#15325));
#15600=CLOSED_SHELL('',(#15326,#15327,#15328,#15329,#15330,#15331,#15332,
#15333,#15334));
#15601=CLOSED_SHELL('',(#15335,#15336,#15337,#15338,#15339,#15340,#15341,
#15342,#15343));
#15602=CLOSED_SHELL('',(#15344,#15345,#15346,#15347,#15348,#15349,#15350,
#15351,#15352,#15353));
#15603=CLOSED_SHELL('',(#15354,#15355,#15356,#15357,#15358,#15359));
#15604=CLOSED_SHELL('',(#15360,#15361,#15362,#15363,#15364,#15365));
#15605=CLOSED_SHELL('',(#15366,#15367,#15368,#15369,#15370,#15371));
#15606=CLOSED_SHELL('',(#15372,#15373,#15374,#15375,#15376,#15377));
#15607=CLOSED_SHELL('',(#15378,#15379,#15380,#15381,#15382,#15383));
#15608=CLOSED_SHELL('',(#15384,#15385,#15386,#15387,#15388,#15389));
#15609=CLOSED_SHELL('',(#15390,#15391,#15392,#15393,#15394,#15395));
#15610=CLOSED_SHELL('',(#15396,#15397,#15398,#15399,#15400,#15401));
#15611=CLOSED_SHELL('',(#15402,#15403,#15404,#15405,#15406,#15407));
#15612=CLOSED_SHELL('',(#15408,#15409,#15410,#15411,#15412,#15413));
#15613=CLOSED_SHELL('',(#15414,#15415,#15416,#15417,#15418,#15419));
#15614=CLOSED_SHELL('',(#15420,#15421,#15422,#15423,#15424,#15425));
#15615=CLOSED_SHELL('',(#15426,#15427,#15428,#15429,#15430,#15431));
#15616=CLOSED_SHELL('',(#15432,#15433,#15434,#15435,#15436,#15437));
#15617=CLOSED_SHELL('',(#15438,#15439,#15440,#15441,#15442,#15443));
#15618=CLOSED_SHELL('',(#15444,#15445,#15446,#15447,#15448,#15449));
#15619=CLOSED_SHELL('',(#15450,#15451,#15452,#15453,#15454,#15455));
#15620=CLOSED_SHELL('',(#15456,#15457,#15458,#15459,#15460,#15461));
#15621=CLOSED_SHELL('',(#15462,#15463,#15464,#15465,#15466,#15467));
#15622=CLOSED_SHELL('',(#15468,#15469,#15470,#15471,#15472,#15473));
#15623=CLOSED_SHELL('',(#15474,#15475,#15476,#15477,#15478,#15479));
#15624=CLOSED_SHELL('',(#15480,#15481,#15482,#15483,#15484,#15485));
#16548=AXIS2_PLACEMENT_3D('',#30705,#19276,#19277);
#16549=AXIS2_PLACEMENT_3D('',#30706,#19278,#19279);
#16550=AXIS2_PLACEMENT_3D('',#30715,#19284,#19285);
#16551=AXIS2_PLACEMENT_3D('',#30721,#19289,#19290);
#16552=AXIS2_PLACEMENT_3D('',#30727,#19294,#19295);
#16553=AXIS2_PLACEMENT_3D('',#30730,#19298,#19299);
#16554=AXIS2_PLACEMENT_3D('',#30731,#19300,#19301);
#16555=AXIS2_PLACEMENT_3D('',#30732,#19302,#19303);
#16556=AXIS2_PLACEMENT_3D('',#30734,#19304,#19305);
#16557=AXIS2_PLACEMENT_3D('',#30737,#19307,#19308);
#16558=AXIS2_PLACEMENT_3D('',#30738,#19309,#19310);
#16559=AXIS2_PLACEMENT_3D('',#30749,#19315,#19316);
#16560=AXIS2_PLACEMENT_3D('',#30751,#19318,#19319);
#16561=AXIS2_PLACEMENT_3D('',#30758,#19322,#19323);
#16562=AXIS2_PLACEMENT_3D('',#30764,#19327,#19328);
#16563=AXIS2_PLACEMENT_3D('',#30767,#19331,#19332);
#16564=AXIS2_PLACEMENT_3D('',#30769,#19334,#19335);
#16565=AXIS2_PLACEMENT_3D('',#30771,#19337,#19338);
#16566=AXIS2_PLACEMENT_3D('',#30773,#19340,#19341);
#16567=AXIS2_PLACEMENT_3D('',#30775,#19343,#19344);
#16568=AXIS2_PLACEMENT_3D('',#30776,#19345,#19346);
#16569=AXIS2_PLACEMENT_3D('',#30778,#19347,#19348);
#16570=AXIS2_PLACEMENT_3D('',#30781,#19350,#19351);
#16571=AXIS2_PLACEMENT_3D('',#30782,#19352,#19353);
#16572=AXIS2_PLACEMENT_3D('',#30789,#19356,#19357);
#16573=AXIS2_PLACEMENT_3D('',#30795,#19361,#19362);
#16574=AXIS2_PLACEMENT_3D('',#30806,#19367,#19368);
#16575=AXIS2_PLACEMENT_3D('',#30808,#19370,#19371);
#16576=AXIS2_PLACEMENT_3D('',#30811,#19374,#19375);
#16577=AXIS2_PLACEMENT_3D('',#30813,#19377,#19378);
#16578=AXIS2_PLACEMENT_3D('',#30815,#19380,#19381);
#16579=AXIS2_PLACEMENT_3D('',#30817,#19383,#19384);
#16580=AXIS2_PLACEMENT_3D('',#30819,#19386,#19387);
#16581=AXIS2_PLACEMENT_3D('',#30820,#19388,#19389);
#16582=AXIS2_PLACEMENT_3D('',#30822,#19390,#19391);
#16583=AXIS2_PLACEMENT_3D('',#30825,#19393,#19394);
#16584=AXIS2_PLACEMENT_3D('',#30826,#19395,#19396);
#16585=AXIS2_PLACEMENT_3D('',#30828,#19397,#19398);
#16586=AXIS2_PLACEMENT_3D('',#30831,#19400,#19401);
#16587=AXIS2_PLACEMENT_3D('',#30832,#19402,#19403);
#16588=AXIS2_PLACEMENT_3D('',#30834,#19404,#19405);
#16589=AXIS2_PLACEMENT_3D('',#30837,#19407,#19408);
#16590=AXIS2_PLACEMENT_3D('',#30838,#19409,#19410);
#16591=AXIS2_PLACEMENT_3D('',#30840,#19411,#19412);
#16592=AXIS2_PLACEMENT_3D('',#30843,#19414,#19415);
#16593=AXIS2_PLACEMENT_3D('',#30844,#19416,#19417);
#16594=AXIS2_PLACEMENT_3D('',#30846,#19418,#19419);
#16595=AXIS2_PLACEMENT_3D('',#30849,#19421,#19422);
#16596=AXIS2_PLACEMENT_3D('',#30850,#19423,#19424);
#16597=AXIS2_PLACEMENT_3D('',#30867,#19433,#19434);
#16598=AXIS2_PLACEMENT_3D('',#30884,#19443,#19444);
#16599=AXIS2_PLACEMENT_3D('',#30887,#19447,#19448);
#16600=AXIS2_PLACEMENT_3D('',#30889,#19450,#19451);
#16601=AXIS2_PLACEMENT_3D('',#30891,#19453,#19454);
#16602=AXIS2_PLACEMENT_3D('',#30893,#19456,#19457);
#16603=AXIS2_PLACEMENT_3D('',#30895,#19459,#19460);
#16604=AXIS2_PLACEMENT_3D('',#30897,#19462,#19463);
#16605=AXIS2_PLACEMENT_3D('',#30899,#19465,#19466);
#16606=AXIS2_PLACEMENT_3D('',#30900,#19467,#19468);
#16607=AXIS2_PLACEMENT_3D('',#30909,#19473,#19474);
#16608=AXIS2_PLACEMENT_3D('',#30915,#19478,#19479);
#16609=AXIS2_PLACEMENT_3D('',#30921,#19483,#19484);
#16610=AXIS2_PLACEMENT_3D('',#30924,#19487,#19488);
#16611=AXIS2_PLACEMENT_3D('',#30925,#19489,#19490);
#16612=AXIS2_PLACEMENT_3D('',#30926,#19491,#19492);
#16613=AXIS2_PLACEMENT_3D('',#30935,#19497,#19498);
#16614=AXIS2_PLACEMENT_3D('',#30941,#19502,#19503);
#16615=AXIS2_PLACEMENT_3D('',#30947,#19507,#19508);
#16616=AXIS2_PLACEMENT_3D('',#30950,#19511,#19512);
#16617=AXIS2_PLACEMENT_3D('',#30951,#19513,#19514);
#16618=AXIS2_PLACEMENT_3D('',#30952,#19515,#19516);
#16619=AXIS2_PLACEMENT_3D('',#30961,#19521,#19522);
#16620=AXIS2_PLACEMENT_3D('',#30967,#19526,#19527);
#16621=AXIS2_PLACEMENT_3D('',#30973,#19531,#19532);
#16622=AXIS2_PLACEMENT_3D('',#30979,#19536,#19537);
#16623=AXIS2_PLACEMENT_3D('',#30985,#19541,#19542);
#16624=AXIS2_PLACEMENT_3D('',#30988,#19545,#19546);
#16625=AXIS2_PLACEMENT_3D('',#30989,#19547,#19548);
#16626=AXIS2_PLACEMENT_3D('',#30990,#19549,#19550);
#16627=AXIS2_PLACEMENT_3D('',#30992,#19551,#19552);
#16628=AXIS2_PLACEMENT_3D('',#30995,#19554,#19555);
#16629=AXIS2_PLACEMENT_3D('',#30996,#19556,#19557);
#16630=AXIS2_PLACEMENT_3D('',#30998,#19558,#19559);
#16631=AXIS2_PLACEMENT_3D('',#31001,#19561,#19562);
#16632=AXIS2_PLACEMENT_3D('',#31002,#19563,#19564);
#16633=AXIS2_PLACEMENT_3D('',#31004,#19565,#19566);
#16634=AXIS2_PLACEMENT_3D('',#31007,#19568,#19569);
#16635=AXIS2_PLACEMENT_3D('',#31008,#19570,#19571);
#16636=AXIS2_PLACEMENT_3D('',#31017,#19576,#19577);
#16637=AXIS2_PLACEMENT_3D('',#31026,#19582,#19583);
#16638=AXIS2_PLACEMENT_3D('',#31029,#19586,#19587);
#16639=AXIS2_PLACEMENT_3D('',#31031,#19589,#19590);
#16640=AXIS2_PLACEMENT_3D('',#31033,#19592,#19593);
#16641=AXIS2_PLACEMENT_3D('',#31034,#19594,#19595);
#16642=AXIS2_PLACEMENT_3D('',#31036,#19596,#19597);
#16643=AXIS2_PLACEMENT_3D('',#31039,#19599,#19600);
#16644=AXIS2_PLACEMENT_3D('',#31040,#19601,#19602);
#16645=AXIS2_PLACEMENT_3D('',#31042,#19603,#19604);
#16646=AXIS2_PLACEMENT_3D('',#31045,#19606,#19607);
#16647=AXIS2_PLACEMENT_3D('',#31046,#19608,#19609);
#16648=AXIS2_PLACEMENT_3D('',#31048,#19610,#19611);
#16649=AXIS2_PLACEMENT_3D('',#31051,#19613,#19614);
#16650=AXIS2_PLACEMENT_3D('',#31052,#19615,#19616);
#16651=AXIS2_PLACEMENT_3D('',#31061,#19621,#19622);
#16652=AXIS2_PLACEMENT_3D('',#31070,#19627,#19628);
#16653=AXIS2_PLACEMENT_3D('',#31073,#19631,#19632);
#16654=AXIS2_PLACEMENT_3D('',#31075,#19634,#19635);
#16655=AXIS2_PLACEMENT_3D('',#31077,#19637,#19638);
#16656=AXIS2_PLACEMENT_3D('',#31078,#19639,#19640);
#16657=AXIS2_PLACEMENT_3D('',#31080,#19641,#19642);
#16658=AXIS2_PLACEMENT_3D('',#31083,#19644,#19645);
#16659=AXIS2_PLACEMENT_3D('',#31084,#19646,#19647);
#16660=AXIS2_PLACEMENT_3D('',#31086,#19648,#19649);
#16661=AXIS2_PLACEMENT_3D('',#31089,#19651,#19652);
#16662=AXIS2_PLACEMENT_3D('',#31090,#19653,#19654);
#16663=AXIS2_PLACEMENT_3D('',#31092,#19655,#19656);
#16664=AXIS2_PLACEMENT_3D('',#31095,#19658,#19659);
#16665=AXIS2_PLACEMENT_3D('',#31096,#19660,#19661);
#16666=AXIS2_PLACEMENT_3D('',#31105,#19666,#19667);
#16667=AXIS2_PLACEMENT_3D('',#31114,#19672,#19673);
#16668=AXIS2_PLACEMENT_3D('',#31117,#19676,#19677);
#16669=AXIS2_PLACEMENT_3D('',#31119,#19679,#19680);
#16670=AXIS2_PLACEMENT_3D('',#31121,#19682,#19683);
#16671=AXIS2_PLACEMENT_3D('',#31122,#19684,#19685);
#16672=AXIS2_PLACEMENT_3D('',#31124,#19686,#19687);
#16673=AXIS2_PLACEMENT_3D('',#31127,#19689,#19690);
#16674=AXIS2_PLACEMENT_3D('',#31128,#19691,#19692);
#16675=AXIS2_PLACEMENT_3D('',#31130,#19693,#19694);
#16676=AXIS2_PLACEMENT_3D('',#31133,#19696,#19697);
#16677=AXIS2_PLACEMENT_3D('',#31134,#19698,#19699);
#16678=AXIS2_PLACEMENT_3D('',#31136,#19700,#19701);
#16679=AXIS2_PLACEMENT_3D('',#31139,#19703,#19704);
#16680=AXIS2_PLACEMENT_3D('',#31140,#19705,#19706);
#16681=AXIS2_PLACEMENT_3D('',#31149,#19711,#19712);
#16682=AXIS2_PLACEMENT_3D('',#31158,#19717,#19718);
#16683=AXIS2_PLACEMENT_3D('',#31161,#19721,#19722);
#16684=AXIS2_PLACEMENT_3D('',#31163,#19724,#19725);
#16685=AXIS2_PLACEMENT_3D('',#31165,#19727,#19728);
#16686=AXIS2_PLACEMENT_3D('',#31166,#19729,#19730);
#16687=AXIS2_PLACEMENT_3D('',#31175,#19735,#19736);
#16688=AXIS2_PLACEMENT_3D('',#31181,#19740,#19741);
#16689=AXIS2_PLACEMENT_3D('',#31187,#19745,#19746);
#16690=AXIS2_PLACEMENT_3D('',#31190,#19749,#19750);
#16691=AXIS2_PLACEMENT_3D('',#31191,#19751,#19752);
#16692=AXIS2_PLACEMENT_3D('',#31192,#19753,#19754);
#16693=AXIS2_PLACEMENT_3D('',#31201,#19759,#19760);
#16694=AXIS2_PLACEMENT_3D('',#31207,#19764,#19765);
#16695=AXIS2_PLACEMENT_3D('',#31213,#19769,#19770);
#16696=AXIS2_PLACEMENT_3D('',#31216,#19773,#19774);
#16697=AXIS2_PLACEMENT_3D('',#31217,#19775,#19776);
#16698=AXIS2_PLACEMENT_3D('',#31218,#19777,#19778);
#16699=AXIS2_PLACEMENT_3D('',#31227,#19783,#19784);
#16700=AXIS2_PLACEMENT_3D('',#31233,#19788,#19789);
#16701=AXIS2_PLACEMENT_3D('',#31239,#19793,#19794);
#16702=AXIS2_PLACEMENT_3D('',#31242,#19797,#19798);
#16703=AXIS2_PLACEMENT_3D('',#31243,#19799,#19800);
#16704=AXIS2_PLACEMENT_3D('',#31244,#19801,#19802);
#16705=AXIS2_PLACEMENT_3D('',#31253,#19807,#19808);
#16706=AXIS2_PLACEMENT_3D('',#31259,#19812,#19813);
#16707=AXIS2_PLACEMENT_3D('',#31265,#19817,#19818);
#16708=AXIS2_PLACEMENT_3D('',#31268,#19821,#19822);
#16709=AXIS2_PLACEMENT_3D('',#31269,#19823,#19824);
#16710=AXIS2_PLACEMENT_3D('',#31270,#19825,#19826);
#16711=AXIS2_PLACEMENT_3D('',#31279,#19831,#19832);
#16712=AXIS2_PLACEMENT_3D('',#31285,#19836,#19837);
#16713=AXIS2_PLACEMENT_3D('',#31291,#19841,#19842);
#16714=AXIS2_PLACEMENT_3D('',#31294,#19845,#19846);
#16715=AXIS2_PLACEMENT_3D('',#31295,#19847,#19848);
#16716=AXIS2_PLACEMENT_3D('',#31296,#19849,#19850);
#16717=AXIS2_PLACEMENT_3D('',#31298,#19851,#19852);
#16718=AXIS2_PLACEMENT_3D('',#31301,#19854,#19855);
#16719=AXIS2_PLACEMENT_3D('',#31302,#19856,#19857);
#16720=AXIS2_PLACEMENT_3D('',#31304,#19858,#19859);
#16721=AXIS2_PLACEMENT_3D('',#31307,#19861,#19862);
#16722=AXIS2_PLACEMENT_3D('',#31308,#19863,#19864);
#16723=AXIS2_PLACEMENT_3D('',#31310,#19865,#19866);
#16724=AXIS2_PLACEMENT_3D('',#31313,#19868,#19869);
#16725=AXIS2_PLACEMENT_3D('',#31314,#19870,#19871);
#16726=AXIS2_PLACEMENT_3D('',#31316,#19872,#19873);
#16727=AXIS2_PLACEMENT_3D('',#31319,#19875,#19876);
#16728=AXIS2_PLACEMENT_3D('',#31320,#19877,#19878);
#16729=AXIS2_PLACEMENT_3D('',#31329,#19883,#19884);
#16730=AXIS2_PLACEMENT_3D('',#31338,#19889,#19890);
#16731=AXIS2_PLACEMENT_3D('',#31341,#19893,#19894);
#16732=AXIS2_PLACEMENT_3D('',#31343,#19896,#19897);
#16733=AXIS2_PLACEMENT_3D('',#31345,#19899,#19900);
#16734=AXIS2_PLACEMENT_3D('',#31346,#19901,#19902);
#16735=AXIS2_PLACEMENT_3D('',#31348,#19903,#19904);
#16736=AXIS2_PLACEMENT_3D('',#31351,#19906,#19907);
#16737=AXIS2_PLACEMENT_3D('',#31352,#19908,#19909);
#16738=AXIS2_PLACEMENT_3D('',#31354,#19910,#19911);
#16739=AXIS2_PLACEMENT_3D('',#31357,#19913,#19914);
#16740=AXIS2_PLACEMENT_3D('',#31358,#19915,#19916);
#16741=AXIS2_PLACEMENT_3D('',#31360,#19917,#19918);
#16742=AXIS2_PLACEMENT_3D('',#31363,#19920,#19921);
#16743=AXIS2_PLACEMENT_3D('',#31364,#19922,#19923);
#16744=AXIS2_PLACEMENT_3D('',#31366,#19924,#19925);
#16745=AXIS2_PLACEMENT_3D('',#31369,#19927,#19928);
#16746=AXIS2_PLACEMENT_3D('',#31370,#19929,#19930);
#16747=AXIS2_PLACEMENT_3D('',#31372,#19931,#19932);
#16748=AXIS2_PLACEMENT_3D('',#31375,#19934,#19935);
#16749=AXIS2_PLACEMENT_3D('',#31376,#19936,#19937);
#16750=AXIS2_PLACEMENT_3D('',#31378,#19938,#19939);
#16751=AXIS2_PLACEMENT_3D('',#31381,#19941,#19942);
#16752=AXIS2_PLACEMENT_3D('',#31382,#19943,#19944);
#16753=AXIS2_PLACEMENT_3D('',#31391,#19949,#19950);
#16754=AXIS2_PLACEMENT_3D('',#31397,#19954,#19955);
#16755=AXIS2_PLACEMENT_3D('',#31403,#19959,#19960);
#16756=AXIS2_PLACEMENT_3D('',#31406,#19963,#19964);
#16757=AXIS2_PLACEMENT_3D('',#31407,#19965,#19966);
#16758=AXIS2_PLACEMENT_3D('',#31408,#19967,#19968);
#16759=AXIS2_PLACEMENT_3D('',#31417,#19973,#19974);
#16760=AXIS2_PLACEMENT_3D('',#31423,#19978,#19979);
#16761=AXIS2_PLACEMENT_3D('',#31429,#19983,#19984);
#16762=AXIS2_PLACEMENT_3D('',#31435,#19988,#19989);
#16763=AXIS2_PLACEMENT_3D('',#31441,#19993,#19994);
#16764=AXIS2_PLACEMENT_3D('',#31447,#19998,#19999);
#16765=AXIS2_PLACEMENT_3D('',#31450,#20002,#20003);
#16766=AXIS2_PLACEMENT_3D('',#31451,#20004,#20005);
#16767=AXIS2_PLACEMENT_3D('',#31452,#20006,#20007);
#16768=AXIS2_PLACEMENT_3D('',#31461,#20012,#20013);
#16769=AXIS2_PLACEMENT_3D('',#31467,#20017,#20018);
#16770=AXIS2_PLACEMENT_3D('',#31473,#20022,#20023);
#16771=AXIS2_PLACEMENT_3D('',#31479,#20027,#20028);
#16772=AXIS2_PLACEMENT_3D('',#31485,#20032,#20033);
#16773=AXIS2_PLACEMENT_3D('',#31491,#20037,#20038);
#16774=AXIS2_PLACEMENT_3D('',#31494,#20041,#20042);
#16775=AXIS2_PLACEMENT_3D('',#31495,#20043,#20044);
#16776=AXIS2_PLACEMENT_3D('',#31496,#20045,#20046);
#16777=AXIS2_PLACEMENT_3D('',#31505,#20051,#20052);
#16778=AXIS2_PLACEMENT_3D('',#31511,#20056,#20057);
#16779=AXIS2_PLACEMENT_3D('',#31517,#20061,#20062);
#16780=AXIS2_PLACEMENT_3D('',#31523,#20066,#20067);
#16781=AXIS2_PLACEMENT_3D('',#31529,#20071,#20072);
#16782=AXIS2_PLACEMENT_3D('',#31535,#20076,#20077);
#16783=AXIS2_PLACEMENT_3D('',#31538,#20080,#20081);
#16784=AXIS2_PLACEMENT_3D('',#31539,#20082,#20083);
#16785=AXIS2_PLACEMENT_3D('',#31540,#20084,#20085);
#16786=AXIS2_PLACEMENT_3D('',#31549,#20090,#20091);
#16787=AXIS2_PLACEMENT_3D('',#31555,#20095,#20096);
#16788=AXIS2_PLACEMENT_3D('',#31561,#20100,#20101);
#16789=AXIS2_PLACEMENT_3D('',#31567,#20105,#20106);
#16790=AXIS2_PLACEMENT_3D('',#31573,#20110,#20111);
#16791=AXIS2_PLACEMENT_3D('',#31579,#20115,#20116);
#16792=AXIS2_PLACEMENT_3D('',#31582,#20119,#20120);
#16793=AXIS2_PLACEMENT_3D('',#31583,#20121,#20122);
#16794=AXIS2_PLACEMENT_3D('',#31584,#20123,#20124);
#16795=AXIS2_PLACEMENT_3D('',#31593,#20129,#20130);
#16796=AXIS2_PLACEMENT_3D('',#31599,#20134,#20135);
#16797=AXIS2_PLACEMENT_3D('',#31605,#20139,#20140);
#16798=AXIS2_PLACEMENT_3D('',#31611,#20144,#20145);
#16799=AXIS2_PLACEMENT_3D('',#31617,#20149,#20150);
#16800=AXIS2_PLACEMENT_3D('',#31623,#20154,#20155);
#16801=AXIS2_PLACEMENT_3D('',#31626,#20158,#20159);
#16802=AXIS2_PLACEMENT_3D('',#31627,#20160,#20161);
#16803=AXIS2_PLACEMENT_3D('',#31628,#20162,#20163);
#16804=AXIS2_PLACEMENT_3D('',#31637,#20168,#20169);
#16805=AXIS2_PLACEMENT_3D('',#31643,#20173,#20174);
#16806=AXIS2_PLACEMENT_3D('',#31649,#20178,#20179);
#16807=AXIS2_PLACEMENT_3D('',#31655,#20183,#20184);
#16808=AXIS2_PLACEMENT_3D('',#31661,#20188,#20189);
#16809=AXIS2_PLACEMENT_3D('',#31667,#20193,#20194);
#16810=AXIS2_PLACEMENT_3D('',#31670,#20197,#20198);
#16811=AXIS2_PLACEMENT_3D('',#31671,#20199,#20200);
#16812=AXIS2_PLACEMENT_3D('',#31672,#20201,#20202);
#16813=AXIS2_PLACEMENT_3D('',#31681,#20207,#20208);
#16814=AXIS2_PLACEMENT_3D('',#31687,#20212,#20213);
#16815=AXIS2_PLACEMENT_3D('',#31693,#20217,#20218);
#16816=AXIS2_PLACEMENT_3D('',#31699,#20222,#20223);
#16817=AXIS2_PLACEMENT_3D('',#31705,#20227,#20228);
#16818=AXIS2_PLACEMENT_3D('',#31711,#20232,#20233);
#16819=AXIS2_PLACEMENT_3D('',#31714,#20236,#20237);
#16820=AXIS2_PLACEMENT_3D('',#31715,#20238,#20239);
#16821=AXIS2_PLACEMENT_3D('',#31716,#20240,#20241);
#16822=AXIS2_PLACEMENT_3D('',#31725,#20246,#20247);
#16823=AXIS2_PLACEMENT_3D('',#31731,#20251,#20252);
#16824=AXIS2_PLACEMENT_3D('',#31737,#20256,#20257);
#16825=AXIS2_PLACEMENT_3D('',#31743,#20261,#20262);
#16826=AXIS2_PLACEMENT_3D('',#31749,#20266,#20267);
#16827=AXIS2_PLACEMENT_3D('',#31755,#20271,#20272);
#16828=AXIS2_PLACEMENT_3D('',#31758,#20275,#20276);
#16829=AXIS2_PLACEMENT_3D('',#31759,#20277,#20278);
#16830=AXIS2_PLACEMENT_3D('',#31760,#20279,#20280);
#16831=AXIS2_PLACEMENT_3D('',#31769,#20285,#20286);
#16832=AXIS2_PLACEMENT_3D('',#31775,#20290,#20291);
#16833=AXIS2_PLACEMENT_3D('',#31781,#20295,#20296);
#16834=AXIS2_PLACEMENT_3D('',#31787,#20300,#20301);
#16835=AXIS2_PLACEMENT_3D('',#31793,#20305,#20306);
#16836=AXIS2_PLACEMENT_3D('',#31799,#20310,#20311);
#16837=AXIS2_PLACEMENT_3D('',#31802,#20314,#20315);
#16838=AXIS2_PLACEMENT_3D('',#31803,#20316,#20317);
#16839=AXIS2_PLACEMENT_3D('',#31804,#20318,#20319);
#16840=AXIS2_PLACEMENT_3D('',#31813,#20324,#20325);
#16841=AXIS2_PLACEMENT_3D('',#31819,#20329,#20330);
#16842=AXIS2_PLACEMENT_3D('',#31825,#20334,#20335);
#16843=AXIS2_PLACEMENT_3D('',#31831,#20339,#20340);
#16844=AXIS2_PLACEMENT_3D('',#31837,#20344,#20345);
#16845=AXIS2_PLACEMENT_3D('',#31843,#20349,#20350);
#16846=AXIS2_PLACEMENT_3D('',#31846,#20353,#20354);
#16847=AXIS2_PLACEMENT_3D('',#31847,#20355,#20356);
#16848=AXIS2_PLACEMENT_3D('',#31848,#20357,#20358);
#16849=AXIS2_PLACEMENT_3D('',#31857,#20363,#20364);
#16850=AXIS2_PLACEMENT_3D('',#31863,#20368,#20369);
#16851=AXIS2_PLACEMENT_3D('',#31869,#20373,#20374);
#16852=AXIS2_PLACEMENT_3D('',#31875,#20378,#20379);
#16853=AXIS2_PLACEMENT_3D('',#31881,#20383,#20384);
#16854=AXIS2_PLACEMENT_3D('',#31887,#20388,#20389);
#16855=AXIS2_PLACEMENT_3D('',#31890,#20392,#20393);
#16856=AXIS2_PLACEMENT_3D('',#31891,#20394,#20395);
#16857=AXIS2_PLACEMENT_3D('',#31892,#20396,#20397);
#16858=AXIS2_PLACEMENT_3D('',#31894,#20398,#20399);
#16859=AXIS2_PLACEMENT_3D('',#31897,#20401,#20402);
#16860=AXIS2_PLACEMENT_3D('',#31898,#20403,#20404);
#16861=AXIS2_PLACEMENT_3D('',#31900,#20405,#20406);
#16862=AXIS2_PLACEMENT_3D('',#31903,#20408,#20409);
#16863=AXIS2_PLACEMENT_3D('',#31904,#20410,#20411);
#16864=AXIS2_PLACEMENT_3D('',#31906,#20412,#20413);
#16865=AXIS2_PLACEMENT_3D('',#31909,#20415,#20416);
#16866=AXIS2_PLACEMENT_3D('',#31910,#20417,#20418);
#16867=AXIS2_PLACEMENT_3D('',#31912,#20419,#20420);
#16868=AXIS2_PLACEMENT_3D('',#31915,#20422,#20423);
#16869=AXIS2_PLACEMENT_3D('',#31916,#20424,#20425);
#16870=AXIS2_PLACEMENT_3D('',#31925,#20430,#20431);
#16871=AXIS2_PLACEMENT_3D('',#31934,#20436,#20437);
#16872=AXIS2_PLACEMENT_3D('',#31937,#20440,#20441);
#16873=AXIS2_PLACEMENT_3D('',#31939,#20443,#20444);
#16874=AXIS2_PLACEMENT_3D('',#31941,#20446,#20447);
#16875=AXIS2_PLACEMENT_3D('',#31942,#20448,#20449);
#16876=AXIS2_PLACEMENT_3D('',#31951,#20454,#20455);
#16877=AXIS2_PLACEMENT_3D('',#31957,#20459,#20460);
#16878=AXIS2_PLACEMENT_3D('',#31963,#20464,#20465);
#16879=AXIS2_PLACEMENT_3D('',#31966,#20468,#20469);
#16880=AXIS2_PLACEMENT_3D('',#31967,#20470,#20471);
#16881=AXIS2_PLACEMENT_3D('',#31968,#20472,#20473);
#16882=AXIS2_PLACEMENT_3D('',#31977,#20478,#20479);
#16883=AXIS2_PLACEMENT_3D('',#31983,#20483,#20484);
#16884=AXIS2_PLACEMENT_3D('',#31989,#20488,#20489);
#16885=AXIS2_PLACEMENT_3D('',#31992,#20492,#20493);
#16886=AXIS2_PLACEMENT_3D('',#31993,#20494,#20495);
#16887=AXIS2_PLACEMENT_3D('',#31994,#20496,#20497);
#16888=AXIS2_PLACEMENT_3D('',#32003,#20502,#20503);
#16889=AXIS2_PLACEMENT_3D('',#32009,#20507,#20508);
#16890=AXIS2_PLACEMENT_3D('',#32015,#20512,#20513);
#16891=AXIS2_PLACEMENT_3D('',#32018,#20516,#20517);
#16892=AXIS2_PLACEMENT_3D('',#32019,#20518,#20519);
#16893=AXIS2_PLACEMENT_3D('',#32020,#20520,#20521);
#16894=AXIS2_PLACEMENT_3D('',#32029,#20526,#20527);
#16895=AXIS2_PLACEMENT_3D('',#32035,#20531,#20532);
#16896=AXIS2_PLACEMENT_3D('',#32041,#20536,#20537);
#16897=AXIS2_PLACEMENT_3D('',#32044,#20540,#20541);
#16898=AXIS2_PLACEMENT_3D('',#32045,#20542,#20543);
#16899=AXIS2_PLACEMENT_3D('',#32046,#20544,#20545);
#16900=AXIS2_PLACEMENT_3D('',#32055,#20550,#20551);
#16901=AXIS2_PLACEMENT_3D('',#32061,#20555,#20556);
#16902=AXIS2_PLACEMENT_3D('',#32067,#20560,#20561);
#16903=AXIS2_PLACEMENT_3D('',#32070,#20564,#20565);
#16904=AXIS2_PLACEMENT_3D('',#32071,#20566,#20567);
#16905=AXIS2_PLACEMENT_3D('',#32072,#20568,#20569);
#16906=AXIS2_PLACEMENT_3D('',#32081,#20574,#20575);
#16907=AXIS2_PLACEMENT_3D('',#32087,#20579,#20580);
#16908=AXIS2_PLACEMENT_3D('',#32093,#20584,#20585);
#16909=AXIS2_PLACEMENT_3D('',#32096,#20588,#20589);
#16910=AXIS2_PLACEMENT_3D('',#32097,#20590,#20591);
#16911=AXIS2_PLACEMENT_3D('',#32098,#20592,#20593);
#16912=AXIS2_PLACEMENT_3D('',#32107,#20598,#20599);
#16913=AXIS2_PLACEMENT_3D('',#32113,#20603,#20604);
#16914=AXIS2_PLACEMENT_3D('',#32119,#20608,#20609);
#16915=AXIS2_PLACEMENT_3D('',#32122,#20612,#20613);
#16916=AXIS2_PLACEMENT_3D('',#32123,#20614,#20615);
#16917=AXIS2_PLACEMENT_3D('',#32124,#20616,#20617);
#16918=AXIS2_PLACEMENT_3D('',#32133,#20622,#20623);
#16919=AXIS2_PLACEMENT_3D('',#32139,#20627,#20628);
#16920=AXIS2_PLACEMENT_3D('',#32145,#20632,#20633);
#16921=AXIS2_PLACEMENT_3D('',#32148,#20636,#20637);
#16922=AXIS2_PLACEMENT_3D('',#32149,#20638,#20639);
#16923=AXIS2_PLACEMENT_3D('',#32150,#20640,#20641);
#16924=AXIS2_PLACEMENT_3D('',#32159,#20646,#20647);
#16925=AXIS2_PLACEMENT_3D('',#32165,#20651,#20652);
#16926=AXIS2_PLACEMENT_3D('',#32171,#20656,#20657);
#16927=AXIS2_PLACEMENT_3D('',#32174,#20660,#20661);
#16928=AXIS2_PLACEMENT_3D('',#32175,#20662,#20663);
#16929=AXIS2_PLACEMENT_3D('',#32176,#20664,#20665);
#16930=AXIS2_PLACEMENT_3D('',#32185,#20670,#20671);
#16931=AXIS2_PLACEMENT_3D('',#32191,#20675,#20676);
#16932=AXIS2_PLACEMENT_3D('',#32197,#20680,#20681);
#16933=AXIS2_PLACEMENT_3D('',#32200,#20684,#20685);
#16934=AXIS2_PLACEMENT_3D('',#32201,#20686,#20687);
#16935=AXIS2_PLACEMENT_3D('',#32202,#20688,#20689);
#16936=AXIS2_PLACEMENT_3D('',#32211,#20694,#20695);
#16937=AXIS2_PLACEMENT_3D('',#32217,#20699,#20700);
#16938=AXIS2_PLACEMENT_3D('',#32223,#20704,#20705);
#16939=AXIS2_PLACEMENT_3D('',#32226,#20708,#20709);
#16940=AXIS2_PLACEMENT_3D('',#32227,#20710,#20711);
#16941=AXIS2_PLACEMENT_3D('',#32228,#20712,#20713);
#16942=AXIS2_PLACEMENT_3D('',#32237,#20718,#20719);
#16943=AXIS2_PLACEMENT_3D('',#32243,#20723,#20724);
#16944=AXIS2_PLACEMENT_3D('',#32249,#20728,#20729);
#16945=AXIS2_PLACEMENT_3D('',#32252,#20732,#20733);
#16946=AXIS2_PLACEMENT_3D('',#32253,#20734,#20735);
#16947=AXIS2_PLACEMENT_3D('',#32254,#20736,#20737);
#16948=AXIS2_PLACEMENT_3D('',#32263,#20742,#20743);
#16949=AXIS2_PLACEMENT_3D('',#32269,#20747,#20748);
#16950=AXIS2_PLACEMENT_3D('',#32275,#20752,#20753);
#16951=AXIS2_PLACEMENT_3D('',#32278,#20756,#20757);
#16952=AXIS2_PLACEMENT_3D('',#32279,#20758,#20759);
#16953=AXIS2_PLACEMENT_3D('',#32280,#20760,#20761);
#16954=AXIS2_PLACEMENT_3D('',#32289,#20766,#20767);
#16955=AXIS2_PLACEMENT_3D('',#32295,#20771,#20772);
#16956=AXIS2_PLACEMENT_3D('',#32301,#20776,#20777);
#16957=AXIS2_PLACEMENT_3D('',#32304,#20780,#20781);
#16958=AXIS2_PLACEMENT_3D('',#32305,#20782,#20783);
#16959=AXIS2_PLACEMENT_3D('',#32306,#20784,#20785);
#16960=AXIS2_PLACEMENT_3D('',#32315,#20790,#20791);
#16961=AXIS2_PLACEMENT_3D('',#32321,#20795,#20796);
#16962=AXIS2_PLACEMENT_3D('',#32327,#20800,#20801);
#16963=AXIS2_PLACEMENT_3D('',#32330,#20804,#20805);
#16964=AXIS2_PLACEMENT_3D('',#32331,#20806,#20807);
#16965=AXIS2_PLACEMENT_3D('',#32332,#20808,#20809);
#16966=AXIS2_PLACEMENT_3D('',#32341,#20814,#20815);
#16967=AXIS2_PLACEMENT_3D('',#32347,#20819,#20820);
#16968=AXIS2_PLACEMENT_3D('',#32353,#20824,#20825);
#16969=AXIS2_PLACEMENT_3D('',#32356,#20828,#20829);
#16970=AXIS2_PLACEMENT_3D('',#32357,#20830,#20831);
#16971=AXIS2_PLACEMENT_3D('',#32358,#20832,#20833);
#16972=AXIS2_PLACEMENT_3D('',#32367,#20838,#20839);
#16973=AXIS2_PLACEMENT_3D('',#32373,#20843,#20844);
#16974=AXIS2_PLACEMENT_3D('',#32379,#20848,#20849);
#16975=AXIS2_PLACEMENT_3D('',#32382,#20852,#20853);
#16976=AXIS2_PLACEMENT_3D('',#32383,#20854,#20855);
#16977=AXIS2_PLACEMENT_3D('',#32384,#20856,#20857);
#16978=AXIS2_PLACEMENT_3D('',#32393,#20862,#20863);
#16979=AXIS2_PLACEMENT_3D('',#32399,#20867,#20868);
#16980=AXIS2_PLACEMENT_3D('',#32405,#20872,#20873);
#16981=AXIS2_PLACEMENT_3D('',#32408,#20876,#20877);
#16982=AXIS2_PLACEMENT_3D('',#32409,#20878,#20879);
#16983=AXIS2_PLACEMENT_3D('',#32410,#20880,#20881);
#16984=AXIS2_PLACEMENT_3D('',#32419,#20886,#20887);
#16985=AXIS2_PLACEMENT_3D('',#32425,#20891,#20892);
#16986=AXIS2_PLACEMENT_3D('',#32431,#20896,#20897);
#16987=AXIS2_PLACEMENT_3D('',#32434,#20900,#20901);
#16988=AXIS2_PLACEMENT_3D('',#32435,#20902,#20903);
#16989=AXIS2_PLACEMENT_3D('',#32436,#20904,#20905);
#16990=AXIS2_PLACEMENT_3D('',#32445,#20910,#20911);
#16991=AXIS2_PLACEMENT_3D('',#32451,#20915,#20916);
#16992=AXIS2_PLACEMENT_3D('',#32457,#20920,#20921);
#16993=AXIS2_PLACEMENT_3D('',#32460,#20924,#20925);
#16994=AXIS2_PLACEMENT_3D('',#32461,#20926,#20927);
#16995=AXIS2_PLACEMENT_3D('',#32462,#20928,#20929);
#16996=AXIS2_PLACEMENT_3D('',#32471,#20934,#20935);
#16997=AXIS2_PLACEMENT_3D('',#32477,#20939,#20940);
#16998=AXIS2_PLACEMENT_3D('',#32483,#20944,#20945);
#16999=AXIS2_PLACEMENT_3D('',#32486,#20948,#20949);
#17000=AXIS2_PLACEMENT_3D('',#32487,#20950,#20951);
#17001=AXIS2_PLACEMENT_3D('',#32488,#20952,#20953);
#17002=AXIS2_PLACEMENT_3D('',#32497,#20958,#20959);
#17003=AXIS2_PLACEMENT_3D('',#32503,#20963,#20964);
#17004=AXIS2_PLACEMENT_3D('',#32509,#20968,#20969);
#17005=AXIS2_PLACEMENT_3D('',#32512,#20972,#20973);
#17006=AXIS2_PLACEMENT_3D('',#32513,#20974,#20975);
#19276=DIRECTION('axis',(0.,0.,1.));
#19277=DIRECTION('refdir',(1.,0.,0.));
#19278=DIRECTION('center_axis',(-1.,0.,0.));
#19279=DIRECTION('ref_axis',(0.,0.,1.));
#19280=DIRECTION('',(0.,1.,0.));
#19281=DIRECTION('',(0.,0.,-1.));
#19282=DIRECTION('',(0.,1.,0.));
#19283=DIRECTION('',(0.,0.,-1.));
#19284=DIRECTION('center_axis',(0.,-1.,0.));
#19285=DIRECTION('ref_axis',(0.,0.,-1.));
#19286=DIRECTION('',(-1.,0.,0.));
#19287=DIRECTION('',(0.,0.,-1.));
#19288=DIRECTION('',(-1.,0.,0.));
#19289=DIRECTION('center_axis',(1.,0.,0.));
#19290=DIRECTION('ref_axis',(0.,0.,-1.));
#19291=DIRECTION('',(0.,-1.,0.));
#19292=DIRECTION('',(0.,0.,-1.));
#19293=DIRECTION('',(0.,-1.,0.));
#19294=DIRECTION('center_axis',(0.,1.,0.));
#19295=DIRECTION('ref_axis',(0.,0.,1.));
#19296=DIRECTION('',(1.,0.,0.));
#19297=DIRECTION('',(1.,0.,0.));
#19298=DIRECTION('center_axis',(0.,0.,-1.));
#19299=DIRECTION('ref_axis',(-1.,0.,0.));
#19300=DIRECTION('center_axis',(0.,0.,-1.));
#19301=DIRECTION('ref_axis',(-1.,0.,0.));
#19302=DIRECTION('center_axis',(-1.,0.,0.));
#19303=DIRECTION('ref_axis',(0.,0.,1.));
#19304=DIRECTION('center_axis',(1.,0.,0.));
#19305=DIRECTION('ref_axis',(0.,0.,-1.));
#19306=DIRECTION('',(-1.,0.,0.));
#19307=DIRECTION('center_axis',(1.,0.,0.));
#19308=DIRECTION('ref_axis',(0.,0.,-1.));
#19309=DIRECTION('center_axis',(1.,0.,0.));
#19310=DIRECTION('ref_axis',(0.,0.,-1.));
#19311=DIRECTION('',(0.,-1.,0.));
#19312=DIRECTION('',(0.,-0.500011000363013,-0.866019052628739));
#19313=DIRECTION('',(0.,0.866029956157432,-0.499992114975783));
#19314=DIRECTION('',(0.,0.782106676792726,0.623144562775154));
#19315=DIRECTION('center_axis',(-1.,0.,0.));
#19316=DIRECTION('ref_axis',(0.,0.,-1.));
#19317=DIRECTION('',(0.,0.,1.));
#19318=DIRECTION('center_axis',(1.,0.,0.));
#19319=DIRECTION('ref_axis',(0.,0.,-1.));
#19320=DIRECTION('',(0.,-1.,0.));
#19321=DIRECTION('',(0.,0.,1.));
#19322=DIRECTION('center_axis',(-1.,0.,0.));
#19323=DIRECTION('ref_axis',(0.,0.,-1.));
#19324=DIRECTION('',(0.,0.782106676792726,0.623144562775154));
#19325=DIRECTION('',(0.,0.866029956157432,-0.499992114975783));
#19326=DIRECTION('',(0.,-0.500011000363013,-0.866019052628739));
#19327=DIRECTION('center_axis',(0.,0.,-1.));
#19328=DIRECTION('ref_axis',(-1.,0.,0.));
#19329=DIRECTION('',(-1.,0.,0.));
#19330=DIRECTION('',(-1.,0.,0.));
#19331=DIRECTION('center_axis',(0.,0.866019052628739,-0.500011000363013));
#19332=DIRECTION('ref_axis',(0.,0.500011000363013,0.866019052628739));
#19333=DIRECTION('',(-1.,0.,0.));
#19334=DIRECTION('center_axis',(0.,0.499992114975783,0.866029956157432));
#19335=DIRECTION('ref_axis',(0.,-0.866029956157432,0.499992114975783));
#19336=DIRECTION('',(-1.,0.,0.));
#19337=DIRECTION('center_axis',(0.,-0.623144562775154,0.782106676792726));
#19338=DIRECTION('ref_axis',(0.,-0.782106676792726,-0.623144562775154));
#19339=DIRECTION('',(-1.,0.,0.));
#19340=DIRECTION('center_axis',(-1.,0.,0.));
#19341=DIRECTION('ref_axis',(0.,0.,1.));
#19342=DIRECTION('',(-1.,0.,0.));
#19343=DIRECTION('center_axis',(0.,-1.,0.));
#19344=DIRECTION('ref_axis',(0.,0.,-1.));
#19345=DIRECTION('center_axis',(1.,0.,0.));
#19346=DIRECTION('ref_axis',(0.,0.,1.));
#19347=DIRECTION('center_axis',(1.,0.,0.));
#19348=DIRECTION('ref_axis',(0.,0.,-1.));
#19349=DIRECTION('',(1.,0.,0.));
#19350=DIRECTION('center_axis',(1.,0.,0.));
#19351=DIRECTION('ref_axis',(0.,0.,-1.));
#19352=DIRECTION('center_axis',(-1.,0.,0.));
#19353=DIRECTION('ref_axis',(0.,0.,-1.));
#19354=DIRECTION('',(0.,-1.,0.));
#19355=DIRECTION('',(0.,0.,1.));
#19356=DIRECTION('center_axis',(-1.,0.,0.));
#19357=DIRECTION('ref_axis',(0.,0.,-1.));
#19358=DIRECTION('',(0.,0.782106676792726,0.623144562775154));
#19359=DIRECTION('',(0.,0.866029956157432,-0.499992114975783));
#19360=DIRECTION('',(0.,-0.500011000363013,-0.866019052628739));
#19361=DIRECTION('center_axis',(-1.,0.,0.));
#19362=DIRECTION('ref_axis',(0.,0.,-1.));
#19363=DIRECTION('',(0.,-1.,0.));
#19364=DIRECTION('',(0.,-0.500011000363013,-0.866019052628739));
#19365=DIRECTION('',(0.,0.866029956157432,-0.499992114975783));
#19366=DIRECTION('',(0.,0.782106676792726,0.623144562775154));
#19367=DIRECTION('center_axis',(-1.,0.,0.));
#19368=DIRECTION('ref_axis',(0.,0.,-1.));
#19369=DIRECTION('',(0.,0.,1.));
#19370=DIRECTION('center_axis',(0.,0.,-1.));
#19371=DIRECTION('ref_axis',(1.,0.,0.));
#19372=DIRECTION('',(1.,0.,0.));
#19373=DIRECTION('',(1.,0.,0.));
#19374=DIRECTION('center_axis',(0.,0.866019052628739,-0.500011000363013));
#19375=DIRECTION('ref_axis',(0.,0.500011000363013,0.866019052628739));
#19376=DIRECTION('',(1.,0.,0.));
#19377=DIRECTION('center_axis',(0.,0.499992114975783,0.866029956157432));
#19378=DIRECTION('ref_axis',(0.,-0.866029956157432,0.499992114975783));
#19379=DIRECTION('',(1.,0.,0.));
#19380=DIRECTION('center_axis',(0.,-0.623144562775154,0.782106676792726));
#19381=DIRECTION('ref_axis',(0.,-0.782106676792726,-0.623144562775154));
#19382=DIRECTION('',(1.,0.,0.));
#19383=DIRECTION('center_axis',(1.,0.,0.));
#19384=DIRECTION('ref_axis',(0.,0.,1.));
#19385=DIRECTION('',(1.,0.,0.));
#19386=DIRECTION('center_axis',(0.,-1.,0.));
#19387=DIRECTION('ref_axis',(0.,0.,-1.));
#19388=DIRECTION('center_axis',(0.,0.499992114975783,0.866029956157432));
#19389=DIRECTION('ref_axis',(0.,-0.866029956157432,0.499992114975783));
#19390=DIRECTION('center_axis',(0.,-0.499992114975783,-0.866029956157432));
#19391=DIRECTION('ref_axis',(0.,0.866029956157432,-0.499992114975783));
#19392=DIRECTION('',(0.,0.499992114975783,0.866029956157432));
#19393=DIRECTION('center_axis',(0.,-0.499992114975783,-0.866029956157432));
#19394=DIRECTION('ref_axis',(0.,0.866029956157432,-0.499992114975783));
#19395=DIRECTION('center_axis',(0.,0.499992114975783,0.866029956157432));
#19396=DIRECTION('ref_axis',(0.,-0.866029956157432,0.499992114975783));
#19397=DIRECTION('center_axis',(0.,-0.499992114975783,-0.866029956157432));
#19398=DIRECTION('ref_axis',(0.,0.866029956157432,-0.499992114975783));
#19399=DIRECTION('',(0.,0.499992114975783,0.866029956157432));
#19400=DIRECTION('center_axis',(0.,-0.499992114975783,-0.866029956157432));
#19401=DIRECTION('ref_axis',(0.,0.866029956157432,-0.499992114975783));
#19402=DIRECTION('center_axis',(0.,0.499992114975783,0.866029956157432));
#19403=DIRECTION('ref_axis',(0.,-0.866029956157432,0.499992114975783));
#19404=DIRECTION('center_axis',(0.,-0.499992114975783,-0.866029956157432));
#19405=DIRECTION('ref_axis',(0.,0.866029956157432,-0.499992114975783));
#19406=DIRECTION('',(0.,0.499992114975783,0.866029956157432));
#19407=DIRECTION('center_axis',(0.,-0.499992114975783,-0.866029956157432));
#19408=DIRECTION('ref_axis',(0.,0.866029956157432,-0.499992114975783));
#19409=DIRECTION('center_axis',(0.,0.499992114975783,0.866029956157432));
#19410=DIRECTION('ref_axis',(0.,-0.866029956157432,0.499992114975783));
#19411=DIRECTION('center_axis',(0.,-0.499992114975783,-0.866029956157432));
#19412=DIRECTION('ref_axis',(0.,0.866029956157432,-0.499992114975783));
#19413=DIRECTION('',(0.,0.499992114975783,0.866029956157432));
#19414=DIRECTION('center_axis',(0.,-0.499992114975783,-0.866029956157432));
#19415=DIRECTION('ref_axis',(0.,0.866029956157432,-0.499992114975783));
#19416=DIRECTION('center_axis',(0.,0.499992114975783,0.866029956157432));
#19417=DIRECTION('ref_axis',(0.,-0.866029956157432,0.499992114975783));
#19418=DIRECTION('center_axis',(0.,-0.499992114975783,-0.866029956157432));
#19419=DIRECTION('ref_axis',(0.,0.866029956157432,-0.499992114975783));
#19420=DIRECTION('',(0.,0.499992114975783,0.866029956157432));
#19421=DIRECTION('center_axis',(0.,-0.499992114975783,-0.866029956157432));
#19422=DIRECTION('ref_axis',(0.,0.866029956157432,-0.499992114975783));
#19423=DIRECTION('center_axis',(0.,0.499992114975783,0.866029956157432));
#19424=DIRECTION('ref_axis',(0.,-0.866029956157432,0.499992114975783));
#19425=DIRECTION('',(0.,-0.866029956157432,0.499992114975783));
#19426=DIRECTION('',(-0.499722453489577,-0.750142665109869,0.433085963129978));
#19427=DIRECTION('',(0.,-0.866029956157433,0.499992114975782));
#19428=DIRECTION('',(-1.,0.,0.));
#19429=DIRECTION('',(0.,0.866029956157433,-0.499992114975782));
#19430=DIRECTION('',(-0.499722453489577,0.750142665109869,-0.433085963129978));
#19431=DIRECTION('',(0.,0.866029956157432,-0.499992114975783));
#19432=DIRECTION('',(1.,0.,0.));
#19433=DIRECTION('center_axis',(0.,0.499992114975783,0.866029956157432));
#19434=DIRECTION('ref_axis',(0.,-0.866029956157432,0.499992114975783));
#19435=DIRECTION('',(0.,-0.866029956157432,0.499992114975783));
#19436=DIRECTION('',(1.,0.,0.));
#19437=DIRECTION('',(0.,0.866029956157432,-0.499992114975783));
#19438=DIRECTION('',(-0.499722453489577,0.750142665109869,-0.433085963129978));
#19439=DIRECTION('',(0.,0.866029956157433,-0.499992114975782));
#19440=DIRECTION('',(-1.,0.,0.));
#19441=DIRECTION('',(0.,-0.866029956157433,0.499992114975782));
#19442=DIRECTION('',(-0.499722453489577,-0.750142665109869,0.433085963129978));
#19443=DIRECTION('center_axis',(-1.,0.,0.));
#19444=DIRECTION('ref_axis',(0.,0.,1.));
#19445=DIRECTION('',(0.,0.499992114975783,0.866029956157432));
#19446=DIRECTION('',(0.,0.499992114975783,0.866029956157432));
#19447=DIRECTION('center_axis',(-0.866185586048601,0.432774614486463,-0.249857286421141));
#19448=DIRECTION('ref_axis',(-0.446950695480888,-0.89455859271998,-3.10117349013882E-18));
#19449=DIRECTION('',(0.,0.499992114975783,0.866029956157432));
#19450=DIRECTION('center_axis',(-1.,0.,0.));
#19451=DIRECTION('ref_axis',(0.,0.,1.));
#19452=DIRECTION('',(0.,0.499992114975783,0.866029956157432));
#19453=DIRECTION('center_axis',(0.,0.866029956157432,-0.499992114975783));
#19454=DIRECTION('ref_axis',(0.,0.499992114975783,0.866029956157432));
#19455=DIRECTION('',(0.,0.499992114975783,0.866029956157432));
#19456=DIRECTION('center_axis',(1.,0.,0.));
#19457=DIRECTION('ref_axis',(0.,0.,-1.));
#19458=DIRECTION('',(0.,0.499992114975783,0.866029956157432));
#19459=DIRECTION('center_axis',(0.866185586048601,0.432774614486463,-0.249857286421141));
#19460=DIRECTION('ref_axis',(-0.446950695480888,0.89455859271998,3.10117349013882E-18));
#19461=DIRECTION('',(0.,0.499992114975783,0.866029956157432));
#19462=DIRECTION('center_axis',(1.,0.,0.));
#19463=DIRECTION('ref_axis',(0.,0.,-1.));
#19464=DIRECTION('',(0.,0.499992114975783,0.866029956157432));
#19465=DIRECTION('center_axis',(0.,-0.866029956157432,0.499992114975783));
#19466=DIRECTION('ref_axis',(0.,-0.499992114975783,-0.866029956157432));
#19467=DIRECTION('center_axis',(9.439207419131E-6,0.500006284256325,0.866021775485516));
#19468=DIRECTION('ref_axis',(5.27658532184428E-22,-0.866021775524096,0.5000062842786));
#19469=DIRECTION('',(0.499722453400429,0.750133220675019,-0.4331023214059));
#19470=DIRECTION('',(-0.866185586048601,0.432774614486463,-0.249857286421141));
#19471=DIRECTION('',(0.499722453400429,0.750133220675019,-0.4331023214059));
#19472=DIRECTION('',(-0.866185586048601,0.432774614486463,-0.249857286421141));
#19473=DIRECTION('center_axis',(-0.499722453400429,-0.750133220675019,0.4331023214059));
#19474=DIRECTION('ref_axis',(0.832237843570743,-0.55441876927889,-3.50686665358977E-17));
#19475=DIRECTION('',(9.43920741954911E-6,0.500006284256325,0.866021775485515));
#19476=DIRECTION('',(-0.866185586048601,0.432774614486463,-0.249857286421141));
#19477=DIRECTION('',(9.43920741954911E-6,0.500006284256325,0.866021775485515));
#19478=DIRECTION('center_axis',(-9.43920741930175E-6,-0.500006284256325,
-0.866021775485516));
#19479=DIRECTION('ref_axis',(-2.61520069381354E-22,0.866021775524096,-0.5000062842786));
#19480=DIRECTION('',(-0.499722453400429,-0.750133220675019,0.4331023214059));
#19481=DIRECTION('',(-0.866185586048601,0.432774614486463,-0.249857286421141));
#19482=DIRECTION('',(-0.499722453400429,-0.750133220675019,0.4331023214059));
#19483=DIRECTION('center_axis',(0.499722453400429,0.750133220675019,-0.4331023214059));
#19484=DIRECTION('ref_axis',(-0.832237843570743,0.55441876927889,2.11982739611214E-17));
#19485=DIRECTION('',(-9.43920741954911E-6,-0.500006284256325,-0.866021775485515));
#19486=DIRECTION('',(-9.43920741954911E-6,-0.500006284256325,-0.866021775485515));
#19487=DIRECTION('center_axis',(-0.866185586048601,0.432774614486463,-0.249857286421141));
#19488=DIRECTION('ref_axis',(-0.446950695480887,-0.89455859271998,-4.18661307789075E-19));
#19489=DIRECTION('center_axis',(-0.866185586048601,0.432774614486463,-0.249857286421141));
#19490=DIRECTION('ref_axis',(-0.446950695480887,-0.89455859271998,-4.18661307789075E-19));
#19491=DIRECTION('center_axis',(0.,0.500011000363013,0.866019052628739));
#19492=DIRECTION('ref_axis',(0.,-0.866019052628739,0.500011000363013));
#19493=DIRECTION('',(0.,0.866019052628739,-0.500011000363013));
#19494=DIRECTION('',(-1.,0.,0.));
#19495=DIRECTION('',(0.,0.866019052628739,-0.500011000363013));
#19496=DIRECTION('',(-1.,0.,0.));
#19497=DIRECTION('center_axis',(0.,-0.866019052628739,0.500011000363013));
#19498=DIRECTION('ref_axis',(0.,-0.500011000363013,-0.866019052628739));
#19499=DIRECTION('',(0.,0.500011000363013,0.866019052628739));
#19500=DIRECTION('',(-1.,0.,0.));
#19501=DIRECTION('',(0.,0.500011000363013,0.866019052628739));
#19502=DIRECTION('center_axis',(0.,-0.500011000363012,-0.86601905262874));
#19503=DIRECTION('ref_axis',(0.,0.86601905262874,-0.500011000363012));
#19504=DIRECTION('',(0.,-0.86601905262874,0.500011000363011));
#19505=DIRECTION('',(-1.,0.,0.));
#19506=DIRECTION('',(0.,-0.86601905262874,0.500011000363011));
#19507=DIRECTION('center_axis',(0.,0.866019052628739,-0.500011000363013));
#19508=DIRECTION('ref_axis',(0.,0.500011000363013,0.866019052628739));
#19509=DIRECTION('',(0.,-0.500011000363013,-0.866019052628739));
#19510=DIRECTION('',(0.,-0.500011000363013,-0.866019052628739));
#19511=DIRECTION('center_axis',(1.,0.,0.));
#19512=DIRECTION('ref_axis',(0.,0.,-1.));
#19513=DIRECTION('center_axis',(1.,0.,0.));
#19514=DIRECTION('ref_axis',(0.,0.,-1.));
#19515=DIRECTION('center_axis',(-0.866183663354203,0.432777500629603,-0.249858952785541));
#19516=DIRECTION('ref_axis',(-0.44695387464567,-0.894557004298341,2.04692415542437E-18));
#19517=DIRECTION('',(0.499725786055908,0.750131555564074,-0.433101360073861));
#19518=DIRECTION('',(-9.43920741916444E-6,-0.500006284256325,-0.866021775485515));
#19519=DIRECTION('',(0.499725786055908,0.750131555564074,-0.433101360073861));
#19520=DIRECTION('',(-9.43920741916444E-6,-0.500006284256325,-0.866021775485515));
#19521=DIRECTION('center_axis',(1.38189965515079E-17,-0.866021775524096,
0.5000062842786));
#19522=DIRECTION('ref_axis',(1.57777990579274E-34,-0.5000062842786,-0.866021775524096));
#19523=DIRECTION('',(-0.999999999955451,4.71966302817637E-6,8.17455916868661E-6));
#19524=DIRECTION('',(-9.43920741916444E-6,-0.500006284256325,-0.866021775485515));
#19525=DIRECTION('',(-0.999999999955451,4.71966302817637E-6,8.17455916868661E-6));
#19526=DIRECTION('center_axis',(0.866187508712929,0.432763552136484,-0.249869781470073));
#19527=DIRECTION('ref_axis',(-0.446940759058379,0.894563557212298,1.17495033585261E-17));
#19528=DIRECTION('',(0.499719120767447,-0.750139602771641,0.433095112755863));
#19529=DIRECTION('',(-9.43920741916444E-6,-0.500006284256325,-0.866021775485515));
#19530=DIRECTION('',(0.499719120767447,-0.750139602771641,0.433095112755863));
#19531=DIRECTION('center_axis',(0.999999999955451,-4.7196630281914E-6,-8.17455916868501E-6));
#19532=DIRECTION('ref_axis',(-8.17455916877606E-6,-2.91745525458034E-27,
-0.999999999966588));
#19533=DIRECTION('',(0.,-0.866021775524096,0.500006284278599));
#19534=DIRECTION('',(-9.43920741916444E-6,-0.500006284256325,-0.866021775485515));
#19535=DIRECTION('',(0.,-0.866021775524096,0.500006284278599));
#19536=DIRECTION('center_axis',(-1.3955513918745E-17,0.866021775524096,
-0.5000062842786));
#19537=DIRECTION('ref_axis',(4.04649682246767E-34,0.5000062842786,0.866021775524096));
#19538=DIRECTION('',(0.999999999955451,-4.71966302817428E-6,-8.17455916868326E-6));
#19539=DIRECTION('',(-9.43920741916444E-6,-0.500006284256325,-0.866021775485515));
#19540=DIRECTION('',(0.999999999955451,-4.71966302817428E-6,-8.17455916868326E-6));
#19541=DIRECTION('center_axis',(-0.999999999955451,4.7196630281914E-6,8.17455916868501E-6));
#19542=DIRECTION('ref_axis',(8.17455916877606E-6,2.91745525458034E-27,0.999999999966588));
#19543=DIRECTION('',(0.,0.866021775524096,-0.500006284278599));
#19544=DIRECTION('',(0.,0.866021775524097,-0.500006284278599));
#19545=DIRECTION('center_axis',(9.43920741915831E-6,0.500006284256325,0.866021775485515));
#19546=DIRECTION('ref_axis',(2.19424632593594E-22,-0.866021775524096,0.5000062842786));
#19547=DIRECTION('center_axis',(9.43920741915831E-6,0.500006284256325,0.866021775485515));
#19548=DIRECTION('ref_axis',(2.19424632593594E-22,-0.866021775524096,0.5000062842786));
#19549=DIRECTION('center_axis',(0.,0.866019052628739,-0.500011000363013));
#19550=DIRECTION('ref_axis',(0.,0.500011000363013,0.866019052628739));
#19551=DIRECTION('center_axis',(0.,-0.866019052628739,0.500011000363013));
#19552=DIRECTION('ref_axis',(0.,-0.500011000363013,-0.866019052628739));
#19553=DIRECTION('',(0.,0.866019052628739,-0.500011000363013));
#19554=DIRECTION('center_axis',(0.,-0.866019052628739,0.500011000363013));
#19555=DIRECTION('ref_axis',(0.,-0.500011000363013,-0.866019052628739));
#19556=DIRECTION('center_axis',(0.,0.866019052628739,-0.500011000363013));
#19557=DIRECTION('ref_axis',(0.,0.500011000363013,0.866019052628739));
#19558=DIRECTION('center_axis',(0.,-0.866019052628739,0.500011000363013));
#19559=DIRECTION('ref_axis',(0.,-0.500011000363013,-0.86601905262874));
#19560=DIRECTION('',(0.,0.866019052628739,-0.500011000363013));
#19561=DIRECTION('center_axis',(0.,-0.866019052628739,0.500011000363013));
#19562=DIRECTION('ref_axis',(0.,-0.500011000363013,-0.86601905262874));
#19563=DIRECTION('center_axis',(0.,0.866019052628739,-0.500011000363013));
#19564=DIRECTION('ref_axis',(0.,0.500011000363013,0.866019052628739));
#19565=DIRECTION('center_axis',(0.,-0.866019052628739,0.500011000363013));
#19566=DIRECTION('ref_axis',(0.,-0.500011000363013,-0.866019052628739));
#19567=DIRECTION('',(0.,0.866019052628739,-0.500011000363013));
#19568=DIRECTION('center_axis',(0.,-0.866019052628739,0.500011000363013));
#19569=DIRECTION('ref_axis',(0.,-0.500011000363013,-0.866019052628739));
#19570=DIRECTION('center_axis',(0.,-0.866019052628739,0.500011000363013));
#19571=DIRECTION('ref_axis',(0.,-0.500011000363013,-0.866019052628739));
#19572=DIRECTION('',(1.88173394004264E-16,-0.500011000363013,-0.866019052628739));
#19573=DIRECTION('',(1.,0.,0.));
#19574=DIRECTION('',(-1.88173394004264E-16,0.500011000363013,0.866019052628739));
#19575=DIRECTION('',(-1.,0.,0.));
#19576=DIRECTION('center_axis',(0.,-0.866019052628739,0.500011000363013));
#19577=DIRECTION('ref_axis',(0.,-0.500011000363013,-0.866019052628739));
#19578=DIRECTION('',(1.88173394004264E-16,-0.500011000363013,-0.866019052628739));
#19579=DIRECTION('',(-1.,0.,0.));
#19580=DIRECTION('',(-1.88173394004264E-16,0.500011000363013,0.866019052628739));
#19581=DIRECTION('',(1.,0.,0.));
#19582=DIRECTION('center_axis',(1.,9.40887669777753E-17,1.62961744405507E-16));
#19583=DIRECTION('ref_axis',(1.62961744405507E-16,0.,-1.));
#19584=DIRECTION('',(0.,0.866019052628739,-0.500011000363013));
#19585=DIRECTION('',(0.,0.866019052628739,-0.500011000363013));
#19586=DIRECTION('center_axis',(0.,0.500011000363013,0.866019052628739));
#19587=DIRECTION('ref_axis',(0.,-0.866019052628739,0.500011000363013));
#19588=DIRECTION('',(0.,0.866019052628739,-0.500011000363013));
#19589=DIRECTION('center_axis',(-1.,-9.40887669777753E-17,-1.62961744405507E-16));
#19590=DIRECTION('ref_axis',(-1.62961744405507E-16,0.,1.));
#19591=DIRECTION('',(0.,0.866019052628739,-0.500011000363013));
#19592=DIRECTION('center_axis',(0.,-0.500011000363013,-0.866019052628739));
#19593=DIRECTION('ref_axis',(0.,0.866019052628739,-0.500011000363013));
#19594=DIRECTION('center_axis',(5.44569658622596E-6,0.866021775511255,-0.500006284271186));
#19595=DIRECTION('ref_axis',(-0.999999999985172,4.71609182512488E-6,-2.72288251788859E-6));
#19596=DIRECTION('center_axis',(-5.44569658622596E-6,-0.866021775511255,
0.500006284271186));
#19597=DIRECTION('ref_axis',(0.999999999985172,-4.71609182512488E-6,2.72288251788859E-6));
#19598=DIRECTION('',(5.44569658622596E-6,0.866021775511255,-0.500006284271186));
#19599=DIRECTION('center_axis',(-5.44569658622596E-6,-0.866021775511255,
0.500006284271186));
#19600=DIRECTION('ref_axis',(0.999999999985172,-4.71609182512488E-6,2.72288251788859E-6));
#19601=DIRECTION('center_axis',(5.44569658622596E-6,0.866021775511255,-0.500006284271186));
#19602=DIRECTION('ref_axis',(-0.999999999985172,4.71609182512488E-6,-2.72288251788859E-6));
#19603=DIRECTION('center_axis',(-5.44569658622596E-6,-0.866021775511255,
0.500006284271186));
#19604=DIRECTION('ref_axis',(0.999999999985172,-4.71609182512488E-6,2.72288251788859E-6));
#19605=DIRECTION('',(5.44569658622596E-6,0.866021775511255,-0.500006284271186));
#19606=DIRECTION('center_axis',(-5.44569658622596E-6,-0.866021775511255,
0.500006284271186));
#19607=DIRECTION('ref_axis',(0.999999999985172,-4.71609182512488E-6,2.72288251788859E-6));
#19608=DIRECTION('center_axis',(5.44569658622596E-6,0.866021775511255,-0.500006284271186));
#19609=DIRECTION('ref_axis',(-0.999999999985172,4.71609182512488E-6,-2.72288251788859E-6));
#19610=DIRECTION('center_axis',(-5.44569658622596E-6,-0.866021775511255,
0.500006284271186));
#19611=DIRECTION('ref_axis',(0.999999999985172,-4.71609182512488E-6,2.72288251788859E-6));
#19612=DIRECTION('',(5.44569658622596E-6,0.866021775511255,-0.500006284271186));
#19613=DIRECTION('center_axis',(-5.44569658622596E-6,-0.866021775511255,
0.500006284271186));
#19614=DIRECTION('ref_axis',(0.999999999985172,-4.71609182512488E-6,2.72288251788859E-6));
#19615=DIRECTION('center_axis',(-5.44569658625102E-6,-0.866021775511255,
0.500006284271186));
#19616=DIRECTION('ref_axis',(0.999999999985172,-4.71609182484123E-6,2.72288251843E-6));
#19617=DIRECTION('',(0.999999999985172,-4.71609182473021E-6,2.72288251859654E-6));
#19618=DIRECTION('',(-3.49148133884313E-15,0.5000062842786,0.866021775524096));
#19619=DIRECTION('',(-0.999999999985172,4.71609182473021E-6,-2.72288251859654E-6));
#19620=DIRECTION('',(3.49148133884313E-15,-0.5000062842786,-0.866021775524096));
#19621=DIRECTION('center_axis',(-5.44569658625102E-6,-0.866021775511255,
0.500006284271186));
#19622=DIRECTION('ref_axis',(0.999999999985172,-4.71609182484123E-6,2.72288251843E-6));
#19623=DIRECTION('',(0.999999999985172,-4.71609182473021E-6,2.72288251859654E-6));
#19624=DIRECTION('',(3.49148133884313E-15,-0.5000062842786,-0.866021775524096));
#19625=DIRECTION('',(-0.999999999985172,4.71609182473021E-6,-2.72288251859654E-6));
#19626=DIRECTION('',(-3.49148133884313E-15,0.5000062842786,0.866021775524096));
#19627=DIRECTION('center_axis',(-3.71924713249427E-15,0.5000062842786,0.866021775524096));
#19628=DIRECTION('ref_axis',(0.866021775524096,0.433016330084161,-0.25000628431809));
#19629=DIRECTION('',(5.44569658622596E-6,0.866021775511255,-0.500006284271186));
#19630=DIRECTION('',(5.44569658622596E-6,0.866021775511255,-0.500006284271186));
#19631=DIRECTION('center_axis',(-0.999999999985172,4.71609182482138E-6,
-2.72288251841425E-6));
#19632=DIRECTION('ref_axis',(-5.44569658622595E-6,-0.866021775511255,0.500006284271186));
#19633=DIRECTION('',(5.44569658622596E-6,0.866021775511255,-0.500006284271186));
#19634=DIRECTION('center_axis',(3.71924713249427E-15,-0.5000062842786,-0.866021775524096));
#19635=DIRECTION('ref_axis',(-0.866021775524096,-0.433016330084161,0.25000628431809));
#19636=DIRECTION('',(5.44569658622596E-6,0.866021775511255,-0.500006284271186));
#19637=DIRECTION('center_axis',(0.999999999985172,-4.71609182482138E-6,
2.72288251841425E-6));
#19638=DIRECTION('ref_axis',(5.44569658622595E-6,0.866021775511255,-0.500006284271186));
#19639=DIRECTION('center_axis',(-2.79110278370762E-17,0.86602449839377,
-0.50000156817936));
#19640=DIRECTION('ref_axis',(6.68375889402081E-33,-0.50000156817936,-0.86602449839377));
#19641=DIRECTION('center_axis',(2.79110278370762E-17,-0.86602449839377,
0.50000156817936));
#19642=DIRECTION('ref_axis',(-6.68375889402081E-33,0.50000156817936,0.86602449839377));
#19643=DIRECTION('',(-2.79110278370762E-17,0.86602449839377,-0.50000156817936));
#19644=DIRECTION('center_axis',(2.79110278370762E-17,-0.86602449839377,
0.50000156817936));
#19645=DIRECTION('ref_axis',(-6.68375889402081E-33,0.50000156817936,0.86602449839377));
#19646=DIRECTION('center_axis',(-2.79110278370762E-17,0.86602449839377,
-0.50000156817936));
#19647=DIRECTION('ref_axis',(2.51726960247898E-32,-0.50000156817936,-0.86602449839377));
#19648=DIRECTION('center_axis',(2.79110278370762E-17,-0.86602449839377,
0.50000156817936));
#19649=DIRECTION('ref_axis',(-2.51726960247898E-32,0.50000156817936,0.86602449839377));
#19650=DIRECTION('',(-2.79110278370762E-17,0.86602449839377,-0.50000156817936));
#19651=DIRECTION('center_axis',(2.79110278370762E-17,-0.86602449839377,
0.50000156817936));
#19652=DIRECTION('ref_axis',(-2.51726960247898E-32,0.50000156817936,0.86602449839377));
#19653=DIRECTION('center_axis',(-2.79110278370762E-17,0.86602449839377,
-0.50000156817936));
#19654=DIRECTION('ref_axis',(-1.48866758124192E-32,-0.50000156817936,-0.86602449839377));
#19655=DIRECTION('center_axis',(2.79110278370762E-17,-0.86602449839377,
0.50000156817936));
#19656=DIRECTION('ref_axis',(1.48866758124192E-32,0.50000156817936,0.86602449839377));
#19657=DIRECTION('',(-2.79110278370762E-17,0.86602449839377,-0.50000156817936));
#19658=DIRECTION('center_axis',(2.79110278370762E-17,-0.86602449839377,
0.50000156817936));
#19659=DIRECTION('ref_axis',(1.48866758124192E-32,0.50000156817936,0.86602449839377));
#19660=DIRECTION('center_axis',(2.79110278370762E-17,-0.86602449839377,
0.50000156817936));
#19661=DIRECTION('ref_axis',(1.51994989013002E-22,0.50000156817936,0.86602449839377));
#19662=DIRECTION('',(-1.88173242009275E-16,0.50000156817936,0.86602449839377));
#19663=DIRECTION('',(-1.,-2.41715578845256E-17,1.395568931942E-17));
#19664=DIRECTION('',(1.88173242009275E-16,-0.50000156817936,-0.86602449839377));
#19665=DIRECTION('',(1.,2.41715578845256E-17,-1.395568931942E-17));
#19666=DIRECTION('center_axis',(2.79110278370762E-17,-0.86602449839377,
0.50000156817936));
#19667=DIRECTION('ref_axis',(1.51994989013002E-22,0.50000156817936,0.86602449839377));
#19668=DIRECTION('',(-1.88173242009275E-16,0.50000156817936,0.86602449839377));
#19669=DIRECTION('',(1.,2.41715578845256E-17,-1.395568931942E-17));
#19670=DIRECTION('',(1.88173242009275E-16,-0.50000156817936,-0.86602449839377));
#19671=DIRECTION('',(-1.,-2.41715578845256E-17,1.395568931942E-17));
#19672=DIRECTION('center_axis',(-1.,-1.1825854997629E-16,-1.49007079834176E-16));
#19673=DIRECTION('ref_axis',(-1.76917433724927E-16,0.866032660168318,0.499987431363815));
#19674=DIRECTION('',(-2.79110278370762E-17,0.86602449839377,-0.50000156817936));
#19675=DIRECTION('',(-2.79110278370762E-17,0.86602449839377,-0.50000156817936));
#19676=DIRECTION('center_axis',(-1.51994989007369E-22,-0.50000156817936,
-0.86602449839377));
#19677=DIRECTION('ref_axis',(2.79110278370762E-17,-0.86602449839377,0.50000156817936));
#19678=DIRECTION('',(-2.79110278370762E-17,0.86602449839377,-0.50000156817936));
#19679=DIRECTION('center_axis',(1.,1.1825854997629E-16,1.49007079834176E-16));
#19680=DIRECTION('ref_axis',(1.76917433724927E-16,-0.866032660168318,-0.499987431363815));
#19681=DIRECTION('',(-2.79110278370762E-17,0.86602449839377,-0.50000156817936));
#19682=DIRECTION('center_axis',(1.51994989007369E-22,0.50000156817936,0.86602449839377));
#19683=DIRECTION('ref_axis',(-2.79110278370762E-17,0.86602449839377,-0.50000156817936));
#19684=DIRECTION('center_axis',(-5.44569658622596E-6,0.866021775511255,
-0.500006284271186));
#19685=DIRECTION('ref_axis',(0.999999999985172,4.71609183046649E-6,-2.72288250863681E-6));
#19686=DIRECTION('center_axis',(5.44569658622596E-6,-0.866021775511255,
0.500006284271186));
#19687=DIRECTION('ref_axis',(-0.999999999985172,-4.71609183046649E-6,2.72288250863681E-6));
#19688=DIRECTION('',(-5.44569658622596E-6,0.866021775511255,-0.500006284271186));
#19689=DIRECTION('center_axis',(5.44569658622596E-6,-0.866021775511255,
0.500006284271186));
#19690=DIRECTION('ref_axis',(-0.999999999985172,-4.71609183046649E-6,2.72288250863681E-6));
#19691=DIRECTION('center_axis',(-5.44569658622596E-6,0.866021775511255,
-0.500006284271186));
#19692=DIRECTION('ref_axis',(0.999999999985172,4.71609183046649E-6,-2.72288250863681E-6));
#19693=DIRECTION('center_axis',(5.44569658622596E-6,-0.866021775511255,
0.500006284271186));
#19694=DIRECTION('ref_axis',(-0.999999999985172,-4.71609183046649E-6,2.72288250863681E-6));
#19695=DIRECTION('',(-5.44569658622596E-6,0.866021775511255,-0.500006284271186));
#19696=DIRECTION('center_axis',(5.44569658622596E-6,-0.866021775511255,
0.500006284271186));
#19697=DIRECTION('ref_axis',(-0.999999999985172,-4.71609183046649E-6,2.72288250863681E-6));
#19698=DIRECTION('center_axis',(-5.44569658622596E-6,0.866021775511255,
-0.500006284271186));
#19699=DIRECTION('ref_axis',(0.999999999985172,4.71609183046649E-6,-2.72288250863681E-6));
#19700=DIRECTION('center_axis',(5.44569658622596E-6,-0.866021775511255,
0.500006284271186));
#19701=DIRECTION('ref_axis',(-0.999999999985172,-4.71609183046649E-6,2.72288250863681E-6));
#19702=DIRECTION('',(-5.44569658622596E-6,0.866021775511255,-0.500006284271186));
#19703=DIRECTION('center_axis',(5.44569658622596E-6,-0.866021775511255,
0.500006284271186));
#19704=DIRECTION('ref_axis',(-0.999999999985172,-4.71609183046649E-6,2.72288250863681E-6));
#19705=DIRECTION('center_axis',(5.44569658619558E-6,-0.866021775511255,
0.500006284271186));
#19706=DIRECTION('ref_axis',(-0.999999999985172,-4.71609183178012E-6,2.72288250630082E-6));
#19707=DIRECTION('',(-0.999999999985172,-4.71609183189114E-6,2.72288250613428E-6));
#19708=DIRECTION('',(1.04744440165294E-14,-0.5000062842786,-0.866021775524096));
#19709=DIRECTION('',(0.999999999985172,4.71609183189114E-6,-2.72288250613428E-6));
#19710=DIRECTION('',(-1.04744440165294E-14,0.5000062842786,0.866021775524096));
#19711=DIRECTION('center_axis',(5.44569658619558E-6,-0.866021775511255,
0.500006284271186));
#19712=DIRECTION('ref_axis',(-0.999999999985172,-4.71609183178012E-6,2.72288250630082E-6));
#19713=DIRECTION('',(-0.999999999985172,-4.71609183189114E-6,2.72288250613428E-6));
#19714=DIRECTION('',(-1.04744440165294E-14,0.5000062842786,0.866021775524096));
#19715=DIRECTION('',(0.999999999985172,4.71609183189114E-6,-2.72288250613428E-6));
#19716=DIRECTION('',(1.04744440165294E-14,-0.5000062842786,-0.866021775524096));
#19717=DIRECTION('center_axis',(1.06303854607859E-14,-0.5000062842786,-0.866021775524096));
#19718=DIRECTION('ref_axis',(-0.866021775524096,0.433016330084155,-0.2500062843181));
#19719=DIRECTION('',(-5.44569658622596E-6,0.866021775511255,-0.500006284271186));
#19720=DIRECTION('',(-5.44569658622596E-6,0.866021775511255,-0.500006284271186));
#19721=DIRECTION('center_axis',(0.999999999985172,4.71609183179441E-6,-2.72288250633682E-6));
#19722=DIRECTION('ref_axis',(5.44569658622596E-6,-0.866021775511255,0.500006284271186));
#19723=DIRECTION('',(-5.44569658622596E-6,0.866021775511255,-0.500006284271186));
#19724=DIRECTION('center_axis',(-1.06303854607859E-14,0.5000062842786,0.866021775524096));
#19725=DIRECTION('ref_axis',(0.866021775524096,-0.433016330084155,0.2500062843181));
#19726=DIRECTION('',(-5.44569658622596E-6,0.866021775511255,-0.500006284271186));
#19727=DIRECTION('center_axis',(-0.999999999985172,-4.71609183179441E-6,
2.72288250633682E-6));
#19728=DIRECTION('ref_axis',(-5.44569658622596E-6,0.866021775511255,-0.500006284271186));
#19729=DIRECTION('center_axis',(-9.439207419131E-6,0.500006284256325,0.866021775485516));
#19730=DIRECTION('ref_axis',(-5.27658532184428E-22,-0.866021775524096,0.5000062842786));
#19731=DIRECTION('',(-0.499722453400429,0.750133220675019,-0.4331023214059));
#19732=DIRECTION('',(0.866185586048601,0.432774614486463,-0.249857286421141));
#19733=DIRECTION('',(-0.499722453400429,0.750133220675019,-0.4331023214059));
#19734=DIRECTION('',(0.866185586048601,0.432774614486463,-0.249857286421141));
#19735=DIRECTION('center_axis',(0.499722453400429,-0.750133220675019,0.4331023214059));
#19736=DIRECTION('ref_axis',(-0.832237843570743,-0.55441876927889,-3.50686665358977E-17));
#19737=DIRECTION('',(-9.43920741954911E-6,0.500006284256325,0.866021775485515));
#19738=DIRECTION('',(-9.43920741954911E-6,0.500006284256325,0.866021775485515));
#19739=DIRECTION('',(0.866185586048601,0.432774614486463,-0.249857286421141));
#19740=DIRECTION('center_axis',(9.43920741930175E-6,-0.500006284256325,
-0.866021775485516));
#19741=DIRECTION('ref_axis',(2.61520069381354E-22,0.866021775524096,-0.5000062842786));
#19742=DIRECTION('',(0.499722453400429,-0.750133220675019,0.4331023214059));
#19743=DIRECTION('',(0.499722453400429,-0.750133220675019,0.4331023214059));
#19744=DIRECTION('',(0.866185586048601,0.432774614486463,-0.249857286421141));
#19745=DIRECTION('center_axis',(-0.499722453400429,0.750133220675019,-0.4331023214059));
#19746=DIRECTION('ref_axis',(0.832237843570743,0.55441876927889,2.11982739611214E-17));
#19747=DIRECTION('',(9.43920741954911E-6,-0.500006284256325,-0.866021775485515));
#19748=DIRECTION('',(9.43920741954911E-6,-0.500006284256325,-0.866021775485515));
#19749=DIRECTION('center_axis',(0.866185586048601,0.432774614486463,-0.249857286421141));
#19750=DIRECTION('ref_axis',(0.446950695480887,-0.89455859271998,-4.18661307789075E-19));
#19751=DIRECTION('center_axis',(0.866185586048601,0.432774614486463,-0.249857286421141));
#19752=DIRECTION('ref_axis',(0.446950695480887,-0.89455859271998,-4.18661307789075E-19));
#19753=DIRECTION('center_axis',(0.,0.500011000363013,0.866019052628739));
#19754=DIRECTION('ref_axis',(0.,-0.866019052628739,0.500011000363013));
#19755=DIRECTION('',(0.,0.866019052628739,-0.500011000363013));
#19756=DIRECTION('',(1.,0.,0.));
#19757=DIRECTION('',(0.,0.866019052628739,-0.500011000363013));
#19758=DIRECTION('',(1.,0.,0.));
#19759=DIRECTION('center_axis',(0.,-0.866019052628739,0.500011000363013));
#19760=DIRECTION('ref_axis',(0.,-0.500011000363013,-0.866019052628739));
#19761=DIRECTION('',(0.,0.500011000363013,0.866019052628739));
#19762=DIRECTION('',(0.,0.500011000363013,0.866019052628739));
#19763=DIRECTION('',(1.,0.,0.));
#19764=DIRECTION('center_axis',(0.,-0.500011000363012,-0.86601905262874));
#19765=DIRECTION('ref_axis',(0.,0.86601905262874,-0.500011000363012));
#19766=DIRECTION('',(0.,-0.86601905262874,0.500011000363011));
#19767=DIRECTION('',(0.,-0.86601905262874,0.500011000363011));
#19768=DIRECTION('',(1.,0.,0.));
#19769=DIRECTION('center_axis',(0.,0.866019052628739,-0.500011000363013));
#19770=DIRECTION('ref_axis',(0.,0.500011000363013,0.866019052628739));
#19771=DIRECTION('',(0.,-0.500011000363013,-0.866019052628739));
#19772=DIRECTION('',(0.,-0.500011000363013,-0.866019052628739));
#19773=DIRECTION('center_axis',(-1.,0.,0.));
#19774=DIRECTION('ref_axis',(0.,0.,-1.));
#19775=DIRECTION('center_axis',(-1.,0.,0.));
#19776=DIRECTION('ref_axis',(0.,0.,-1.));
#19777=DIRECTION('center_axis',(1.,0.,0.));
#19778=DIRECTION('ref_axis',(0.,0.,-1.));
#19779=DIRECTION('',(0.,0.,1.));
#19780=DIRECTION('',(0.,-1.,0.));
#19781=DIRECTION('',(0.,0.,1.));
#19782=DIRECTION('',(0.,-1.,0.));
#19783=DIRECTION('center_axis',(0.,0.,-1.));
#19784=DIRECTION('ref_axis',(-1.,0.,0.));
#19785=DIRECTION('',(1.,0.,0.));
#19786=DIRECTION('',(0.,-1.,0.));
#19787=DIRECTION('',(1.,0.,0.));
#19788=DIRECTION('center_axis',(-1.,0.,0.));
#19789=DIRECTION('ref_axis',(0.,0.,1.));
#19790=DIRECTION('',(0.,0.,-1.));
#19791=DIRECTION('',(0.,-1.,0.));
#19792=DIRECTION('',(0.,0.,-1.));
#19793=DIRECTION('center_axis',(0.,0.,1.));
#19794=DIRECTION('ref_axis',(1.,0.,0.));
#19795=DIRECTION('',(-1.,0.,0.));
#19796=DIRECTION('',(-1.,0.,0.));
#19797=DIRECTION('center_axis',(0.,-1.,0.));
#19798=DIRECTION('ref_axis',(0.,0.,-1.));
#19799=DIRECTION('center_axis',(0.,-1.,0.));
#19800=DIRECTION('ref_axis',(0.,0.,-1.));
#19801=DIRECTION('center_axis',(-1.,0.,0.));
#19802=DIRECTION('ref_axis',(0.,0.,1.));
#19803=DIRECTION('',(0.,0.,1.));
#19804=DIRECTION('',(0.,1.,0.));
#19805=DIRECTION('',(0.,0.,1.));
#19806=DIRECTION('',(0.,1.,0.));
#19807=DIRECTION('center_axis',(-1.09275353725347E-14,0.,-1.));
#19808=DIRECTION('ref_axis',(-1.,0.,1.09275353725347E-14));
#19809=DIRECTION('',(-1.,0.,1.09275353725347E-14));
#19810=DIRECTION('',(0.,1.,0.));
#19811=DIRECTION('',(-1.,0.,1.09275353725347E-14));
#19812=DIRECTION('center_axis',(1.,0.,-1.04157383973362E-14));
#19813=DIRECTION('ref_axis',(-1.04157383973362E-14,0.,-1.));
#19814=DIRECTION('',(-1.04157383973362E-14,0.,-1.));
#19815=DIRECTION('',(0.,1.,0.));
#19816=DIRECTION('',(-1.04157383973362E-14,0.,-1.));
#19817=DIRECTION('center_axis',(0.,0.,1.));
#19818=DIRECTION('ref_axis',(1.,0.,0.));
#19819=DIRECTION('',(1.,0.,0.));
#19820=DIRECTION('',(1.,0.,0.));
#19821=DIRECTION('center_axis',(0.,1.,0.));
#19822=DIRECTION('ref_axis',(0.,0.,1.));
#19823=DIRECTION('center_axis',(0.,1.,0.));
#19824=DIRECTION('ref_axis',(0.,0.,1.));
#19825=DIRECTION('center_axis',(1.,0.,0.));
#19826=DIRECTION('ref_axis',(0.,0.,1.));
#19827=DIRECTION('',(0.,0.,1.));
#19828=DIRECTION('',(0.,1.,0.));
#19829=DIRECTION('',(0.,0.,1.));
#19830=DIRECTION('',(0.,1.,0.));
#19831=DIRECTION('center_axis',(1.09275353725347E-14,0.,-1.));
#19832=DIRECTION('ref_axis',(1.,0.,1.09275353725347E-14));
#19833=DIRECTION('',(1.,0.,1.09275353725347E-14));
#19834=DIRECTION('',(1.,0.,1.09275353725347E-14));
#19835=DIRECTION('',(0.,1.,0.));
#19836=DIRECTION('center_axis',(-1.,0.,-1.04157383973362E-14));
#19837=DIRECTION('ref_axis',(1.04157383973362E-14,0.,-1.));
#19838=DIRECTION('',(1.04157383973362E-14,0.,-1.));
#19839=DIRECTION('',(1.04157383973362E-14,0.,-1.));
#19840=DIRECTION('',(0.,1.,0.));
#19841=DIRECTION('center_axis',(0.,0.,1.));
#19842=DIRECTION('ref_axis',(-1.,0.,0.));
#19843=DIRECTION('',(-1.,0.,0.));
#19844=DIRECTION('',(-1.,0.,0.));
#19845=DIRECTION('center_axis',(0.,1.,0.));
#19846=DIRECTION('ref_axis',(0.,0.,1.));
#19847=DIRECTION('center_axis',(0.,1.,0.));
#19848=DIRECTION('ref_axis',(0.,0.,1.));
#19849=DIRECTION('center_axis',(0.,1.,0.));
#19850=DIRECTION('ref_axis',(0.,0.,1.));
#19851=DIRECTION('center_axis',(0.,-1.,0.));
#19852=DIRECTION('ref_axis',(0.,0.,-1.));
#19853=DIRECTION('',(0.,1.,0.));
#19854=DIRECTION('center_axis',(0.,-1.,0.));
#19855=DIRECTION('ref_axis',(0.,0.,-1.));
#19856=DIRECTION('center_axis',(0.,1.,0.));
#19857=DIRECTION('ref_axis',(0.,0.,1.));
#19858=DIRECTION('center_axis',(0.,-1.,0.));
#19859=DIRECTION('ref_axis',(0.,0.,-1.));
#19860=DIRECTION('',(0.,1.,0.));
#19861=DIRECTION('center_axis',(0.,-1.,0.));
#19862=DIRECTION('ref_axis',(0.,0.,-1.));
#19863=DIRECTION('center_axis',(0.,1.,0.));
#19864=DIRECTION('ref_axis',(0.,0.,1.));
#19865=DIRECTION('center_axis',(0.,-1.,0.));
#19866=DIRECTION('ref_axis',(0.,0.,-1.));
#19867=DIRECTION('',(0.,1.,0.));
#19868=DIRECTION('center_axis',(0.,-1.,0.));
#19869=DIRECTION('ref_axis',(0.,0.,-1.));
#19870=DIRECTION('center_axis',(0.,1.,0.));
#19871=DIRECTION('ref_axis',(0.,0.,1.));
#19872=DIRECTION('center_axis',(0.,-1.,0.));
#19873=DIRECTION('ref_axis',(0.,0.,-1.));
#19874=DIRECTION('',(0.,1.,0.));
#19875=DIRECTION('center_axis',(0.,-1.,0.));
#19876=DIRECTION('ref_axis',(0.,0.,-1.));
#19877=DIRECTION('center_axis',(0.,1.,0.));
#19878=DIRECTION('ref_axis',(0.,0.,1.));
#19879=DIRECTION('',(2.36721327212187E-16,0.,-1.));
#19880=DIRECTION('',(1.,0.,-3.03339624214524E-16));
#19881=DIRECTION('',(-2.36721327212187E-16,0.,1.));
#19882=DIRECTION('',(-1.,0.,-1.13752359080446E-16));
#19883=DIRECTION('center_axis',(0.,1.,0.));
#19884=DIRECTION('ref_axis',(0.,0.,1.));
#19885=DIRECTION('',(2.36721327212187E-16,0.,-1.));
#19886=DIRECTION('',(-1.,0.,-1.13752359080446E-16));
#19887=DIRECTION('',(-2.36721327212187E-16,0.,1.));
#19888=DIRECTION('',(1.,0.,-3.03339624214524E-16));
#19889=DIRECTION('center_axis',(1.,0.,2.36721327212187E-16));
#19890=DIRECTION('ref_axis',(2.36721327212187E-16,0.,-1.));
#19891=DIRECTION('',(0.,1.,0.));
#19892=DIRECTION('',(0.,1.,0.));
#19893=DIRECTION('center_axis',(3.03339624214524E-16,0.,1.));
#19894=DIRECTION('ref_axis',(1.,0.,-3.03339624214524E-16));
#19895=DIRECTION('',(0.,1.,0.));
#19896=DIRECTION('center_axis',(-1.,0.,-2.36721327212187E-16));
#19897=DIRECTION('ref_axis',(-2.36721327212187E-16,0.,1.));
#19898=DIRECTION('',(0.,1.,0.));
#19899=DIRECTION('center_axis',(1.13752359080446E-16,0.,-1.));
#19900=DIRECTION('ref_axis',(-1.,0.,-1.13752359080446E-16));
#19901=DIRECTION('center_axis',(0.,-1.,0.));
#19902=DIRECTION('ref_axis',(0.,0.,-1.));
#19903=DIRECTION('center_axis',(0.,-1.,0.));
#19904=DIRECTION('ref_axis',(0.,0.,-1.));
#19905=DIRECTION('',(0.,-1.,0.));
#19906=DIRECTION('center_axis',(0.,-1.,0.));
#19907=DIRECTION('ref_axis',(0.,0.,-1.));
#19908=DIRECTION('center_axis',(0.,-1.,0.));
#19909=DIRECTION('ref_axis',(0.,0.,-1.));
#19910=DIRECTION('center_axis',(0.,-1.,0.));
#19911=DIRECTION('ref_axis',(0.,0.,-1.));
#19912=DIRECTION('',(0.,-1.,0.));
#19913=DIRECTION('center_axis',(0.,-1.,0.));
#19914=DIRECTION('ref_axis',(0.,0.,-1.));
#19915=DIRECTION('center_axis',(0.,-1.,0.));
#19916=DIRECTION('ref_axis',(0.,0.,-1.));
#19917=DIRECTION('center_axis',(0.,-1.,0.));
#19918=DIRECTION('ref_axis',(0.,0.,-1.));
#19919=DIRECTION('',(0.,-1.,0.));
#19920=DIRECTION('center_axis',(0.,-1.,0.));
#19921=DIRECTION('ref_axis',(0.,0.,-1.));
#19922=DIRECTION('center_axis',(0.,-1.,0.));
#19923=DIRECTION('ref_axis',(0.,0.,-1.));
#19924=DIRECTION('center_axis',(0.,-1.,0.));
#19925=DIRECTION('ref_axis',(0.,0.,-1.));
#19926=DIRECTION('',(0.,-1.,0.));
#19927=DIRECTION('center_axis',(0.,-1.,0.));
#19928=DIRECTION('ref_axis',(0.,0.,-1.));
#19929=DIRECTION('center_axis',(0.,-1.,0.));
#19930=DIRECTION('ref_axis',(0.,0.,-1.));
#19931=DIRECTION('center_axis',(0.,-1.,0.));
#19932=DIRECTION('ref_axis',(0.,0.,-1.));
#19933=DIRECTION('',(0.,-1.,0.));
#19934=DIRECTION('center_axis',(0.,-1.,0.));
#19935=DIRECTION('ref_axis',(0.,0.,-1.));
#19936=DIRECTION('center_axis',(0.,-1.,0.));
#19937=DIRECTION('ref_axis',(0.,0.,-1.));
#19938=DIRECTION('center_axis',(0.,-1.,0.));
#19939=DIRECTION('ref_axis',(0.,0.,-1.));
#19940=DIRECTION('',(0.,-1.,0.));
#19941=DIRECTION('center_axis',(0.,-1.,0.));
#19942=DIRECTION('ref_axis',(0.,0.,-1.));
#19943=DIRECTION('center_axis',(1.,0.,0.));
#19944=DIRECTION('ref_axis',(0.,0.,-1.));
#19945=DIRECTION('',(0.,0.,1.));
#19946=DIRECTION('',(0.,-1.,0.));
#19947=DIRECTION('',(0.,0.,1.));
#19948=DIRECTION('',(0.,-1.,0.));
#19949=DIRECTION('center_axis',(1.22307178094722E-16,0.,-1.));
#19950=DIRECTION('ref_axis',(-1.,0.,-1.22307178094722E-16));
#19951=DIRECTION('',(1.,0.,1.22307178094722E-16));
#19952=DIRECTION('',(0.,-1.,0.));
#19953=DIRECTION('',(1.,0.,1.22307178094722E-16));
#19954=DIRECTION('center_axis',(-1.,0.,0.));
#19955=DIRECTION('ref_axis',(0.,0.,1.));
#19956=DIRECTION('',(0.,0.,-1.));
#19957=DIRECTION('',(0.,-1.,0.));
#19958=DIRECTION('',(0.,0.,-1.));
#19959=DIRECTION('center_axis',(-9.31864214055025E-17,0.,1.));
#19960=DIRECTION('ref_axis',(1.,0.,9.31864214055025E-17));
#19961=DIRECTION('',(-1.,0.,-9.31864214055025E-17));
#19962=DIRECTION('',(-1.,0.,-9.31864214055025E-17));
#19963=DIRECTION('center_axis',(0.,-1.,0.));
#19964=DIRECTION('ref_axis',(0.,0.,-1.));
#19965=DIRECTION('center_axis',(0.,-1.,0.));
#19966=DIRECTION('ref_axis',(0.,0.,-1.));
#19967=DIRECTION('center_axis',(-0.400352069216121,-0.916361402872453,0.));
#19968=DIRECTION('ref_axis',(0.916361402872453,-0.400352069216121,0.));
#19969=DIRECTION('',(0.916361402872453,-0.400352069216121,0.));
#19970=DIRECTION('',(0.,0.,1.));
#19971=DIRECTION('',(0.916361402872453,-0.400352069216121,0.));
#19972=DIRECTION('',(0.,0.,1.));
#19973=DIRECTION('center_axis',(-1.,0.,0.));
#19974=DIRECTION('ref_axis',(0.,0.,1.));
#19975=DIRECTION('',(0.,-1.,0.));
#19976=DIRECTION('',(0.,0.,1.));
#19977=DIRECTION('',(0.,-1.,0.));
#19978=DIRECTION('center_axis',(1.92747052886312E-16,1.,0.));
#19979=DIRECTION('ref_axis',(-1.,1.92747052886312E-16,0.));
#19980=DIRECTION('',(-1.,1.92747052886312E-16,0.));
#19981=DIRECTION('',(0.,0.,1.));
#19982=DIRECTION('',(-1.,1.92747052886312E-16,0.));
#19983=DIRECTION('center_axis',(0.707106781186551,0.707106781186544,0.));
#19984=DIRECTION('ref_axis',(-0.707106781186544,0.707106781186551,0.));
#19985=DIRECTION('',(-0.707106781186544,0.707106781186551,0.));
#19986=DIRECTION('',(0.,0.,1.));
#19987=DIRECTION('',(-0.707106781186544,0.707106781186551,0.));
#19988=DIRECTION('center_axis',(1.,0.,0.));
#19989=DIRECTION('ref_axis',(0.,0.,-1.));
#19990=DIRECTION('',(0.,1.,0.));
#19991=DIRECTION('',(0.,0.,1.));
#19992=DIRECTION('',(0.,1.,0.));
#19993=DIRECTION('center_axis',(0.707106781186546,-0.707106781186549,0.));
#19994=DIRECTION('ref_axis',(0.707106781186549,0.707106781186546,0.));
#19995=DIRECTION('',(0.707106781186549,0.707106781186546,0.));
#19996=DIRECTION('',(0.,0.,1.));
#19997=DIRECTION('',(0.707106781186549,0.707106781186546,0.));
#19998=DIRECTION('center_axis',(1.35393051783556E-15,-1.,0.));
#19999=DIRECTION('ref_axis',(1.,1.35393051783556E-15,0.));
#20000=DIRECTION('',(1.,1.35393051783556E-15,0.));
#20001=DIRECTION('',(1.,1.35393051783556E-15,0.));
#20002=DIRECTION('center_axis',(0.,0.,1.));
#20003=DIRECTION('ref_axis',(1.,0.,0.));
#20004=DIRECTION('center_axis',(0.,0.,1.));
#20005=DIRECTION('ref_axis',(1.,0.,0.));
#20006=DIRECTION('center_axis',(-0.400352069216121,-0.916361402872453,0.));
#20007=DIRECTION('ref_axis',(0.916361402872453,-0.400352069216121,0.));
#20008=DIRECTION('',(0.916361402872453,-0.400352069216121,0.));
#20009=DIRECTION('',(0.,0.,1.));
#20010=DIRECTION('',(0.916361402872453,-0.400352069216121,0.));
#20011=DIRECTION('',(0.,0.,1.));
#20012=DIRECTION('center_axis',(-1.,0.,0.));
#20013=DIRECTION('ref_axis',(0.,0.,1.));
#20014=DIRECTION('',(0.,-1.,0.));
#20015=DIRECTION('',(0.,0.,1.));
#20016=DIRECTION('',(0.,-1.,0.));
#20017=DIRECTION('center_axis',(1.92747052886312E-16,1.,0.));
#20018=DIRECTION('ref_axis',(-1.,1.92747052886312E-16,0.));
#20019=DIRECTION('',(-1.,1.92747052886312E-16,0.));
#20020=DIRECTION('',(0.,0.,1.));
#20021=DIRECTION('',(-1.,1.92747052886312E-16,0.));
#20022=DIRECTION('center_axis',(0.707106781186551,0.707106781186544,0.));
#20023=DIRECTION('ref_axis',(-0.707106781186544,0.707106781186551,0.));
#20024=DIRECTION('',(-0.707106781186544,0.707106781186551,0.));
#20025=DIRECTION('',(0.,0.,1.));
#20026=DIRECTION('',(-0.707106781186544,0.707106781186551,0.));
#20027=DIRECTION('center_axis',(1.,0.,0.));
#20028=DIRECTION('ref_axis',(0.,0.,-1.));
#20029=DIRECTION('',(0.,1.,0.));
#20030=DIRECTION('',(0.,0.,1.));
#20031=DIRECTION('',(0.,1.,0.));
#20032=DIRECTION('center_axis',(0.707106781186546,-0.707106781186549,0.));
#20033=DIRECTION('ref_axis',(0.707106781186549,0.707106781186546,0.));
#20034=DIRECTION('',(0.707106781186549,0.707106781186546,0.));
#20035=DIRECTION('',(0.,0.,1.));
#20036=DIRECTION('',(0.707106781186549,0.707106781186546,0.));
#20037=DIRECTION('center_axis',(1.35393051783556E-15,-1.,0.));
#20038=DIRECTION('ref_axis',(1.,1.35393051783556E-15,0.));
#20039=DIRECTION('',(1.,1.35393051783556E-15,0.));
#20040=DIRECTION('',(1.,1.35393051783556E-15,0.));
#20041=DIRECTION('center_axis',(0.,0.,1.));
#20042=DIRECTION('ref_axis',(1.,0.,0.));
#20043=DIRECTION('center_axis',(0.,0.,1.));
#20044=DIRECTION('ref_axis',(1.,0.,0.));
#20045=DIRECTION('center_axis',(-0.400352069216121,-0.916361402872453,0.));
#20046=DIRECTION('ref_axis',(0.916361402872453,-0.400352069216121,0.));
#20047=DIRECTION('',(0.916361402872453,-0.400352069216121,0.));
#20048=DIRECTION('',(0.,0.,1.));
#20049=DIRECTION('',(0.916361402872453,-0.400352069216121,0.));
#20050=DIRECTION('',(0.,0.,1.));
#20051=DIRECTION('center_axis',(-1.,0.,0.));
#20052=DIRECTION('ref_axis',(0.,0.,1.));
#20053=DIRECTION('',(0.,-1.,0.));
#20054=DIRECTION('',(0.,0.,1.));
#20055=DIRECTION('',(0.,-1.,0.));
#20056=DIRECTION('center_axis',(1.92747052886312E-16,1.,0.));
#20057=DIRECTION('ref_axis',(-1.,1.92747052886312E-16,0.));
#20058=DIRECTION('',(-1.,1.92747052886312E-16,0.));
#20059=DIRECTION('',(0.,0.,1.));
#20060=DIRECTION('',(-1.,1.92747052886312E-16,0.));
#20061=DIRECTION('center_axis',(0.707106781186551,0.707106781186544,0.));
#20062=DIRECTION('ref_axis',(-0.707106781186544,0.707106781186551,0.));
#20063=DIRECTION('',(-0.707106781186544,0.707106781186551,0.));
#20064=DIRECTION('',(0.,0.,1.));
#20065=DIRECTION('',(-0.707106781186544,0.707106781186551,0.));
#20066=DIRECTION('center_axis',(1.,0.,0.));
#20067=DIRECTION('ref_axis',(0.,0.,-1.));
#20068=DIRECTION('',(0.,1.,0.));
#20069=DIRECTION('',(0.,0.,1.));
#20070=DIRECTION('',(0.,1.,0.));
#20071=DIRECTION('center_axis',(0.707106781186546,-0.707106781186549,0.));
#20072=DIRECTION('ref_axis',(0.707106781186549,0.707106781186546,0.));
#20073=DIRECTION('',(0.707106781186549,0.707106781186546,0.));
#20074=DIRECTION('',(0.,0.,1.));
#20075=DIRECTION('',(0.707106781186549,0.707106781186546,0.));
#20076=DIRECTION('center_axis',(1.35393051783556E-15,-1.,0.));
#20077=DIRECTION('ref_axis',(1.,1.35393051783556E-15,0.));
#20078=DIRECTION('',(1.,1.35393051783556E-15,0.));
#20079=DIRECTION('',(1.,1.35393051783556E-15,0.));
#20080=DIRECTION('center_axis',(0.,0.,1.));
#20081=DIRECTION('ref_axis',(1.,0.,0.));
#20082=DIRECTION('center_axis',(0.,0.,1.));
#20083=DIRECTION('ref_axis',(1.,0.,0.));
#20084=DIRECTION('center_axis',(0.,0.886474799840877,0.462776867666349));
#20085=DIRECTION('ref_axis',(0.,-0.462776867666349,0.886474799840877));
#20086=DIRECTION('',(0.,-0.462776867666349,0.886474799840877));
#20087=DIRECTION('',(1.,0.,0.));
#20088=DIRECTION('',(0.,-0.462776867666349,0.886474799840877));
#20089=DIRECTION('',(1.,0.,0.));
#20090=DIRECTION('center_axis',(0.,1.,0.));
#20091=DIRECTION('ref_axis',(0.,0.,1.));
#20092=DIRECTION('',(0.,0.,1.));
#20093=DIRECTION('',(1.,0.,0.));
#20094=DIRECTION('',(0.,0.,1.));
#20095=DIRECTION('center_axis',(0.,0.707106781186542,-0.707106781186553));
#20096=DIRECTION('ref_axis',(0.,0.707106781186553,0.707106781186542));
#20097=DIRECTION('',(0.,0.707106781186553,0.707106781186542));
#20098=DIRECTION('',(1.,0.,0.));
#20099=DIRECTION('',(0.,0.707106781186553,0.707106781186542));
#20100=DIRECTION('center_axis',(0.,0.,-1.));
#20101=DIRECTION('ref_axis',(-1.,0.,0.));
#20102=DIRECTION('',(0.,1.,0.));
#20103=DIRECTION('',(1.,0.,0.));
#20104=DIRECTION('',(0.,1.,0.));
#20105=DIRECTION('center_axis',(0.,-0.707106781186547,-0.707106781186548));
#20106=DIRECTION('ref_axis',(0.,0.707106781186548,-0.707106781186547));
#20107=DIRECTION('',(0.,0.707106781186548,-0.707106781186547));
#20108=DIRECTION('',(1.,0.,0.));
#20109=DIRECTION('',(0.,0.707106781186548,-0.707106781186547));
#20110=DIRECTION('center_axis',(0.,-1.,0.));
#20111=DIRECTION('ref_axis',(0.,0.,-1.));
#20112=DIRECTION('',(0.,0.,-1.));
#20113=DIRECTION('',(1.,0.,0.));
#20114=DIRECTION('',(0.,0.,-1.));
#20115=DIRECTION('center_axis',(0.,0.,1.));
#20116=DIRECTION('ref_axis',(1.,0.,0.));
#20117=DIRECTION('',(0.,-1.,0.));
#20118=DIRECTION('',(0.,-1.,0.));
#20119=DIRECTION('center_axis',(-1.,0.,0.));
#20120=DIRECTION('ref_axis',(0.,0.,1.));
#20121=DIRECTION('center_axis',(-1.,0.,0.));
#20122=DIRECTION('ref_axis',(0.,0.,1.));
#20123=DIRECTION('center_axis',(0.,0.886474799840877,0.462776867666349));
#20124=DIRECTION('ref_axis',(0.,-0.462776867666349,0.886474799840877));
#20125=DIRECTION('',(0.,-0.462776867666349,0.886474799840877));
#20126=DIRECTION('',(1.,0.,0.));
#20127=DIRECTION('',(0.,-0.462776867666349,0.886474799840877));
#20128=DIRECTION('',(1.,0.,0.));
#20129=DIRECTION('center_axis',(0.,1.,0.));
#20130=DIRECTION('ref_axis',(0.,0.,1.));
#20131=DIRECTION('',(0.,0.,1.));
#20132=DIRECTION('',(1.,0.,0.));
#20133=DIRECTION('',(0.,0.,1.));
#20134=DIRECTION('center_axis',(0.,0.707106781186542,-0.707106781186553));
#20135=DIRECTION('ref_axis',(0.,0.707106781186553,0.707106781186542));
#20136=DIRECTION('',(0.,0.707106781186553,0.707106781186542));
#20137=DIRECTION('',(1.,0.,0.));
#20138=DIRECTION('',(0.,0.707106781186553,0.707106781186542));
#20139=DIRECTION('center_axis',(0.,0.,-1.));
#20140=DIRECTION('ref_axis',(-1.,0.,0.));
#20141=DIRECTION('',(0.,1.,0.));
#20142=DIRECTION('',(1.,0.,0.));
#20143=DIRECTION('',(0.,1.,0.));
#20144=DIRECTION('center_axis',(0.,-0.707106781186547,-0.707106781186548));
#20145=DIRECTION('ref_axis',(0.,0.707106781186548,-0.707106781186547));
#20146=DIRECTION('',(0.,0.707106781186548,-0.707106781186547));
#20147=DIRECTION('',(1.,0.,0.));
#20148=DIRECTION('',(0.,0.707106781186548,-0.707106781186547));
#20149=DIRECTION('center_axis',(0.,-1.,0.));
#20150=DIRECTION('ref_axis',(0.,0.,-1.));
#20151=DIRECTION('',(0.,0.,-1.));
#20152=DIRECTION('',(1.,0.,0.));
#20153=DIRECTION('',(0.,0.,-1.));
#20154=DIRECTION('center_axis',(0.,0.,1.));
#20155=DIRECTION('ref_axis',(1.,0.,0.));
#20156=DIRECTION('',(0.,-1.,0.));
#20157=DIRECTION('',(0.,-1.,0.));
#20158=DIRECTION('center_axis',(-1.,0.,0.));
#20159=DIRECTION('ref_axis',(0.,0.,1.));
#20160=DIRECTION('center_axis',(-1.,0.,0.));
#20161=DIRECTION('ref_axis',(0.,0.,1.));
#20162=DIRECTION('center_axis',(0.,0.886474799840877,0.462776867666349));
#20163=DIRECTION('ref_axis',(0.,-0.462776867666349,0.886474799840877));
#20164=DIRECTION('',(0.,-0.462776867666349,0.886474799840877));
#20165=DIRECTION('',(1.,0.,0.));
#20166=DIRECTION('',(0.,-0.462776867666349,0.886474799840877));
#20167=DIRECTION('',(1.,0.,0.));
#20168=DIRECTION('center_axis',(0.,1.,0.));
#20169=DIRECTION('ref_axis',(0.,0.,1.));
#20170=DIRECTION('',(0.,0.,1.));
#20171=DIRECTION('',(1.,0.,0.));
#20172=DIRECTION('',(0.,0.,1.));
#20173=DIRECTION('center_axis',(0.,0.707106781186542,-0.707106781186553));
#20174=DIRECTION('ref_axis',(0.,0.707106781186553,0.707106781186542));
#20175=DIRECTION('',(0.,0.707106781186553,0.707106781186542));
#20176=DIRECTION('',(1.,0.,0.));
#20177=DIRECTION('',(0.,0.707106781186553,0.707106781186542));
#20178=DIRECTION('center_axis',(0.,0.,-1.));
#20179=DIRECTION('ref_axis',(-1.,0.,0.));
#20180=DIRECTION('',(0.,1.,0.));
#20181=DIRECTION('',(1.,0.,0.));
#20182=DIRECTION('',(0.,1.,0.));
#20183=DIRECTION('center_axis',(0.,-0.707106781186547,-0.707106781186548));
#20184=DIRECTION('ref_axis',(0.,0.707106781186548,-0.707106781186547));
#20185=DIRECTION('',(0.,0.707106781186548,-0.707106781186547));
#20186=DIRECTION('',(1.,0.,0.));
#20187=DIRECTION('',(0.,0.707106781186548,-0.707106781186547));
#20188=DIRECTION('center_axis',(0.,-1.,0.));
#20189=DIRECTION('ref_axis',(0.,0.,-1.));
#20190=DIRECTION('',(0.,0.,-1.));
#20191=DIRECTION('',(1.,0.,0.));
#20192=DIRECTION('',(0.,0.,-1.));
#20193=DIRECTION('center_axis',(0.,0.,1.));
#20194=DIRECTION('ref_axis',(1.,0.,0.));
#20195=DIRECTION('',(0.,-1.,0.));
#20196=DIRECTION('',(0.,-1.,0.));
#20197=DIRECTION('center_axis',(-1.,0.,0.));
#20198=DIRECTION('ref_axis',(0.,0.,1.));
#20199=DIRECTION('center_axis',(-1.,0.,0.));
#20200=DIRECTION('ref_axis',(0.,0.,1.));
#20201=DIRECTION('center_axis',(0.,0.886474799840877,0.462776867666349));
#20202=DIRECTION('ref_axis',(0.,-0.462776867666349,0.886474799840877));
#20203=DIRECTION('',(0.,-0.462776867666349,0.886474799840877));
#20204=DIRECTION('',(-1.,0.,0.));
#20205=DIRECTION('',(0.,-0.462776867666349,0.886474799840877));
#20206=DIRECTION('',(-1.,0.,0.));
#20207=DIRECTION('center_axis',(0.,1.,0.));
#20208=DIRECTION('ref_axis',(0.,0.,1.));
#20209=DIRECTION('',(0.,0.,1.));
#20210=DIRECTION('',(0.,0.,1.));
#20211=DIRECTION('',(-1.,0.,0.));
#20212=DIRECTION('center_axis',(0.,0.707106781186542,-0.707106781186553));
#20213=DIRECTION('ref_axis',(0.,0.707106781186553,0.707106781186542));
#20214=DIRECTION('',(0.,0.707106781186553,0.707106781186542));
#20215=DIRECTION('',(0.,0.707106781186553,0.707106781186542));
#20216=DIRECTION('',(-1.,0.,0.));
#20217=DIRECTION('center_axis',(0.,0.,-1.));
#20218=DIRECTION('ref_axis',(1.,0.,0.));
#20219=DIRECTION('',(0.,1.,0.));
#20220=DIRECTION('',(0.,1.,0.));
#20221=DIRECTION('',(-1.,0.,0.));
#20222=DIRECTION('center_axis',(0.,-0.707106781186547,-0.707106781186548));
#20223=DIRECTION('ref_axis',(0.,0.707106781186548,-0.707106781186547));
#20224=DIRECTION('',(0.,0.707106781186548,-0.707106781186547));
#20225=DIRECTION('',(0.,0.707106781186548,-0.707106781186547));
#20226=DIRECTION('',(-1.,0.,0.));
#20227=DIRECTION('center_axis',(0.,-1.,0.));
#20228=DIRECTION('ref_axis',(0.,0.,-1.));
#20229=DIRECTION('',(0.,0.,-1.));
#20230=DIRECTION('',(0.,0.,-1.));
#20231=DIRECTION('',(-1.,0.,0.));
#20232=DIRECTION('center_axis',(0.,0.,1.));
#20233=DIRECTION('ref_axis',(-1.,0.,0.));
#20234=DIRECTION('',(0.,-1.,0.));
#20235=DIRECTION('',(0.,-1.,0.));
#20236=DIRECTION('center_axis',(1.,0.,0.));
#20237=DIRECTION('ref_axis',(0.,0.,1.));
#20238=DIRECTION('center_axis',(1.,0.,0.));
#20239=DIRECTION('ref_axis',(0.,0.,1.));
#20240=DIRECTION('center_axis',(0.,0.886474799840877,0.462776867666349));
#20241=DIRECTION('ref_axis',(0.,-0.462776867666349,0.886474799840877));
#20242=DIRECTION('',(0.,-0.462776867666349,0.886474799840877));
#20243=DIRECTION('',(-1.,0.,0.));
#20244=DIRECTION('',(0.,-0.462776867666349,0.886474799840877));
#20245=DIRECTION('',(-1.,0.,0.));
#20246=DIRECTION('center_axis',(0.,1.,0.));
#20247=DIRECTION('ref_axis',(0.,0.,1.));
#20248=DIRECTION('',(0.,0.,1.));
#20249=DIRECTION('',(0.,0.,1.));
#20250=DIRECTION('',(-1.,0.,0.));
#20251=DIRECTION('center_axis',(0.,0.707106781186542,-0.707106781186553));
#20252=DIRECTION('ref_axis',(0.,0.707106781186553,0.707106781186542));
#20253=DIRECTION('',(0.,0.707106781186553,0.707106781186542));
#20254=DIRECTION('',(0.,0.707106781186553,0.707106781186542));
#20255=DIRECTION('',(-1.,0.,0.));
#20256=DIRECTION('center_axis',(0.,0.,-1.));
#20257=DIRECTION('ref_axis',(1.,0.,0.));
#20258=DIRECTION('',(0.,1.,0.));
#20259=DIRECTION('',(0.,1.,0.));
#20260=DIRECTION('',(-1.,0.,0.));
#20261=DIRECTION('center_axis',(0.,-0.707106781186547,-0.707106781186548));
#20262=DIRECTION('ref_axis',(0.,0.707106781186548,-0.707106781186547));
#20263=DIRECTION('',(0.,0.707106781186548,-0.707106781186547));
#20264=DIRECTION('',(0.,0.707106781186548,-0.707106781186547));
#20265=DIRECTION('',(-1.,0.,0.));
#20266=DIRECTION('center_axis',(0.,-1.,0.));
#20267=DIRECTION('ref_axis',(0.,0.,-1.));
#20268=DIRECTION('',(0.,0.,-1.));
#20269=DIRECTION('',(0.,0.,-1.));
#20270=DIRECTION('',(-1.,0.,0.));
#20271=DIRECTION('center_axis',(0.,0.,1.));
#20272=DIRECTION('ref_axis',(-1.,0.,0.));
#20273=DIRECTION('',(0.,-1.,0.));
#20274=DIRECTION('',(0.,-1.,0.));
#20275=DIRECTION('center_axis',(1.,0.,0.));
#20276=DIRECTION('ref_axis',(0.,0.,1.));
#20277=DIRECTION('center_axis',(1.,0.,0.));
#20278=DIRECTION('ref_axis',(0.,0.,1.));
#20279=DIRECTION('center_axis',(0.400352069216121,-0.916361402872453,0.));
#20280=DIRECTION('ref_axis',(-0.916361402872453,-0.400352069216121,0.));
#20281=DIRECTION('',(-0.916361402872453,-0.400352069216121,0.));
#20282=DIRECTION('',(0.,0.,1.));
#20283=DIRECTION('',(-0.916361402872453,-0.400352069216121,0.));
#20284=DIRECTION('',(0.,0.,1.));
#20285=DIRECTION('center_axis',(1.,0.,0.));
#20286=DIRECTION('ref_axis',(0.,0.,1.));
#20287=DIRECTION('',(0.,-1.,0.));
#20288=DIRECTION('',(0.,-1.,0.));
#20289=DIRECTION('',(0.,0.,1.));
#20290=DIRECTION('center_axis',(-1.92747052886312E-16,1.,0.));
#20291=DIRECTION('ref_axis',(1.,1.92747052886312E-16,0.));
#20292=DIRECTION('',(1.,1.92747052886312E-16,0.));
#20293=DIRECTION('',(1.,1.92747052886312E-16,0.));
#20294=DIRECTION('',(0.,0.,1.));
#20295=DIRECTION('center_axis',(-0.707106781186551,0.707106781186544,0.));
#20296=DIRECTION('ref_axis',(0.707106781186544,0.707106781186551,0.));
#20297=DIRECTION('',(0.707106781186544,0.707106781186551,0.));
#20298=DIRECTION('',(0.707106781186544,0.707106781186551,0.));
#20299=DIRECTION('',(0.,0.,1.));
#20300=DIRECTION('center_axis',(-1.,0.,0.));
#20301=DIRECTION('ref_axis',(0.,0.,-1.));
#20302=DIRECTION('',(0.,1.,0.));
#20303=DIRECTION('',(0.,1.,0.));
#20304=DIRECTION('',(0.,0.,1.));
#20305=DIRECTION('center_axis',(-0.707106781186546,-0.707106781186549,0.));
#20306=DIRECTION('ref_axis',(-0.707106781186549,0.707106781186546,0.));
#20307=DIRECTION('',(-0.707106781186549,0.707106781186546,0.));
#20308=DIRECTION('',(-0.707106781186549,0.707106781186546,0.));
#20309=DIRECTION('',(0.,0.,1.));
#20310=DIRECTION('center_axis',(-1.35393051783556E-15,-1.,0.));
#20311=DIRECTION('ref_axis',(-1.,1.35393051783556E-15,0.));
#20312=DIRECTION('',(-1.,1.35393051783556E-15,0.));
#20313=DIRECTION('',(-1.,1.35393051783556E-15,0.));
#20314=DIRECTION('center_axis',(0.,0.,1.));
#20315=DIRECTION('ref_axis',(-1.,0.,0.));
#20316=DIRECTION('center_axis',(0.,0.,1.));
#20317=DIRECTION('ref_axis',(-1.,0.,0.));
#20318=DIRECTION('center_axis',(0.400352069216121,-0.916361402872453,0.));
#20319=DIRECTION('ref_axis',(-0.916361402872453,-0.400352069216121,0.));
#20320=DIRECTION('',(-0.916361402872453,-0.400352069216121,0.));
#20321=DIRECTION('',(0.,0.,1.));
#20322=DIRECTION('',(-0.916361402872453,-0.400352069216121,0.));
#20323=DIRECTION('',(0.,0.,1.));
#20324=DIRECTION('center_axis',(1.,0.,0.));
#20325=DIRECTION('ref_axis',(0.,0.,1.));
#20326=DIRECTION('',(0.,-1.,0.));
#20327=DIRECTION('',(0.,-1.,0.));
#20328=DIRECTION('',(0.,0.,1.));
#20329=DIRECTION('center_axis',(-1.92747052886312E-16,1.,0.));
#20330=DIRECTION('ref_axis',(1.,1.92747052886312E-16,0.));
#20331=DIRECTION('',(1.,1.92747052886312E-16,0.));
#20332=DIRECTION('',(1.,1.92747052886312E-16,0.));
#20333=DIRECTION('',(0.,0.,1.));
#20334=DIRECTION('center_axis',(-0.707106781186551,0.707106781186544,0.));
#20335=DIRECTION('ref_axis',(0.707106781186544,0.707106781186551,0.));
#20336=DIRECTION('',(0.707106781186544,0.707106781186551,0.));
#20337=DIRECTION('',(0.707106781186544,0.707106781186551,0.));
#20338=DIRECTION('',(0.,0.,1.));
#20339=DIRECTION('center_axis',(-1.,0.,0.));
#20340=DIRECTION('ref_axis',(0.,0.,-1.));
#20341=DIRECTION('',(0.,1.,0.));
#20342=DIRECTION('',(0.,1.,0.));
#20343=DIRECTION('',(0.,0.,1.));
#20344=DIRECTION('center_axis',(-0.707106781186546,-0.707106781186549,0.));
#20345=DIRECTION('ref_axis',(-0.707106781186549,0.707106781186546,0.));
#20346=DIRECTION('',(-0.707106781186549,0.707106781186546,0.));
#20347=DIRECTION('',(-0.707106781186549,0.707106781186546,0.));
#20348=DIRECTION('',(0.,0.,1.));
#20349=DIRECTION('center_axis',(-1.35393051783556E-15,-1.,0.));
#20350=DIRECTION('ref_axis',(-1.,1.35393051783556E-15,0.));
#20351=DIRECTION('',(-1.,1.35393051783556E-15,0.));
#20352=DIRECTION('',(-1.,1.35393051783556E-15,0.));
#20353=DIRECTION('center_axis',(0.,0.,1.));
#20354=DIRECTION('ref_axis',(-1.,0.,0.));
#20355=DIRECTION('center_axis',(0.,0.,1.));
#20356=DIRECTION('ref_axis',(-1.,0.,0.));
#20357=DIRECTION('center_axis',(0.400352069216121,-0.916361402872453,0.));
#20358=DIRECTION('ref_axis',(-0.916361402872453,-0.400352069216121,0.));
#20359=DIRECTION('',(-0.916361402872453,-0.400352069216121,0.));
#20360=DIRECTION('',(0.,0.,1.));
#20361=DIRECTION('',(-0.916361402872453,-0.400352069216121,0.));
#20362=DIRECTION('',(0.,0.,1.));
#20363=DIRECTION('center_axis',(1.,0.,0.));
#20364=DIRECTION('ref_axis',(0.,0.,1.));
#20365=DIRECTION('',(0.,-1.,0.));
#20366=DIRECTION('',(0.,-1.,0.));
#20367=DIRECTION('',(0.,0.,1.));
#20368=DIRECTION('center_axis',(-1.92747052886312E-16,1.,0.));
#20369=DIRECTION('ref_axis',(1.,1.92747052886312E-16,0.));
#20370=DIRECTION('',(1.,1.92747052886312E-16,0.));
#20371=DIRECTION('',(1.,1.92747052886312E-16,0.));
#20372=DIRECTION('',(0.,0.,1.));
#20373=DIRECTION('center_axis',(-0.707106781186551,0.707106781186544,0.));
#20374=DIRECTION('ref_axis',(0.707106781186544,0.707106781186551,0.));
#20375=DIRECTION('',(0.707106781186544,0.707106781186551,0.));
#20376=DIRECTION('',(0.707106781186544,0.707106781186551,0.));
#20377=DIRECTION('',(0.,0.,1.));
#20378=DIRECTION('center_axis',(-1.,0.,0.));
#20379=DIRECTION('ref_axis',(0.,0.,-1.));
#20380=DIRECTION('',(0.,1.,0.));
#20381=DIRECTION('',(0.,1.,0.));
#20382=DIRECTION('',(0.,0.,1.));
#20383=DIRECTION('center_axis',(-0.707106781186546,-0.707106781186549,0.));
#20384=DIRECTION('ref_axis',(-0.707106781186549,0.707106781186546,0.));
#20385=DIRECTION('',(-0.707106781186549,0.707106781186546,0.));
#20386=DIRECTION('',(-0.707106781186549,0.707106781186546,0.));
#20387=DIRECTION('',(0.,0.,1.));
#20388=DIRECTION('center_axis',(-1.35393051783556E-15,-1.,0.));
#20389=DIRECTION('ref_axis',(-1.,1.35393051783556E-15,0.));
#20390=DIRECTION('',(-1.,1.35393051783556E-15,0.));
#20391=DIRECTION('',(-1.,1.35393051783556E-15,0.));
#20392=DIRECTION('center_axis',(0.,0.,1.));
#20393=DIRECTION('ref_axis',(-1.,0.,0.));
#20394=DIRECTION('center_axis',(0.,0.,1.));
#20395=DIRECTION('ref_axis',(-1.,0.,0.));
#20396=DIRECTION('center_axis',(0.,1.,0.));
#20397=DIRECTION('ref_axis',(0.,0.,1.));
#20398=DIRECTION('center_axis',(0.,1.,0.));
#20399=DIRECTION('ref_axis',(0.,0.,-1.));
#20400=DIRECTION('',(0.,1.,0.));
#20401=DIRECTION('center_axis',(0.,1.,0.));
#20402=DIRECTION('ref_axis',(0.,0.,-1.));
#20403=DIRECTION('center_axis',(0.,1.,0.));
#20404=DIRECTION('ref_axis',(0.,0.,1.));
#20405=DIRECTION('center_axis',(0.,1.,0.));
#20406=DIRECTION('ref_axis',(0.,0.,-1.));
#20407=DIRECTION('',(0.,1.,0.));
#20408=DIRECTION('center_axis',(0.,1.,0.));
#20409=DIRECTION('ref_axis',(0.,0.,-1.));
#20410=DIRECTION('center_axis',(0.,1.,0.));
#20411=DIRECTION('ref_axis',(0.,0.,1.));
#20412=DIRECTION('center_axis',(0.,1.,0.));
#20413=DIRECTION('ref_axis',(0.,0.,-1.));
#20414=DIRECTION('',(0.,1.,0.));
#20415=DIRECTION('center_axis',(0.,1.,0.));
#20416=DIRECTION('ref_axis',(0.,0.,-1.));
#20417=DIRECTION('center_axis',(0.,1.,0.));
#20418=DIRECTION('ref_axis',(0.,0.,1.));
#20419=DIRECTION('center_axis',(0.,1.,0.));
#20420=DIRECTION('ref_axis',(0.,0.,-1.));
#20421=DIRECTION('',(0.,1.,0.));
#20422=DIRECTION('center_axis',(0.,1.,0.));
#20423=DIRECTION('ref_axis',(0.,0.,-1.));
#20424=DIRECTION('center_axis',(0.,1.,0.));
#20425=DIRECTION('ref_axis',(0.,0.,1.));
#20426=DIRECTION('',(-2.36721327212187E-16,0.,-1.));
#20427=DIRECTION('',(1.,0.,-1.13752359080446E-16));
#20428=DIRECTION('',(2.36721327212187E-16,0.,1.));
#20429=DIRECTION('',(-1.,0.,-3.03339624214524E-16));
#20430=DIRECTION('center_axis',(0.,1.,0.));
#20431=DIRECTION('ref_axis',(0.,0.,1.));
#20432=DIRECTION('',(-2.36721327212187E-16,0.,-1.));
#20433=DIRECTION('',(-1.,0.,-3.03339624214524E-16));
#20434=DIRECTION('',(2.36721327212187E-16,0.,1.));
#20435=DIRECTION('',(1.,0.,-1.13752359080446E-16));
#20436=DIRECTION('center_axis',(-1.,0.,2.36721327212187E-16));
#20437=DIRECTION('ref_axis',(-2.36721327212187E-16,0.,-1.));
#20438=DIRECTION('',(0.,1.,0.));
#20439=DIRECTION('',(0.,1.,0.));
#20440=DIRECTION('center_axis',(-3.03339624214524E-16,0.,1.));
#20441=DIRECTION('ref_axis',(-1.,0.,-3.03339624214524E-16));
#20442=DIRECTION('',(0.,1.,0.));
#20443=DIRECTION('center_axis',(1.,0.,-2.36721327212187E-16));
#20444=DIRECTION('ref_axis',(2.36721327212187E-16,0.,1.));
#20445=DIRECTION('',(0.,1.,0.));
#20446=DIRECTION('center_axis',(-1.13752359080446E-16,0.,-1.));
#20447=DIRECTION('ref_axis',(1.,0.,-1.13752359080446E-16));
#20448=DIRECTION('center_axis',(1.,1.23267486838602E-16,-7.11670202791209E-17));
#20449=DIRECTION('ref_axis',(-1.23267486838602E-16,1.,6.0466247699241E-49));
#20450=DIRECTION('',(1.42336285208353E-16,-0.866029956157432,0.499992114975783));
#20451=DIRECTION('',(0.,-0.499992114975783,-0.866029956157432));
#20452=DIRECTION('',(1.42336285208353E-16,-0.866029956157432,0.499992114975783));
#20453=DIRECTION('',(0.,-0.499992114975783,-0.866029956157432));
#20454=DIRECTION('center_axis',(0.,0.866029956157432,-0.499992114975783));
#20455=DIRECTION('ref_axis',(0.,0.499992114975783,0.866029956157432));
#20456=DIRECTION('',(1.,0.,0.));
#20457=DIRECTION('',(0.,-0.499992114975783,-0.866029956157432));
#20458=DIRECTION('',(1.,0.,0.));
#20459=DIRECTION('center_axis',(-1.,0.,0.));
#20460=DIRECTION('ref_axis',(0.,0.,1.));
#20461=DIRECTION('',(0.,0.866029956157432,-0.499992114975783));
#20462=DIRECTION('',(0.,-0.499992114975783,-0.866029956157432));
#20463=DIRECTION('',(0.,0.866029956157432,-0.499992114975783));
#20464=DIRECTION('center_axis',(0.,-0.866029956157432,0.499992114975783));
#20465=DIRECTION('ref_axis',(0.,-0.499992114975783,-0.866029956157432));
#20466=DIRECTION('',(-1.,0.,0.));
#20467=DIRECTION('',(-1.,0.,0.));
#20468=DIRECTION('center_axis',(0.,0.499992114975783,0.866029956157432));
#20469=DIRECTION('ref_axis',(0.,-0.866029956157432,0.499992114975783));
#20470=DIRECTION('center_axis',(0.,0.499992114975783,0.866029956157432));
#20471=DIRECTION('ref_axis',(0.,-0.866029956157432,0.499992114975783));
#20472=DIRECTION('center_axis',(1.,-7.11113466337029E-16,4.10552918514724E-16));
#20473=DIRECTION('ref_axis',(7.1111346633703E-16,1.,8.60465311718737E-48));
#20474=DIRECTION('',(-8.21118786112474E-16,-0.866029956157432,0.499992114975783));
#20475=DIRECTION('',(0.,-0.499992114975783,-0.866029956157432));
#20476=DIRECTION('',(-8.21118786112474E-16,-0.866029956157432,0.499992114975783));
#20477=DIRECTION('',(0.,-0.499992114975783,-0.866029956157432));
#20478=DIRECTION('center_axis',(0.,0.866029956157432,-0.499992114975783));
#20479=DIRECTION('ref_axis',(0.,0.499992114975783,0.866029956157432));
#20480=DIRECTION('',(1.,0.,0.));
#20481=DIRECTION('',(0.,-0.499992114975783,-0.866029956157432));
#20482=DIRECTION('',(1.,0.,0.));
#20483=DIRECTION('center_axis',(-1.,0.,0.));
#20484=DIRECTION('ref_axis',(0.,0.,1.));
#20485=DIRECTION('',(0.,0.866029956157432,-0.499992114975783));
#20486=DIRECTION('',(0.,-0.499992114975783,-0.866029956157432));
#20487=DIRECTION('',(0.,0.866029956157432,-0.499992114975783));
#20488=DIRECTION('center_axis',(0.,-0.866029956157432,0.499992114975783));
#20489=DIRECTION('ref_axis',(0.,-0.499992114975783,-0.866029956157432));
#20490=DIRECTION('',(-1.,0.,0.));
#20491=DIRECTION('',(-1.,0.,0.));
#20492=DIRECTION('center_axis',(0.,0.499992114975783,0.866029956157432));
#20493=DIRECTION('ref_axis',(0.,-0.866029956157432,0.499992114975783));
#20494=DIRECTION('center_axis',(0.,0.499992114975783,0.866029956157432));
#20495=DIRECTION('ref_axis',(0.,-0.866029956157432,0.499992114975783));
#20496=DIRECTION('center_axis',(1.,0.,0.));
#20497=DIRECTION('ref_axis',(0.,0.,-1.));
#20498=DIRECTION('',(0.,-0.866029956157432,0.499992114975783));
#20499=DIRECTION('',(0.,-0.499992114975783,-0.866029956157432));
#20500=DIRECTION('',(0.,-0.866029956157432,0.499992114975783));
#20501=DIRECTION('',(0.,-0.499992114975783,-0.866029956157432));
#20502=DIRECTION('center_axis',(0.,0.866029956157432,-0.499992114975783));
#20503=DIRECTION('ref_axis',(0.,0.499992114975783,0.866029956157432));
#20504=DIRECTION('',(1.,0.,0.));
#20505=DIRECTION('',(0.,-0.499992114975783,-0.866029956157432));
#20506=DIRECTION('',(1.,0.,0.));
#20507=DIRECTION('center_axis',(-1.,0.,0.));
#20508=DIRECTION('ref_axis',(0.,0.,1.));
#20509=DIRECTION('',(0.,0.866029956157432,-0.499992114975783));
#20510=DIRECTION('',(0.,-0.499992114975783,-0.866029956157432));
#20511=DIRECTION('',(0.,0.866029956157432,-0.499992114975783));
#20512=DIRECTION('center_axis',(0.,-0.866029956157432,0.499992114975783));
#20513=DIRECTION('ref_axis',(0.,-0.499992114975783,-0.866029956157432));
#20514=DIRECTION('',(-1.,0.,0.));
#20515=DIRECTION('',(-1.,0.,0.));
#20516=DIRECTION('center_axis',(0.,0.499992114975783,0.866029956157432));
#20517=DIRECTION('ref_axis',(0.,-0.866029956157432,0.499992114975783));
#20518=DIRECTION('center_axis',(0.,0.499992114975783,0.866029956157432));
#20519=DIRECTION('ref_axis',(0.,-0.866029956157432,0.499992114975783));
#20520=DIRECTION('center_axis',(1.,0.,0.));
#20521=DIRECTION('ref_axis',(0.,0.,-1.));
#20522=DIRECTION('',(0.,-0.866029956157432,0.499992114975783));
#20523=DIRECTION('',(0.,-0.499992114975783,-0.866029956157432));
#20524=DIRECTION('',(0.,-0.866029956157432,0.499992114975783));
#20525=DIRECTION('',(0.,-0.499992114975783,-0.866029956157432));
#20526=DIRECTION('center_axis',(0.,0.866029956157432,-0.499992114975783));
#20527=DIRECTION('ref_axis',(0.,0.499992114975783,0.866029956157432));
#20528=DIRECTION('',(1.,0.,0.));
#20529=DIRECTION('',(0.,-0.499992114975783,-0.866029956157432));
#20530=DIRECTION('',(1.,0.,0.));
#20531=DIRECTION('center_axis',(-1.,0.,0.));
#20532=DIRECTION('ref_axis',(0.,0.,1.));
#20533=DIRECTION('',(0.,0.866029956157432,-0.499992114975783));
#20534=DIRECTION('',(0.,-0.499992114975783,-0.866029956157432));
#20535=DIRECTION('',(0.,0.866029956157432,-0.499992114975783));
#20536=DIRECTION('center_axis',(0.,-0.866029956157432,0.499992114975783));
#20537=DIRECTION('ref_axis',(0.,-0.499992114975783,-0.866029956157432));
#20538=DIRECTION('',(-1.,0.,0.));
#20539=DIRECTION('',(-1.,0.,0.));
#20540=DIRECTION('center_axis',(0.,0.499992114975783,0.866029956157432));
#20541=DIRECTION('ref_axis',(0.,-0.866029956157432,0.499992114975783));
#20542=DIRECTION('center_axis',(0.,0.499992114975783,0.866029956157432));
#20543=DIRECTION('ref_axis',(0.,-0.866029956157432,0.499992114975783));
#20544=DIRECTION('center_axis',(1.,0.,0.));
#20545=DIRECTION('ref_axis',(0.,0.,-1.));
#20546=DIRECTION('',(0.,-0.866029956157432,0.499992114975783));
#20547=DIRECTION('',(0.,-0.499992114975783,-0.866029956157432));
#20548=DIRECTION('',(0.,-0.866029956157432,0.499992114975783));
#20549=DIRECTION('',(0.,-0.499992114975783,-0.866029956157432));
#20550=DIRECTION('center_axis',(0.,0.866029956157432,-0.499992114975783));
#20551=DIRECTION('ref_axis',(0.,0.499992114975783,0.866029956157432));
#20552=DIRECTION('',(1.,0.,0.));
#20553=DIRECTION('',(0.,-0.499992114975783,-0.866029956157432));
#20554=DIRECTION('',(1.,0.,0.));
#20555=DIRECTION('center_axis',(-1.,0.,0.));
#20556=DIRECTION('ref_axis',(0.,0.,1.));
#20557=DIRECTION('',(0.,0.866029956157432,-0.499992114975783));
#20558=DIRECTION('',(0.,-0.499992114975783,-0.866029956157432));
#20559=DIRECTION('',(0.,0.866029956157432,-0.499992114975783));
#20560=DIRECTION('center_axis',(0.,-0.866029956157432,0.499992114975783));
#20561=DIRECTION('ref_axis',(0.,-0.499992114975783,-0.866029956157432));
#20562=DIRECTION('',(-1.,0.,0.));
#20563=DIRECTION('',(-1.,0.,0.));
#20564=DIRECTION('center_axis',(0.,0.499992114975783,0.866029956157432));
#20565=DIRECTION('ref_axis',(0.,-0.866029956157432,0.499992114975783));
#20566=DIRECTION('center_axis',(0.,0.499992114975783,0.866029956157432));
#20567=DIRECTION('ref_axis',(0.,-0.866029956157432,0.499992114975783));
#20568=DIRECTION('center_axis',(1.,-3.55556733168515E-16,2.05276459257362E-16));
#20569=DIRECTION('ref_axis',(3.55556733168515E-16,1.,2.15116327929684E-48));
#20570=DIRECTION('',(-4.10559393056237E-16,-0.866029956157432,0.499992114975783));
#20571=DIRECTION('',(0.,-0.499992114975783,-0.866029956157432));
#20572=DIRECTION('',(-4.10559393056237E-16,-0.866029956157432,0.499992114975783));
#20573=DIRECTION('',(0.,-0.499992114975783,-0.866029956157432));
#20574=DIRECTION('center_axis',(0.,0.866029956157432,-0.499992114975783));
#20575=DIRECTION('ref_axis',(0.,0.499992114975783,0.866029956157432));
#20576=DIRECTION('',(1.,0.,0.));
#20577=DIRECTION('',(0.,-0.499992114975783,-0.866029956157432));
#20578=DIRECTION('',(1.,0.,0.));
#20579=DIRECTION('center_axis',(-1.,7.16669040292788E-16,-4.1376036319062E-16));
#20580=DIRECTION('ref_axis',(-7.16669040292788E-16,-1.,2.01352657371916E-47));
#20581=DIRECTION('',(8.27533776628978E-16,0.866029956157432,-0.499992114975783));
#20582=DIRECTION('',(0.,-0.499992114975783,-0.866029956157432));
#20583=DIRECTION('',(8.27533776628978E-16,0.866029956157432,-0.499992114975783));
#20584=DIRECTION('center_axis',(0.,-0.866029956157432,0.499992114975783));
#20585=DIRECTION('ref_axis',(0.,-0.499992114975783,-0.866029956157432));
#20586=DIRECTION('',(-1.,0.,0.));
#20587=DIRECTION('',(-1.,0.,0.));
#20588=DIRECTION('center_axis',(0.,0.499992114975783,0.866029956157432));
#20589=DIRECTION('ref_axis',(0.,-0.866029956157432,0.499992114975783));
#20590=DIRECTION('center_axis',(0.,0.499992114975783,0.866029956157432));
#20591=DIRECTION('ref_axis',(0.,-0.866029956157432,0.499992114975783));
#20592=DIRECTION('center_axis',(1.67968331250372E-16,-0.866029956157432,
0.499992114975783));
#20593=DIRECTION('ref_axis',(-5.57351334278697E-33,-0.499992114975783,-0.866029956157432));
#20594=DIRECTION('',(-1.,-1.50505749146232E-16,7.52528745731158E-17));
#20595=DIRECTION('',(0.,-0.499992114975783,-0.866029956157432));
#20596=DIRECTION('',(-1.,-1.50505749146232E-16,7.52528745731158E-17));
#20597=DIRECTION('',(0.,-0.499992114975783,-0.866029956157432));
#20598=DIRECTION('center_axis',(0.866185586048601,0.432774614486462,-0.249857286421141));
#20599=DIRECTION('ref_axis',(-0.446950695480887,0.894558592719981,-6.35609056424636E-18));
#20600=DIRECTION('',(0.499722453489576,-0.750142665109869,0.433085963129978));
#20601=DIRECTION('',(0.,-0.499992114975783,-0.866029956157432));
#20602=DIRECTION('',(0.499722453489576,-0.750142665109869,0.433085963129978));
#20603=DIRECTION('center_axis',(0.,0.866029956157432,-0.499992114975783));
#20604=DIRECTION('ref_axis',(0.,0.499992114975783,0.866029956157432));
#20605=DIRECTION('',(1.,0.,0.));
#20606=DIRECTION('',(0.,-0.499992114975783,-0.866029956157432));
#20607=DIRECTION('',(1.,0.,0.));
#20608=DIRECTION('center_axis',(-0.866185586048601,0.432774614486462,-0.249857286421141));
#20609=DIRECTION('ref_axis',(-0.446950695480887,-0.89455859271998,8.76410190439018E-18));
#20610=DIRECTION('',(0.499722453489577,0.750142665109869,-0.433085963129978));
#20611=DIRECTION('',(0.499722453489577,0.750142665109869,-0.433085963129978));
#20612=DIRECTION('center_axis',(-1.00804441643628E-17,0.499992114975783,
0.866029956157432));
#20613=DIRECTION('ref_axis',(6.68767698777501E-35,-0.866029956157432,0.499992114975783));
#20614=DIRECTION('center_axis',(-1.00804441643628E-17,0.499992114975783,
0.866029956157432));
#20615=DIRECTION('ref_axis',(6.68767698777501E-35,-0.866029956157432,0.499992114975783));
#20616=DIRECTION('center_axis',(3.0024060161137E-16,0.499992114975783,0.866029956157432));
#20617=DIRECTION('ref_axis',(-1.13450604310479E-33,-0.866029956157432,0.499992114975783));
#20618=DIRECTION('',(-0.499722453489577,-0.750142665109869,0.433085963129978));
#20619=DIRECTION('',(0.866185586048601,-0.432774614486463,0.249857286421141));
#20620=DIRECTION('',(-0.499722453489577,-0.750142665109869,0.433085963129978));
#20621=DIRECTION('',(0.866185586048601,-0.432774614486463,0.249857286421141));
#20622=DIRECTION('center_axis',(0.499722453489577,0.750142665109869,-0.433085963129978));
#20623=DIRECTION('ref_axis',(-0.832241064261676,0.554413934670291,-3.58035061299401E-18));
#20624=DIRECTION('',(0.,0.499992114975783,0.866029956157432));
#20625=DIRECTION('',(0.866185586048601,-0.432774614486463,0.249857286421141));
#20626=DIRECTION('',(0.,0.499992114975783,0.866029956157432));
#20627=DIRECTION('center_axis',(0.,-0.499992114975783,-0.866029956157432));
#20628=DIRECTION('ref_axis',(0.,0.866029956157432,-0.499992114975783));
#20629=DIRECTION('',(0.499722453489577,0.750142665109869,-0.433085963129978));
#20630=DIRECTION('',(0.866185586048601,-0.432774614486463,0.249857286421141));
#20631=DIRECTION('',(0.499722453489577,0.750142665109869,-0.433085963129978));
#20632=DIRECTION('center_axis',(-0.499722453489577,-0.750142665109869,0.433085963129978));
#20633=DIRECTION('ref_axis',(0.832241064261676,-0.554413934670291,3.58035061299401E-18));
#20634=DIRECTION('',(0.,-0.499992114975783,-0.866029956157432));
#20635=DIRECTION('',(0.,-0.499992114975783,-0.866029956157432));
#20636=DIRECTION('center_axis',(-0.866185586048601,0.432774614486463,-0.249857286421141));
#20637=DIRECTION('ref_axis',(-0.446950695480888,-0.89455859271998,1.05171903626344E-18));
#20638=DIRECTION('center_axis',(-0.866185586048601,0.432774614486463,-0.249857286421141));
#20639=DIRECTION('ref_axis',(-0.446950695480888,-0.89455859271998,1.05171903626344E-18));
#20640=DIRECTION('center_axis',(3.0024060161137E-16,0.499992114975783,0.866029956157432));
#20641=DIRECTION('ref_axis',(-1.13450604310479E-33,-0.866029956157432,0.499992114975783));
#20642=DIRECTION('',(-0.499722453489577,-0.750142665109869,0.433085963129978));
#20643=DIRECTION('',(0.866185586048601,-0.432774614486463,0.249857286421141));
#20644=DIRECTION('',(-0.499722453489577,-0.750142665109869,0.433085963129978));
#20645=DIRECTION('',(0.866185586048601,-0.432774614486463,0.249857286421141));
#20646=DIRECTION('center_axis',(0.499722453489577,0.750142665109869,-0.433085963129978));
#20647=DIRECTION('ref_axis',(-0.832241064261676,0.554413934670291,-3.58035061299401E-18));
#20648=DIRECTION('',(0.,0.499992114975783,0.866029956157432));
#20649=DIRECTION('',(0.866185586048601,-0.432774614486463,0.249857286421141));
#20650=DIRECTION('',(0.,0.499992114975783,0.866029956157432));
#20651=DIRECTION('center_axis',(0.,-0.499992114975783,-0.866029956157432));
#20652=DIRECTION('ref_axis',(0.,0.866029956157432,-0.499992114975783));
#20653=DIRECTION('',(0.499722453489577,0.750142665109869,-0.433085963129978));
#20654=DIRECTION('',(0.866185586048601,-0.432774614486463,0.249857286421141));
#20655=DIRECTION('',(0.499722453489577,0.750142665109869,-0.433085963129978));
#20656=DIRECTION('center_axis',(-0.499722453489577,-0.750142665109869,0.433085963129978));
#20657=DIRECTION('ref_axis',(0.832241064261676,-0.554413934670291,3.58035061299401E-18));
#20658=DIRECTION('',(0.,-0.499992114975783,-0.866029956157432));
#20659=DIRECTION('',(0.,-0.499992114975783,-0.866029956157432));
#20660=DIRECTION('center_axis',(-0.866185586048601,0.432774614486463,-0.249857286421141));
#20661=DIRECTION('ref_axis',(-0.446950695480888,-0.89455859271998,1.05171903626344E-18));
#20662=DIRECTION('center_axis',(-0.866185586048601,0.432774614486463,-0.249857286421141));
#20663=DIRECTION('ref_axis',(-0.446950695480888,-0.89455859271998,1.05171903626344E-18));
#20664=DIRECTION('center_axis',(3.0024060161137E-16,0.499992114975783,0.866029956157432));
#20665=DIRECTION('ref_axis',(-1.13450604310479E-33,-0.866029956157432,0.499992114975783));
#20666=DIRECTION('',(-0.499722453489577,-0.750142665109869,0.433085963129978));
#20667=DIRECTION('',(0.866185586048601,-0.432774614486463,0.249857286421141));
#20668=DIRECTION('',(-0.499722453489577,-0.750142665109869,0.433085963129978));
#20669=DIRECTION('',(0.866185586048601,-0.432774614486463,0.249857286421141));
#20670=DIRECTION('center_axis',(0.499722453489577,0.750142665109869,-0.433085963129978));
#20671=DIRECTION('ref_axis',(-0.832241064261676,0.554413934670291,-3.58035061299401E-18));
#20672=DIRECTION('',(0.,0.499992114975783,0.866029956157432));
#20673=DIRECTION('',(0.866185586048601,-0.432774614486463,0.249857286421141));
#20674=DIRECTION('',(0.,0.499992114975783,0.866029956157432));
#20675=DIRECTION('center_axis',(0.,-0.499992114975783,-0.866029956157432));
#20676=DIRECTION('ref_axis',(0.,0.866029956157432,-0.499992114975783));
#20677=DIRECTION('',(0.499722453489577,0.750142665109869,-0.433085963129978));
#20678=DIRECTION('',(0.866185586048601,-0.432774614486463,0.249857286421141));
#20679=DIRECTION('',(0.499722453489577,0.750142665109869,-0.433085963129978));
#20680=DIRECTION('center_axis',(-0.499722453489577,-0.750142665109869,0.433085963129978));
#20681=DIRECTION('ref_axis',(0.832241064261676,-0.554413934670291,3.58035061299401E-18));
#20682=DIRECTION('',(0.,-0.499992114975783,-0.866029956157432));
#20683=DIRECTION('',(0.,-0.499992114975783,-0.866029956157432));
#20684=DIRECTION('center_axis',(-0.866185586048601,0.432774614486463,-0.249857286421141));
#20685=DIRECTION('ref_axis',(-0.446950695480888,-0.89455859271998,1.05171903626344E-18));
#20686=DIRECTION('center_axis',(-0.866185586048601,0.432774614486463,-0.249857286421141));
#20687=DIRECTION('ref_axis',(-0.446950695480888,-0.89455859271998,1.05171903626344E-18));
#20688=DIRECTION('center_axis',(3.0024060161137E-16,0.499992114975783,0.866029956157432));
#20689=DIRECTION('ref_axis',(-1.13450604310479E-33,-0.866029956157432,0.499992114975783));
#20690=DIRECTION('',(-0.499722453489577,-0.750142665109869,0.433085963129978));
#20691=DIRECTION('',(0.866185586048601,-0.432774614486463,0.249857286421141));
#20692=DIRECTION('',(-0.499722453489577,-0.750142665109869,0.433085963129978));
#20693=DIRECTION('',(0.866185586048601,-0.432774614486463,0.249857286421141));
#20694=DIRECTION('center_axis',(0.499722453489577,0.750142665109869,-0.433085963129978));
#20695=DIRECTION('ref_axis',(-0.832241064261676,0.554413934670291,-3.58035061299401E-18));
#20696=DIRECTION('',(0.,0.499992114975783,0.866029956157432));
#20697=DIRECTION('',(0.866185586048601,-0.432774614486463,0.249857286421141));
#20698=DIRECTION('',(0.,0.499992114975783,0.866029956157432));
#20699=DIRECTION('center_axis',(0.,-0.499992114975783,-0.866029956157432));
#20700=DIRECTION('ref_axis',(0.,0.866029956157432,-0.499992114975783));
#20701=DIRECTION('',(0.499722453489577,0.750142665109869,-0.433085963129978));
#20702=DIRECTION('',(0.866185586048601,-0.432774614486463,0.249857286421141));
#20703=DIRECTION('',(0.499722453489577,0.750142665109869,-0.433085963129978));
#20704=DIRECTION('center_axis',(-0.499722453489577,-0.750142665109869,0.433085963129978));
#20705=DIRECTION('ref_axis',(0.832241064261676,-0.554413934670291,3.58035061299401E-18));
#20706=DIRECTION('',(0.,-0.499992114975783,-0.866029956157432));
#20707=DIRECTION('',(0.,-0.499992114975783,-0.866029956157432));
#20708=DIRECTION('center_axis',(-0.866185586048601,0.432774614486463,-0.249857286421141));
#20709=DIRECTION('ref_axis',(-0.446950695480888,-0.89455859271998,1.05171903626344E-18));
#20710=DIRECTION('center_axis',(-0.866185586048601,0.432774614486463,-0.249857286421141));
#20711=DIRECTION('ref_axis',(-0.446950695480888,-0.89455859271998,1.05171903626344E-18));
#20712=DIRECTION('center_axis',(-3.0024060161137E-16,0.499992114975783,
0.866029956157432));
#20713=DIRECTION('ref_axis',(1.13450604310479E-33,-0.866029956157432,0.499992114975783));
#20714=DIRECTION('',(0.499722453489577,-0.750142665109869,0.433085963129978));
#20715=DIRECTION('',(-0.866185586048601,-0.432774614486463,0.249857286421141));
#20716=DIRECTION('',(0.499722453489577,-0.750142665109869,0.433085963129978));
#20717=DIRECTION('',(-0.866185586048601,-0.432774614486463,0.249857286421141));
#20718=DIRECTION('center_axis',(-0.499722453489577,0.750142665109869,-0.433085963129978));
#20719=DIRECTION('ref_axis',(0.832241064261676,0.554413934670291,-3.58035061299401E-18));
#20720=DIRECTION('',(0.,0.499992114975783,0.866029956157432));
#20721=DIRECTION('',(0.,0.499992114975783,0.866029956157432));
#20722=DIRECTION('',(-0.866185586048601,-0.432774614486463,0.249857286421141));
#20723=DIRECTION('center_axis',(0.,-0.499992114975783,-0.866029956157432));
#20724=DIRECTION('ref_axis',(0.,0.866029956157432,-0.499992114975783));
#20725=DIRECTION('',(-0.499722453489577,0.750142665109869,-0.433085963129978));
#20726=DIRECTION('',(-0.499722453489577,0.750142665109869,-0.433085963129978));
#20727=DIRECTION('',(-0.866185586048601,-0.432774614486463,0.249857286421141));
#20728=DIRECTION('center_axis',(0.499722453489577,-0.750142665109869,0.433085963129978));
#20729=DIRECTION('ref_axis',(-0.832241064261676,-0.554413934670291,3.58035061299401E-18));
#20730=DIRECTION('',(0.,-0.499992114975783,-0.866029956157432));
#20731=DIRECTION('',(0.,-0.499992114975783,-0.866029956157432));
#20732=DIRECTION('center_axis',(0.866185586048601,0.432774614486463,-0.249857286421141));
#20733=DIRECTION('ref_axis',(0.446950695480888,-0.89455859271998,1.05171903626344E-18));
#20734=DIRECTION('center_axis',(0.866185586048601,0.432774614486463,-0.249857286421141));
#20735=DIRECTION('ref_axis',(0.446950695480888,-0.89455859271998,1.05171903626344E-18));
#20736=DIRECTION('center_axis',(-3.0024060161137E-16,0.499992114975783,
0.866029956157432));
#20737=DIRECTION('ref_axis',(1.13450604310479E-33,-0.866029956157432,0.499992114975783));
#20738=DIRECTION('',(0.499722453489577,-0.750142665109869,0.433085963129978));
#20739=DIRECTION('',(-0.866185586048601,-0.432774614486463,0.249857286421141));
#20740=DIRECTION('',(0.499722453489577,-0.750142665109869,0.433085963129978));
#20741=DIRECTION('',(-0.866185586048601,-0.432774614486463,0.249857286421141));
#20742=DIRECTION('center_axis',(-0.499722453489577,0.750142665109869,-0.433085963129978));
#20743=DIRECTION('ref_axis',(0.832241064261676,0.554413934670291,-3.58035061299401E-18));
#20744=DIRECTION('',(0.,0.499992114975783,0.866029956157432));
#20745=DIRECTION('',(0.,0.499992114975783,0.866029956157432));
#20746=DIRECTION('',(-0.866185586048601,-0.432774614486463,0.249857286421141));
#20747=DIRECTION('center_axis',(0.,-0.499992114975783,-0.866029956157432));
#20748=DIRECTION('ref_axis',(0.,0.866029956157432,-0.499992114975783));
#20749=DIRECTION('',(-0.499722453489577,0.750142665109869,-0.433085963129978));
#20750=DIRECTION('',(-0.499722453489577,0.750142665109869,-0.433085963129978));
#20751=DIRECTION('',(-0.866185586048601,-0.432774614486463,0.249857286421141));
#20752=DIRECTION('center_axis',(0.499722453489577,-0.750142665109869,0.433085963129978));
#20753=DIRECTION('ref_axis',(-0.832241064261676,-0.554413934670291,3.58035061299401E-18));
#20754=DIRECTION('',(0.,-0.499992114975783,-0.866029956157432));
#20755=DIRECTION('',(0.,-0.499992114975783,-0.866029956157432));
#20756=DIRECTION('center_axis',(0.866185586048601,0.432774614486463,-0.249857286421141));
#20757=DIRECTION('ref_axis',(0.446950695480888,-0.89455859271998,1.05171903626344E-18));
#20758=DIRECTION('center_axis',(0.866185586048601,0.432774614486463,-0.249857286421141));
#20759=DIRECTION('ref_axis',(0.446950695480888,-0.89455859271998,1.05171903626344E-18));
#20760=DIRECTION('center_axis',(-3.0024060161137E-16,0.499992114975783,
0.866029956157432));
#20761=DIRECTION('ref_axis',(1.13450604310479E-33,-0.866029956157432,0.499992114975783));
#20762=DIRECTION('',(0.499722453489577,-0.750142665109869,0.433085963129978));
#20763=DIRECTION('',(-0.866185586048601,-0.432774614486463,0.249857286421141));
#20764=DIRECTION('',(0.499722453489577,-0.750142665109869,0.433085963129978));
#20765=DIRECTION('',(-0.866185586048601,-0.432774614486463,0.249857286421141));
#20766=DIRECTION('center_axis',(-0.499722453489577,0.750142665109869,-0.433085963129978));
#20767=DIRECTION('ref_axis',(0.832241064261676,0.554413934670291,-3.58035061299401E-18));
#20768=DIRECTION('',(0.,0.499992114975783,0.866029956157432));
#20769=DIRECTION('',(0.,0.499992114975783,0.866029956157432));
#20770=DIRECTION('',(-0.866185586048601,-0.432774614486463,0.249857286421141));
#20771=DIRECTION('center_axis',(0.,-0.499992114975783,-0.866029956157432));
#20772=DIRECTION('ref_axis',(0.,0.866029956157432,-0.499992114975783));
#20773=DIRECTION('',(-0.499722453489577,0.750142665109869,-0.433085963129978));
#20774=DIRECTION('',(-0.499722453489577,0.750142665109869,-0.433085963129978));
#20775=DIRECTION('',(-0.866185586048601,-0.432774614486463,0.249857286421141));
#20776=DIRECTION('center_axis',(0.499722453489577,-0.750142665109869,0.433085963129978));
#20777=DIRECTION('ref_axis',(-0.832241064261676,-0.554413934670291,3.58035061299401E-18));
#20778=DIRECTION('',(0.,-0.499992114975783,-0.866029956157432));
#20779=DIRECTION('',(0.,-0.499992114975783,-0.866029956157432));
#20780=DIRECTION('center_axis',(0.866185586048601,0.432774614486463,-0.249857286421141));
#20781=DIRECTION('ref_axis',(0.446950695480888,-0.89455859271998,1.05171903626344E-18));
#20782=DIRECTION('center_axis',(0.866185586048601,0.432774614486463,-0.249857286421141));
#20783=DIRECTION('ref_axis',(0.446950695480888,-0.89455859271998,1.05171903626344E-18));
#20784=DIRECTION('center_axis',(-3.0024060161137E-16,0.499992114975783,
0.866029956157432));
#20785=DIRECTION('ref_axis',(1.13450604310479E-33,-0.866029956157432,0.499992114975783));
#20786=DIRECTION('',(0.499722453489577,-0.750142665109869,0.433085963129978));
#20787=DIRECTION('',(-0.866185586048601,-0.432774614486463,0.249857286421141));
#20788=DIRECTION('',(0.499722453489577,-0.750142665109869,0.433085963129978));
#20789=DIRECTION('',(-0.866185586048601,-0.432774614486463,0.249857286421141));
#20790=DIRECTION('center_axis',(-0.499722453489577,0.750142665109869,-0.433085963129978));
#20791=DIRECTION('ref_axis',(0.832241064261676,0.554413934670291,-3.58035061299401E-18));
#20792=DIRECTION('',(0.,0.499992114975783,0.866029956157432));
#20793=DIRECTION('',(0.,0.499992114975783,0.866029956157432));
#20794=DIRECTION('',(-0.866185586048601,-0.432774614486463,0.249857286421141));
#20795=DIRECTION('center_axis',(0.,-0.499992114975783,-0.866029956157432));
#20796=DIRECTION('ref_axis',(0.,0.866029956157432,-0.499992114975783));
#20797=DIRECTION('',(-0.499722453489577,0.750142665109869,-0.433085963129978));
#20798=DIRECTION('',(-0.499722453489577,0.750142665109869,-0.433085963129978));
#20799=DIRECTION('',(-0.866185586048601,-0.432774614486463,0.249857286421141));
#20800=DIRECTION('center_axis',(0.499722453489577,-0.750142665109869,0.433085963129978));
#20801=DIRECTION('ref_axis',(-0.832241064261676,-0.554413934670291,3.58035061299401E-18));
#20802=DIRECTION('',(0.,-0.499992114975783,-0.866029956157432));
#20803=DIRECTION('',(0.,-0.499992114975783,-0.866029956157432));
#20804=DIRECTION('center_axis',(0.866185586048601,0.432774614486463,-0.249857286421141));
#20805=DIRECTION('ref_axis',(0.446950695480888,-0.89455859271998,1.05171903626344E-18));
#20806=DIRECTION('center_axis',(0.866185586048601,0.432774614486463,-0.249857286421141));
#20807=DIRECTION('ref_axis',(0.446950695480888,-0.89455859271998,1.05171903626344E-18));
#20808=DIRECTION('center_axis',(7.72189864380049E-11,-0.866021775524098,
0.500006284278597));
#20809=DIRECTION('ref_axis',(9.43920741915831E-6,0.500006284256323,0.866021775485517));
#20810=DIRECTION('',(-0.999999999955451,4.71959615486962E-6,8.17459777866693E-6));
#20811=DIRECTION('',(9.43920741915831E-6,0.500006284256323,0.866021775485517));
#20812=DIRECTION('',(-0.999999999955451,4.71959615486962E-6,8.17459777866693E-6));
#20813=DIRECTION('',(9.43920741915831E-6,0.500006284256323,0.866021775485517));
#20814=DIRECTION('center_axis',(0.866185585971425,0.43276643839414,-0.249871447858675));
#20815=DIRECTION('ref_axis',(-0.44695491741627,0.447282837726406,-0.774705986082997));
#20816=DIRECTION('',(0.4997224535342,-0.75013793765136,0.433094151345782));
#20817=DIRECTION('',(0.4997224535342,-0.75013793765136,0.433094151345782));
#20818=DIRECTION('',(9.43920741915831E-6,0.500006284256323,0.866021775485517));
#20819=DIRECTION('center_axis',(-7.72188184696774E-11,0.866021775524098,
-0.500006284278597));
#20820=DIRECTION('ref_axis',(-9.43920741915831E-6,-0.500006284256323,-0.866021775485517));
#20821=DIRECTION('',(0.999999999955451,-4.71959615501004E-6,-8.17459777857421E-6));
#20822=DIRECTION('',(0.999999999955451,-4.71959615501004E-6,-8.17459777857421E-6));
#20823=DIRECTION('',(9.43920741915831E-6,0.500006284256323,0.866021775485517));
#20824=DIRECTION('center_axis',(-0.866185586048601,0.432774614486463,-0.24985728642114));
#20825=DIRECTION('ref_axis',(-0.446946473505681,-0.447278618872838,0.774713293367322));
#20826=DIRECTION('',(0.499722453400429,0.75013322067502,-0.433102321405899));
#20827=DIRECTION('',(0.499722453400429,0.75013322067502,-0.433102321405899));
#20828=DIRECTION('center_axis',(-9.43920741916839E-6,-0.500006284256323,
-0.866021775485517));
#20829=DIRECTION('ref_axis',(7.72188184718094E-11,-0.866021775524098,0.500006284278598));
#20830=DIRECTION('center_axis',(-9.43920741916839E-6,-0.500006284256323,
-0.866021775485517));
#20831=DIRECTION('ref_axis',(7.72188184718094E-11,-0.866021775524098,0.500006284278598));
#20832=DIRECTION('center_axis',(-1.,1.68317620470764E-16,0.));
#20833=DIRECTION('ref_axis',(-1.68317620470764E-16,-1.,0.));
#20834=DIRECTION('',(-1.68317620470764E-16,-1.,0.));
#20835=DIRECTION('',(0.,0.,1.));
#20836=DIRECTION('',(-1.68317620470764E-16,-1.,0.));
#20837=DIRECTION('',(0.,0.,1.));
#20838=DIRECTION('center_axis',(0.,1.,0.));
#20839=DIRECTION('ref_axis',(0.,0.,1.));
#20840=DIRECTION('',(-1.,0.,0.));
#20841=DIRECTION('',(0.,0.,1.));
#20842=DIRECTION('',(-1.,0.,0.));
#20843=DIRECTION('center_axis',(1.,0.,0.));
#20844=DIRECTION('ref_axis',(0.,0.,-1.));
#20845=DIRECTION('',(0.,1.,0.));
#20846=DIRECTION('',(0.,0.,1.));
#20847=DIRECTION('',(0.,1.,0.));
#20848=DIRECTION('center_axis',(0.,-1.,0.));
#20849=DIRECTION('ref_axis',(0.,0.,-1.));
#20850=DIRECTION('',(1.,0.,0.));
#20851=DIRECTION('',(1.,0.,0.));
#20852=DIRECTION('center_axis',(0.,0.,-1.));
#20853=DIRECTION('ref_axis',(-1.,0.,0.));
#20854=DIRECTION('center_axis',(0.,0.,-1.));
#20855=DIRECTION('ref_axis',(-1.,0.,0.));
#20856=DIRECTION('center_axis',(-1.,1.68317620470764E-16,0.));
#20857=DIRECTION('ref_axis',(-1.68317620470764E-16,-1.,0.));
#20858=DIRECTION('',(-1.68317620470764E-16,-1.,0.));
#20859=DIRECTION('',(0.,0.,1.));
#20860=DIRECTION('',(-1.68317620470764E-16,-1.,0.));
#20861=DIRECTION('',(0.,0.,1.));
#20862=DIRECTION('center_axis',(0.,1.,0.));
#20863=DIRECTION('ref_axis',(0.,0.,1.));
#20864=DIRECTION('',(-1.,0.,0.));
#20865=DIRECTION('',(0.,0.,1.));
#20866=DIRECTION('',(-1.,0.,0.));
#20867=DIRECTION('center_axis',(1.,-1.68317620470764E-16,0.));
#20868=DIRECTION('ref_axis',(1.68317620470764E-16,1.,0.));
#20869=DIRECTION('',(1.68317620470764E-16,1.,0.));
#20870=DIRECTION('',(0.,0.,1.));
#20871=DIRECTION('',(1.68317620470764E-16,1.,0.));
#20872=DIRECTION('center_axis',(0.,-1.,0.));
#20873=DIRECTION('ref_axis',(0.,0.,-1.));
#20874=DIRECTION('',(1.,0.,0.));
#20875=DIRECTION('',(1.,0.,0.));
#20876=DIRECTION('center_axis',(0.,0.,-1.));
#20877=DIRECTION('ref_axis',(-1.,0.,0.));
#20878=DIRECTION('center_axis',(0.,0.,-1.));
#20879=DIRECTION('ref_axis',(-1.,0.,0.));
#20880=DIRECTION('center_axis',(-1.,0.,0.));
#20881=DIRECTION('ref_axis',(0.,0.,1.));
#20882=DIRECTION('',(0.,-1.,0.));
#20883=DIRECTION('',(0.,0.,1.));
#20884=DIRECTION('',(0.,-1.,0.));
#20885=DIRECTION('',(0.,0.,1.));
#20886=DIRECTION('center_axis',(0.,1.,0.));
#20887=DIRECTION('ref_axis',(0.,0.,1.));
#20888=DIRECTION('',(-1.,0.,0.));
#20889=DIRECTION('',(0.,0.,1.));
#20890=DIRECTION('',(-1.,0.,0.));
#20891=DIRECTION('center_axis',(1.,0.,0.));
#20892=DIRECTION('ref_axis',(0.,0.,-1.));
#20893=DIRECTION('',(0.,1.,0.));
#20894=DIRECTION('',(0.,0.,1.));
#20895=DIRECTION('',(0.,1.,0.));
#20896=DIRECTION('center_axis',(0.,-1.,0.));
#20897=DIRECTION('ref_axis',(0.,0.,-1.));
#20898=DIRECTION('',(1.,0.,0.));
#20899=DIRECTION('',(1.,0.,0.));
#20900=DIRECTION('center_axis',(0.,0.,1.));
#20901=DIRECTION('ref_axis',(1.,0.,0.));
#20902=DIRECTION('center_axis',(0.,0.,1.));
#20903=DIRECTION('ref_axis',(1.,0.,0.));
#20904=DIRECTION('center_axis',(-1.,0.,0.));
#20905=DIRECTION('ref_axis',(0.,0.,1.));
#20906=DIRECTION('',(0.,-1.,0.));
#20907=DIRECTION('',(0.,0.,1.));
#20908=DIRECTION('',(0.,-1.,0.));
#20909=DIRECTION('',(0.,0.,1.));
#20910=DIRECTION('center_axis',(0.,1.,0.));
#20911=DIRECTION('ref_axis',(0.,0.,1.));
#20912=DIRECTION('',(-1.,0.,0.));
#20913=DIRECTION('',(0.,0.,1.));
#20914=DIRECTION('',(-1.,0.,0.));
#20915=DIRECTION('center_axis',(1.,0.,0.));
#20916=DIRECTION('ref_axis',(0.,0.,-1.));
#20917=DIRECTION('',(0.,1.,0.));
#20918=DIRECTION('',(0.,0.,1.));
#20919=DIRECTION('',(0.,1.,0.));
#20920=DIRECTION('center_axis',(0.,-1.,0.));
#20921=DIRECTION('ref_axis',(0.,0.,-1.));
#20922=DIRECTION('',(1.,0.,0.));
#20923=DIRECTION('',(1.,0.,0.));
#20924=DIRECTION('center_axis',(0.,0.,1.));
#20925=DIRECTION('ref_axis',(1.,0.,0.));
#20926=DIRECTION('center_axis',(0.,0.,1.));
#20927=DIRECTION('ref_axis',(1.,0.,0.));
#20928=DIRECTION('center_axis',(-1.,3.73454720419507E-16,0.));
#20929=DIRECTION('ref_axis',(-3.73454720419507E-16,-1.,0.));
#20930=DIRECTION('',(-3.73454720419507E-16,-1.,0.));
#20931=DIRECTION('',(0.,0.,1.));
#20932=DIRECTION('',(-3.73454720419507E-16,-1.,0.));
#20933=DIRECTION('',(0.,0.,1.));
#20934=DIRECTION('center_axis',(0.,1.,0.));
#20935=DIRECTION('ref_axis',(0.,0.,1.));
#20936=DIRECTION('',(-1.,0.,0.));
#20937=DIRECTION('',(0.,0.,1.));
#20938=DIRECTION('',(-1.,0.,0.));
#20939=DIRECTION('center_axis',(1.,-3.36635240941527E-16,0.));
#20940=DIRECTION('ref_axis',(3.36635240941527E-16,1.,0.));
#20941=DIRECTION('',(3.36635240941527E-16,1.,0.));
#20942=DIRECTION('',(0.,0.,1.));
#20943=DIRECTION('',(3.36635240941527E-16,1.,0.));
#20944=DIRECTION('center_axis',(0.,-1.,0.));
#20945=DIRECTION('ref_axis',(0.,0.,-1.));
#20946=DIRECTION('',(1.,0.,0.));
#20947=DIRECTION('',(1.,0.,0.));
#20948=DIRECTION('center_axis',(0.,0.,-1.));
#20949=DIRECTION('ref_axis',(-1.,0.,0.));
#20950=DIRECTION('center_axis',(0.,0.,-1.));
#20951=DIRECTION('ref_axis',(-1.,0.,0.));
#20952=DIRECTION('center_axis',(-1.,6.73270481883054E-16,0.));
#20953=DIRECTION('ref_axis',(-6.73270481883054E-16,-1.,0.));
#20954=DIRECTION('',(-6.73270481883054E-16,-1.,0.));
#20955=DIRECTION('',(0.,0.,1.));
#20956=DIRECTION('',(-6.73270481883054E-16,-1.,0.));
#20957=DIRECTION('',(0.,0.,1.));
#20958=DIRECTION('center_axis',(0.,1.,0.));
#20959=DIRECTION('ref_axis',(0.,0.,1.));
#20960=DIRECTION('',(-1.,0.,0.));
#20961=DIRECTION('',(0.,0.,1.));
#20962=DIRECTION('',(-1.,0.,0.));
#20963=DIRECTION('center_axis',(1.,-6.73270481883054E-16,0.));
#20964=DIRECTION('ref_axis',(6.73270481883054E-16,1.,0.));
#20965=DIRECTION('',(6.73270481883054E-16,1.,0.));
#20966=DIRECTION('',(0.,0.,1.));
#20967=DIRECTION('',(6.73270481883054E-16,1.,0.));
#20968=DIRECTION('center_axis',(0.,-1.,0.));
#20969=DIRECTION('ref_axis',(0.,0.,-1.));
#20970=DIRECTION('',(1.,0.,0.));
#20971=DIRECTION('',(1.,0.,0.));
#20972=DIRECTION('center_axis',(0.,0.,-1.));
#20973=DIRECTION('ref_axis',(-1.,0.,0.));
#20974=DIRECTION('center_axis',(0.,0.,-1.));
#20975=DIRECTION('ref_axis',(-1.,0.,0.));
#30705=CARTESIAN_POINT('',(0.,0.,0.));
#30706=CARTESIAN_POINT('Origin',(400.,-277.5,15.875));
#30707=CARTESIAN_POINT('',(400.,-277.5,0.));
#30708=CARTESIAN_POINT('',(400.,277.5,0.));
#30709=CARTESIAN_POINT('',(400.,-277.5,0.));
#30710=CARTESIAN_POINT('',(400.,277.5,15.875));
#30711=CARTESIAN_POINT('',(400.,277.5,15.875));
#30712=CARTESIAN_POINT('',(400.,-277.5,15.875));
#30713=CARTESIAN_POINT('',(400.,-277.5,15.875));
#30714=CARTESIAN_POINT('',(400.,-277.5,15.875));
#30715=CARTESIAN_POINT('Origin',(-400.,277.5,15.875));
#30716=CARTESIAN_POINT('',(-400.,277.5,0.));
#30717=CARTESIAN_POINT('',(-400.,277.5,0.));
#30718=CARTESIAN_POINT('',(-400.,277.5,15.875));
#30719=CARTESIAN_POINT('',(-400.,277.5,15.875));
#30720=CARTESIAN_POINT('',(-400.,277.5,15.875));
#30721=CARTESIAN_POINT('Origin',(-400.,-277.5,15.875));
#30722=CARTESIAN_POINT('',(-400.,-277.5,0.));
#30723=CARTESIAN_POINT('',(-400.,-277.5,0.));
#30724=CARTESIAN_POINT('',(-400.,-277.5,15.875));
#30725=CARTESIAN_POINT('',(-400.,-277.5,15.875));
#30726=CARTESIAN_POINT('',(-400.,-277.5,15.875));
#30727=CARTESIAN_POINT('Origin',(-400.,-277.5,15.875));
#30728=CARTESIAN_POINT('',(-400.,-277.5,0.));
#30729=CARTESIAN_POINT('',(-400.,-277.5,15.875));
#30730=CARTESIAN_POINT('Origin',(0.,0.,15.875));
#30731=CARTESIAN_POINT('Origin',(0.,0.,0.));
#30732=CARTESIAN_POINT('Origin',(412.7,-0.499999999999945,-407.52));
#30733=CARTESIAN_POINT('',(412.7,-0.49999999999995,-447.52));
#30734=CARTESIAN_POINT('Origin',(412.7,-0.499999999999945,-407.52));
#30735=CARTESIAN_POINT('',(400.,-0.49999999999995,-447.52));
#30736=CARTESIAN_POINT('',(412.7,-0.49999999999995,-447.52));
#30737=CARTESIAN_POINT('Origin',(400.,-0.499999999999945,-407.52));
#30738=CARTESIAN_POINT('Origin',(412.7,277.5,-647.52));
#30739=CARTESIAN_POINT('',(412.7,277.5,0.));
#30740=CARTESIAN_POINT('',(412.7,-282.5,0.));
#30741=CARTESIAN_POINT('',(412.7,-282.5,0.));
#30742=CARTESIAN_POINT('',(412.7,-532.5,-433.));
#30743=CARTESIAN_POINT('',(412.7,-532.5,-433.));
#30744=CARTESIAN_POINT('',(412.7,23.5000000000001,-754.));
#30745=CARTESIAN_POINT('',(412.7,23.5000000000001,-754.));
#30746=CARTESIAN_POINT('',(412.7,230.764157791864,-588.861999240546));
#30747=CARTESIAN_POINT('',(412.7,230.764157791864,-588.861999240546));
#30748=CARTESIAN_POINT('',(412.7,277.5,-572.52));
#30749=CARTESIAN_POINT('Origin',(412.7,277.5,-647.52));
#30750=CARTESIAN_POINT('',(412.7,277.5,0.));
#30751=CARTESIAN_POINT('Origin',(400.,277.5,-647.52));
#30752=CARTESIAN_POINT('',(400.,277.5,0.));
#30753=CARTESIAN_POINT('',(400.,-282.5,0.));
#30754=CARTESIAN_POINT('',(400.,-282.5,0.));
#30755=CARTESIAN_POINT('',(400.,277.5,-572.52));
#30756=CARTESIAN_POINT('',(400.,277.5,0.));
#30757=CARTESIAN_POINT('',(400.,230.764157791864,-588.861999240546));
#30758=CARTESIAN_POINT('Origin',(400.,277.5,-647.52));
#30759=CARTESIAN_POINT('',(400.,23.5000000000001,-754.));
#30760=CARTESIAN_POINT('',(400.,230.764157791864,-588.861999240546));
#30761=CARTESIAN_POINT('',(400.,-532.5,-433.));
#30762=CARTESIAN_POINT('',(400.,23.5000000000001,-754.));
#30763=CARTESIAN_POINT('',(400.,-532.5,-433.));
#30764=CARTESIAN_POINT('Origin',(412.7,-282.5,0.));
#30765=CARTESIAN_POINT('',(412.7,-282.5,0.));
#30766=CARTESIAN_POINT('',(412.7,277.5,0.));
#30767=CARTESIAN_POINT('Origin',(412.7,-532.5,-433.));
#30768=CARTESIAN_POINT('',(412.7,-532.5,-433.));
#30769=CARTESIAN_POINT('Origin',(412.7,23.5000000000001,-754.));
#30770=CARTESIAN_POINT('',(412.7,23.5000000000001,-754.));
#30771=CARTESIAN_POINT('Origin',(412.7,230.764157791864,-588.861999240546));
#30772=CARTESIAN_POINT('',(412.7,230.764157791864,-588.861999240546));
#30773=CARTESIAN_POINT('Origin',(412.7,277.5,-647.52));
#30774=CARTESIAN_POINT('',(412.7,277.5,-572.52));
#30775=CARTESIAN_POINT('Origin',(412.7,277.5,0.));
#30776=CARTESIAN_POINT('Origin',(-412.7,-0.499999999999945,-407.52));
#30777=CARTESIAN_POINT('',(-412.7,-0.49999999999994,-447.52));
#30778=CARTESIAN_POINT('Origin',(-412.7,-0.499999999999945,-407.52));
#30779=CARTESIAN_POINT('',(-400.,-0.49999999999994,-447.52));
#30780=CARTESIAN_POINT('',(-412.7,-0.49999999999994,-447.52));
#30781=CARTESIAN_POINT('Origin',(-400.,-0.499999999999945,-407.52));
#30782=CARTESIAN_POINT('Origin',(-412.7,277.5,-647.52));
#30783=CARTESIAN_POINT('',(-412.7,277.5,0.));
#30784=CARTESIAN_POINT('',(-412.7,-282.5,0.));
#30785=CARTESIAN_POINT('',(-412.7,-282.5,0.));
#30786=CARTESIAN_POINT('',(-412.7,277.5,-572.52));
#30787=CARTESIAN_POINT('',(-412.7,277.5,0.));
#30788=CARTESIAN_POINT('',(-412.7,230.764157791864,-588.861999240546));
#30789=CARTESIAN_POINT('Origin',(-412.7,277.5,-647.52));
#30790=CARTESIAN_POINT('',(-412.7,23.5000000000001,-754.));
#30791=CARTESIAN_POINT('',(-412.7,230.764157791864,-588.861999240546));
#30792=CARTESIAN_POINT('',(-412.7,-532.5,-433.));
#30793=CARTESIAN_POINT('',(-412.7,23.5000000000001,-754.));
#30794=CARTESIAN_POINT('',(-412.7,-532.5,-433.));
#30795=CARTESIAN_POINT('Origin',(-400.,277.5,-647.52));
#30796=CARTESIAN_POINT('',(-400.,277.5,0.));
#30797=CARTESIAN_POINT('',(-400.,-282.5,0.));
#30798=CARTESIAN_POINT('',(-400.,-282.5,0.));
#30799=CARTESIAN_POINT('',(-400.,-532.5,-433.));
#30800=CARTESIAN_POINT('',(-400.,-532.5,-433.));
#30801=CARTESIAN_POINT('',(-400.,23.5000000000001,-754.));
#30802=CARTESIAN_POINT('',(-400.,23.5000000000001,-754.));
#30803=CARTESIAN_POINT('',(-400.,230.764157791864,-588.861999240546));
#30804=CARTESIAN_POINT('',(-400.,230.764157791864,-588.861999240546));
#30805=CARTESIAN_POINT('',(-400.,277.5,-572.52));
#30806=CARTESIAN_POINT('Origin',(-400.,277.5,-647.52));
#30807=CARTESIAN_POINT('',(-400.,277.5,0.));
#30808=CARTESIAN_POINT('Origin',(-412.7,-282.5,0.));
#30809=CARTESIAN_POINT('',(-412.7,277.5,0.));
#30810=CARTESIAN_POINT('',(-412.7,-282.5,0.));
#30811=CARTESIAN_POINT('Origin',(-412.7,-532.5,-433.));
#30812=CARTESIAN_POINT('',(-412.7,-532.5,-433.));
#30813=CARTESIAN_POINT('Origin',(-412.7,23.5000000000001,-754.));
#30814=CARTESIAN_POINT('',(-412.7,23.5000000000001,-754.));
#30815=CARTESIAN_POINT('Origin',(-412.7,230.764157791864,-588.861999240546));
#30816=CARTESIAN_POINT('',(-412.7,230.764157791864,-588.861999240546));
#30817=CARTESIAN_POINT('Origin',(-412.7,277.5,-647.52));
#30818=CARTESIAN_POINT('',(-412.7,277.5,-572.52));
#30819=CARTESIAN_POINT('Origin',(-412.7,277.5,0.));
#30820=CARTESIAN_POINT('Origin',(300.,-4.50064876413007,-752.498777568804));
#30821=CARTESIAN_POINT('',(300.,3.2936208412868,-756.998706603586));
#30822=CARTESIAN_POINT('Origin',(300.,-4.50064876413007,-752.498777568804));
#30823=CARTESIAN_POINT('',(300.,9.64352070147921,-746.000126160387));
#30824=CARTESIAN_POINT('',(300.,3.2936208412868,-756.998706603586));
#30825=CARTESIAN_POINT('Origin',(300.,1.84925109606238,-741.500197125605));
#30826=CARTESIAN_POINT('Origin',(150.,-4.50064876412913,-752.498777568804));
#30827=CARTESIAN_POINT('',(150.,3.29362084128775,-756.998706603587));
#30828=CARTESIAN_POINT('Origin',(150.,-4.50064876412913,-752.498777568804));
#30829=CARTESIAN_POINT('',(150.,9.64352070148016,-746.000126160387));
#30830=CARTESIAN_POINT('',(150.,3.29362084128775,-756.998706603587));
#30831=CARTESIAN_POINT('Origin',(150.,1.84925109606332,-741.500197125605));
#30832=CARTESIAN_POINT('Origin',(-300.,-4.50064876412824,-752.498777568805));
#30833=CARTESIAN_POINT('',(-300.,3.29362084128862,-756.998706603587));
#30834=CARTESIAN_POINT('Origin',(-300.,-4.50064876412824,-752.498777568805));
#30835=CARTESIAN_POINT('',(-300.,9.64352070148111,-746.000126160388));
#30836=CARTESIAN_POINT('',(-300.,3.29362084128863,-756.998706603587));
#30837=CARTESIAN_POINT('Origin',(-300.,1.84925109606421,-741.500197125606));
#30838=CARTESIAN_POINT('Origin',(-150.,-4.50064876412824,-752.498777568805));
#30839=CARTESIAN_POINT('',(-150.,3.29362084128864,-756.998706603587));
#30840=CARTESIAN_POINT('Origin',(-150.,-4.50064876412824,-752.498777568805));
#30841=CARTESIAN_POINT('',(-150.,9.64352070148113,-746.000126160388));
#30842=CARTESIAN_POINT('',(-150.,3.29362084128864,-756.998706603587));
#30843=CARTESIAN_POINT('Origin',(-150.,1.84925109606421,-741.500197125606));
#30844=CARTESIAN_POINT('Origin',(0.,-4.50064876412824,-752.498777568805));
#30845=CARTESIAN_POINT('',(-1.10218211923262E-15,3.29362084128864,-756.998706603587));
#30846=CARTESIAN_POINT('Origin',(0.,-4.50064876412824,-752.498777568805));
#30847=CARTESIAN_POINT('',(-1.10218211923262E-15,9.64352070148112,-746.000126160388));
#30848=CARTESIAN_POINT('',(-1.10218211923262E-15,3.29362084128864,-756.998706603587));
#30849=CARTESIAN_POINT('Origin',(0.,1.84925109606421,-741.500197125606));
#30850=CARTESIAN_POINT('Origin',(0.,-326.963229813101,-566.328834193409));
#30851=CARTESIAN_POINT('',(400.,17.1501001398076,-764.9985804432));
#30852=CARTESIAN_POINT('',(400.,-538.849899860193,-443.9985804432));
#30853=CARTESIAN_POINT('',(400.,-538.849899860193,-443.9985804432));
#30854=CARTESIAN_POINT('',(250.,-764.017688461125,-314.000630549496));
#30855=CARTESIAN_POINT('',(250.,-764.017688461125,-314.000630549496));
#30856=CARTESIAN_POINT('',(250.,-805.587126356682,-290.001009030658));
#30857=CARTESIAN_POINT('',(250.,-805.587126356682,-290.001009030658));
#30858=CARTESIAN_POINT('',(-250.,-805.587126356682,-290.001009030658));
#30859=CARTESIAN_POINT('',(-250.,-805.587126356682,-290.001009030658));
#30860=CARTESIAN_POINT('',(-250.,-764.017688461125,-314.000630549496));
#30861=CARTESIAN_POINT('',(-250.,-764.017688461125,-314.000630549496));
#30862=CARTESIAN_POINT('',(-400.,-538.849899860193,-443.9985804432));
#30863=CARTESIAN_POINT('',(-400.,-538.849899860193,-443.9985804432));
#30864=CARTESIAN_POINT('',(-400.,17.1501001398076,-764.9985804432));
#30865=CARTESIAN_POINT('',(-400.,17.1501001398076,-764.9985804432));
#30866=CARTESIAN_POINT('',(400.,17.1501001398076,-764.9985804432));
#30867=CARTESIAN_POINT('Origin',(0.,-320.613329952909,-555.33025375021));
#30868=CARTESIAN_POINT('',(400.,23.5,-754.));
#30869=CARTESIAN_POINT('',(400.,-532.5,-433.));
#30870=CARTESIAN_POINT('',(400.,-532.5,-433.));
#30871=CARTESIAN_POINT('',(-400.,23.5,-754.));
#30872=CARTESIAN_POINT('',(400.,23.5,-754.));
#30873=CARTESIAN_POINT('',(-400.,-532.5,-433.));
#30874=CARTESIAN_POINT('',(-400.,23.5,-754.));
#30875=CARTESIAN_POINT('',(-250.,-757.667788600933,-303.002050106297));
#30876=CARTESIAN_POINT('',(-400.,-532.5,-433.));
#30877=CARTESIAN_POINT('',(-250.,-799.237226496489,-279.002428587459));
#30878=CARTESIAN_POINT('',(-250.,-757.667788600933,-303.002050106297));
#30879=CARTESIAN_POINT('',(250.,-799.237226496489,-279.002428587459));
#30880=CARTESIAN_POINT('',(-250.,-799.237226496489,-279.002428587459));
#30881=CARTESIAN_POINT('',(250.,-757.667788600933,-303.002050106297));
#30882=CARTESIAN_POINT('',(250.,-799.237226496489,-279.002428587459));
#30883=CARTESIAN_POINT('',(250.,-757.667788600933,-303.002050106297));
#30884=CARTESIAN_POINT('Origin',(400.,-538.849899860193,-443.9985804432));
#30885=CARTESIAN_POINT('',(400.,-538.849899860193,-443.9985804432));
#30886=CARTESIAN_POINT('',(400.,17.1501001398076,-764.9985804432));
#30887=CARTESIAN_POINT('Origin',(250.,-764.017688461125,-314.000630549496));
#30888=CARTESIAN_POINT('',(250.,-764.017688461125,-314.000630549496));
#30889=CARTESIAN_POINT('Origin',(250.,-805.587126356682,-290.001009030658));
#30890=CARTESIAN_POINT('',(250.,-805.587126356682,-290.001009030658));
#30891=CARTESIAN_POINT('Origin',(-250.,-805.587126356682,-290.001009030658));
#30892=CARTESIAN_POINT('',(-250.,-805.587126356682,-290.001009030658));
#30893=CARTESIAN_POINT('Origin',(-250.,-764.017688461125,-314.000630549496));
#30894=CARTESIAN_POINT('',(-250.,-764.017688461125,-314.000630549496));
#30895=CARTESIAN_POINT('Origin',(-400.,-538.849899860193,-443.9985804432));
#30896=CARTESIAN_POINT('',(-400.,-538.849899860193,-443.9985804432));
#30897=CARTESIAN_POINT('Origin',(-400.,17.1501001398076,-764.9985804432));
#30898=CARTESIAN_POINT('',(-400.,17.1501001398076,-764.9985804432));
#30899=CARTESIAN_POINT('Origin',(400.,17.1501001398076,-764.9985804432));
#30900=CARTESIAN_POINT('Origin',(411.000556942817,-537.996237603978,-429.826812462452));
#30901=CARTESIAN_POINT('',(251.582431340073,-755.289566540481,-304.368610542448));
#30902=CARTESIAN_POINT('',(400.,-532.5,-433.));
#30903=CARTESIAN_POINT('',(400.,-532.5,-433.));
#30904=CARTESIAN_POINT('',(411.000556942817,-537.996237603978,-429.826812462452));
#30905=CARTESIAN_POINT('',(411.000556942817,-537.996237603978,-429.826812462452));
#30906=CARTESIAN_POINT('',(262.58298828289,-760.785804144459,-301.195423004899));
#30907=CARTESIAN_POINT('',(411.000556942817,-537.996237603978,-429.826812462452));
#30908=CARTESIAN_POINT('',(262.58298828289,-760.785804144459,-301.195423004899));
#30909=CARTESIAN_POINT('Origin',(411.000556942817,-537.996237603978,-429.826812462452));
#30910=CARTESIAN_POINT('',(400.004719499877,-282.502358016311,0.00136137272609138));
#30911=CARTESIAN_POINT('',(400.,-532.5,-433.));
#30912=CARTESIAN_POINT('',(411.005276442694,-287.998595620289,3.17454891027458));
#30913=CARTESIAN_POINT('',(411.005276442694,-287.998595620289,3.17454891027458));
#30914=CARTESIAN_POINT('',(411.000556942817,-537.996237603978,-429.826812462452));
#30915=CARTESIAN_POINT('Origin',(411.005276442694,-287.998595620289,3.17454891027458));
#30916=CARTESIAN_POINT('',(251.58715083995,-505.291924556791,128.632750830278));
#30917=CARTESIAN_POINT('',(400.004719499877,-282.502358016311,0.00136137272609138));
#30918=CARTESIAN_POINT('',(262.587707782767,-510.788162160769,131.805938367827));
#30919=CARTESIAN_POINT('',(262.587707782767,-510.788162160769,131.805938367827));
#30920=CARTESIAN_POINT('',(411.005276442694,-287.998595620289,3.17454891027458));
#30921=CARTESIAN_POINT('Origin',(262.58298828289,-760.785804144459,-301.195423004899));
#30922=CARTESIAN_POINT('',(251.582431340073,-755.289566540481,-304.368610542448));
#30923=CARTESIAN_POINT('',(262.58298828289,-760.785804144459,-301.195423004899));
#30924=CARTESIAN_POINT('Origin',(417.015099327983,-208.354366262308,120.290920090289));
#30925=CARTESIAN_POINT('Origin',(406.014542385166,-202.85812865833,117.117732552741));
#30926=CARTESIAN_POINT('Origin',(262.7,-799.237226496489,-279.002428587459));
#30927=CARTESIAN_POINT('',(250.,-799.237226496489,-279.002428587459));
#30928=CARTESIAN_POINT('',(250.,-760.266369128196,-301.502923603794));
#30929=CARTESIAN_POINT('',(250.,-799.237226496489,-279.002428587459));
#30930=CARTESIAN_POINT('',(262.7,-760.266369128196,-301.502923603794));
#30931=CARTESIAN_POINT('',(262.7,-760.266369128196,-301.502923603794));
#30932=CARTESIAN_POINT('',(262.7,-799.237226496489,-279.002428587459));
#30933=CARTESIAN_POINT('',(262.7,-799.237226496489,-279.002428587459));
#30934=CARTESIAN_POINT('',(262.7,-799.237226496489,-279.002428587459));
#30935=CARTESIAN_POINT('Origin',(262.7,-760.266369128196,-301.502923603794));
#30936=CARTESIAN_POINT('',(250.,-510.263080007906,131.502773152548));
#30937=CARTESIAN_POINT('',(250.,-760.266369128196,-301.502923603794));
#30938=CARTESIAN_POINT('',(262.7,-510.263080007906,131.502773152548));
#30939=CARTESIAN_POINT('',(262.7,-510.263080007906,131.502773152548));
#30940=CARTESIAN_POINT('',(262.7,-760.266369128196,-301.502923603794));
#30941=CARTESIAN_POINT('Origin',(262.7,-549.2339373762,154.003268168884));
#30942=CARTESIAN_POINT('',(250.,-549.2339373762,154.003268168884));
#30943=CARTESIAN_POINT('',(250.,-549.2339373762,154.003268168884));
#30944=CARTESIAN_POINT('',(262.7,-549.2339373762,154.003268168884));
#30945=CARTESIAN_POINT('',(262.7,-549.2339373762,154.003268168884));
#30946=CARTESIAN_POINT('',(262.7,-549.2339373762,154.003268168884));
#30947=CARTESIAN_POINT('Origin',(262.7,-799.237226496489,-279.002428587459));
#30948=CARTESIAN_POINT('',(250.,-799.237226496489,-279.002428587459));
#30949=CARTESIAN_POINT('',(262.7,-799.237226496489,-279.002428587459));
#30950=CARTESIAN_POINT('Origin',(262.7,0.,0.));
#30951=CARTESIAN_POINT('Origin',(250.,0.,0.));
#30952=CARTESIAN_POINT('Origin',(249.998786597631,-501.314873870463,141.001336655876));
#30953=CARTESIAN_POINT('',(249.998666719697,-507.664953680518,130.00286010721));
#30954=CARTESIAN_POINT('',(400.,-282.5,-1.38777878078145E-14));
#30955=CARTESIAN_POINT('',(249.998666719697,-507.664953680518,130.00286010721));
#30956=CARTESIAN_POINT('',(400.000119877934,-276.149920189945,10.998476548666));
#30957=CARTESIAN_POINT('',(400.000119877934,-276.149920189945,10.998476548666));
#30958=CARTESIAN_POINT('',(249.998786597631,-501.314873870463,141.001336655876));
#30959=CARTESIAN_POINT('',(249.998786597631,-501.314873870463,141.001336655876));
#30960=CARTESIAN_POINT('',(249.998786597631,-501.314873870463,141.001336655876));
#30961=CARTESIAN_POINT('Origin',(400.000119877934,-276.149920189945,10.998476548666));
#30962=CARTESIAN_POINT('',(-399.999999928721,-282.496224269578,0.00653964733464407));
#30963=CARTESIAN_POINT('',(400.,-282.5,-1.38777878078145E-14));
#30964=CARTESIAN_POINT('',(-399.999880050787,-276.146144459522,11.0050161960007));
#30965=CARTESIAN_POINT('',(-399.999880050787,-276.146144459522,11.0050161960007));
#30966=CARTESIAN_POINT('',(400.000119877934,-276.149920189945,10.998476548666));
#30967=CARTESIAN_POINT('Origin',(-399.999880050787,-276.146144459522,11.0050161960007));
#30968=CARTESIAN_POINT('',(-250.001333258029,-507.662593849004,130.006947386795));
#30969=CARTESIAN_POINT('',(-399.999999928721,-282.496224269578,0.00653964733464407));
#30970=CARTESIAN_POINT('',(-250.001213380094,-501.312514038949,141.005423935461));
#30971=CARTESIAN_POINT('',(-250.001213380094,-501.312514038949,141.005423935461));
#30972=CARTESIAN_POINT('',(-399.999880050787,-276.146144459522,11.0050161960007));
#30973=CARTESIAN_POINT('Origin',(-250.001213380094,-501.312514038949,141.005423935461));
#30974=CARTESIAN_POINT('',(-250.001333258029,-549.231639074161,154.007249032168));
#30975=CARTESIAN_POINT('',(-250.001333258029,-507.662593849004,130.006947386795));
#30976=CARTESIAN_POINT('',(-250.001213380094,-542.881559264105,165.005725580834));
#30977=CARTESIAN_POINT('',(-250.001213380094,-542.881559264105,165.005725580834));
#30978=CARTESIAN_POINT('',(-250.001213380094,-501.312514038949,141.005423935461));
#30979=CARTESIAN_POINT('Origin',(-250.001213380094,-542.881559264105,165.005725580834));
#30980=CARTESIAN_POINT('',(249.998666719697,-549.233998905675,154.003161752583));
#30981=CARTESIAN_POINT('',(-250.001333258029,-549.231639074161,154.007249032168));
#30982=CARTESIAN_POINT('',(249.998786597631,-542.883919095619,165.001638301249));
#30983=CARTESIAN_POINT('',(249.998786597631,-542.883919095619,165.001638301249));
#30984=CARTESIAN_POINT('',(-250.001213380094,-542.881559264105,165.005725580834));
#30985=CARTESIAN_POINT('Origin',(249.998786597631,-542.883919095619,165.001638301249));
#30986=CARTESIAN_POINT('',(249.998666719697,-549.233998905675,154.003161752583));
#30987=CARTESIAN_POINT('',(249.998786597631,-542.883919095619,165.001638301249));
#30988=CARTESIAN_POINT('Origin',(-0.00121339123172574,-64.2748076383018,
-111.325366865542));
#30989=CARTESIAN_POINT('Origin',(-0.00133326916594913,-70.6248874483571,
-122.323843414208));
#30990=CARTESIAN_POINT('Origin',(296.200000000004,-734.583240701635,-141.622283996917));
#30991=CARTESIAN_POINT('',(296.200000000004,-739.083339704902,-149.416455470576));
#30992=CARTESIAN_POINT('Origin',(296.200000000004,-734.583240701635,-141.622283996917));
#30993=CARTESIAN_POINT('',(296.200000000004,-728.084897736517,-155.766595175186));
#30994=CARTESIAN_POINT('',(296.200000000004,-739.083339704902,-149.416455470576));
#30995=CARTESIAN_POINT('Origin',(296.200000000004,-723.58479873325,-147.972423701528));
#30996=CARTESIAN_POINT('Origin',(296.200000000002,-635.581062629759,29.8494884235731));
#30997=CARTESIAN_POINT('',(296.200000000002,-640.081161633026,22.0553169499145));
#30998=CARTESIAN_POINT('Origin',(296.200000000002,-635.581062629759,29.8494884235731));
#30999=CARTESIAN_POINT('',(296.200000000002,-629.082719664641,15.7051772453043));
#31000=CARTESIAN_POINT('',(296.200000000002,-640.081161633026,22.0553169499145));
#31001=CARTESIAN_POINT('Origin',(296.200000000002,-624.582620661374,23.4993487189629));
#31002=CARTESIAN_POINT('Origin',(296.2,-536.578884557882,201.321260844064));
#31003=CARTESIAN_POINT('',(296.2,-541.078983561149,193.527089370405));
#31004=CARTESIAN_POINT('Origin',(296.2,-536.578884557882,201.321260844064));
#31005=CARTESIAN_POINT('',(296.2,-530.080541592764,187.176949665795));
#31006=CARTESIAN_POINT('',(296.2,-541.078983561149,193.527089370405));
#31007=CARTESIAN_POINT('Origin',(296.2,-525.580442589497,194.971121139453));
#31008=CARTESIAN_POINT('Origin',(0.,-489.60420247788,282.681410206628));
#31009=CARTESIAN_POINT('',(262.7,-521.578554546992,227.301832422926));
#31010=CARTESIAN_POINT('',(262.7,-816.585044761169,-283.649408628031));
#31011=CARTESIAN_POINT('',(262.7,-521.578554546992,227.301832422926));
#31012=CARTESIAN_POINT('',(326.2,-816.585044761169,-283.649408628031));
#31013=CARTESIAN_POINT('',(262.7,-816.585044761169,-283.649408628031));
#31014=CARTESIAN_POINT('',(326.2,-521.578554546992,227.301832422926));
#31015=CARTESIAN_POINT('',(326.2,-521.578554546992,227.301832422926));
#31016=CARTESIAN_POINT('',(262.7,-521.578554546992,227.301832422926));
#31017=CARTESIAN_POINT('Origin',(0.,-478.605760509495,276.331270502017));
#31018=CARTESIAN_POINT('',(262.7,-510.580112578607,220.951692718316));
#31019=CARTESIAN_POINT('',(262.7,-805.586602792784,-289.999548332641));
#31020=CARTESIAN_POINT('',(262.7,-510.580112578607,220.951692718316));
#31021=CARTESIAN_POINT('',(326.2,-510.580112578607,220.951692718316));
#31022=CARTESIAN_POINT('',(262.7,-510.580112578607,220.951692718316));
#31023=CARTESIAN_POINT('',(326.2,-805.586602792784,-289.999548332641));
#31024=CARTESIAN_POINT('',(326.2,-510.580112578607,220.951692718316));
#31025=CARTESIAN_POINT('',(262.7,-805.586602792784,-289.999548332641));
#31026=CARTESIAN_POINT('Origin',(262.7,-521.578554546992,227.301832422926));
#31027=CARTESIAN_POINT('',(262.7,-816.585044761169,-283.649408628031));
#31028=CARTESIAN_POINT('',(262.7,-521.578554546992,227.301832422926));
#31029=CARTESIAN_POINT('Origin',(262.7,-816.585044761169,-283.649408628031));
#31030=CARTESIAN_POINT('',(326.2,-816.585044761169,-283.649408628031));
#31031=CARTESIAN_POINT('Origin',(326.2,-521.578554546992,227.301832422926));
#31032=CARTESIAN_POINT('',(326.2,-521.578554546992,227.301832422926));
#31033=CARTESIAN_POINT('Origin',(262.7,-521.578554546992,227.301832422926));
#31034=CARTESIAN_POINT('Origin',(98.6978247534365,-537.131180039572,200.368985977147));
#31035=CARTESIAN_POINT('',(107.697824753303,-537.131222484398,200.36901048309));
#31036=CARTESIAN_POINT('Origin',(98.6978247534365,-537.131180039572,200.368985977147));
#31037=CARTESIAN_POINT('',(107.69789391365,-526.132745935405,194.018930672846));
#31038=CARTESIAN_POINT('',(107.697824753303,-537.131222484398,200.36901048309));
#31039=CARTESIAN_POINT('Origin',(98.6978939137833,-526.132703490579,194.018906166903));
#31040=CARTESIAN_POINT('Origin',(-99.3021752436275,-537.130246253392,200.368446846407));
#31041=CARTESIAN_POINT('',(-90.302175243761,-537.130288698218,200.368471352349));
#31042=CARTESIAN_POINT('Origin',(-99.3021752436275,-537.130246253392,200.368446846407));
#31043=CARTESIAN_POINT('',(-90.3021060834143,-526.131812149225,194.018391542105));
#31044=CARTESIAN_POINT('',(-90.302175243761,-537.130288698218,200.368471352349));
#31045=CARTESIAN_POINT('Origin',(-99.3021060832809,-526.131769704399,194.018367036163));
#31046=CARTESIAN_POINT('Origin',(-297.302175240692,-537.129312467211,200.367907715666));
#31047=CARTESIAN_POINT('',(-288.302175240825,-537.129354912038,200.367932221609));
#31048=CARTESIAN_POINT('Origin',(-297.302175240692,-537.129312467211,200.367907715666));
#31049=CARTESIAN_POINT('',(-288.302106080479,-526.130878363045,194.017852411365));
#31050=CARTESIAN_POINT('',(-288.302175240825,-537.129354912038,200.367932221609));
#31051=CARTESIAN_POINT('Origin',(-297.302106080345,-526.130835918218,194.017827905422));
#31052=CARTESIAN_POINT('Origin',(-391.249472490554,-685.230730806452,-56.1479980020244));
#31053=CARTESIAN_POINT('',(-327.302175240247,-553.87938150779,171.356096549133));
#31054=CARTESIAN_POINT('',(262.697824751005,-553.882164001966,171.357703049819));
#31055=CARTESIAN_POINT('',(-327.302175240247,-553.87938150779,171.356096549133));
#31056=CARTESIAN_POINT('',(262.697824751005,-522.131764950275,226.350085795599));
#31057=CARTESIAN_POINT('',(262.697824751005,-553.882164001966,171.357703049819));
#31058=CARTESIAN_POINT('',(-327.302175240247,-522.128982456099,226.348479294913));
#31059=CARTESIAN_POINT('',(-327.302175240247,-522.128982456099,226.348479294913));
#31060=CARTESIAN_POINT('',(-327.302175240247,-553.87938150779,171.356096549133));
#31061=CARTESIAN_POINT('Origin',(-391.249403330208,-674.232254257459,-62.4980778122685));
#31062=CARTESIAN_POINT('',(-327.3021060799,-542.880904958797,165.006016738889));
#31063=CARTESIAN_POINT('',(262.697893911352,-542.883687452973,165.007623239575));
#31064=CARTESIAN_POINT('',(-327.3021060799,-542.880904958797,165.006016738889));
#31065=CARTESIAN_POINT('',(-327.3021060799,-511.130505907106,219.998399484669));
#31066=CARTESIAN_POINT('',(-327.3021060799,-542.880904958797,165.006016738889));
#31067=CARTESIAN_POINT('',(262.697893911351,-511.133288401282,220.000005985355));
#31068=CARTESIAN_POINT('',(-327.3021060799,-511.130505907106,219.998399484669));
#31069=CARTESIAN_POINT('',(262.697893911352,-542.883687452973,165.007623239575));
#31070=CARTESIAN_POINT('Origin',(-327.302175240247,-553.87938150779,171.356096549133));
#31071=CARTESIAN_POINT('',(262.697824751005,-553.882164001966,171.357703049819));
#31072=CARTESIAN_POINT('',(-327.302175240247,-553.87938150779,171.356096549133));
#31073=CARTESIAN_POINT('Origin',(262.697824751005,-553.882164001966,171.357703049819));
#31074=CARTESIAN_POINT('',(262.697824751005,-522.131764950275,226.350085795599));
#31075=CARTESIAN_POINT('Origin',(-327.302175240247,-522.128982456099,226.348479294913));
#31076=CARTESIAN_POINT('',(-327.302175240247,-522.128982456099,226.348479294913));
#31077=CARTESIAN_POINT('Origin',(-327.302175240247,-553.87938150779,171.356096549133));
#31078=CARTESIAN_POINT('Origin',(-296.201333258033,-635.883508821549,29.3278015002441));
#31079=CARTESIAN_POINT('',(-296.201333258033,-631.383494707935,37.122021985788));
#31080=CARTESIAN_POINT('Origin',(-296.201333258033,-635.883508821549,29.3278015002441));
#31081=CARTESIAN_POINT('',(-296.201333258033,-620.384983578334,30.7720020699101));
#31082=CARTESIAN_POINT('',(-296.201333258033,-631.383494707935,37.122021985788));
#31083=CARTESIAN_POINT('Origin',(-296.201333258033,-624.884997691948,22.9777815843661));
#31084=CARTESIAN_POINT('Origin',(-296.201333258031,-734.883819321062,-142.145049181723));
#31085=CARTESIAN_POINT('',(-296.201333258031,-730.383805207448,-134.350828696179));
#31086=CARTESIAN_POINT('Origin',(-296.201333258031,-734.883819321062,-142.145049181723));
#31087=CARTESIAN_POINT('',(-296.201333258031,-719.385294077847,-140.700848612057));
#31088=CARTESIAN_POINT('',(-296.201333258031,-730.383805207448,-134.350828696179));
#31089=CARTESIAN_POINT('Origin',(-296.201333258031,-723.885308191461,-148.4950690976));
#31090=CARTESIAN_POINT('Origin',(-296.201333258029,-833.884129820575,-313.617899863689));
#31091=CARTESIAN_POINT('',(-296.201333258029,-829.384115706961,-305.823679378145));
#31092=CARTESIAN_POINT('Origin',(-296.201333258029,-833.884129820575,-313.617899863689));
#31093=CARTESIAN_POINT('',(-296.201333258029,-818.38560457736,-312.173699294023));
#31094=CARTESIAN_POINT('',(-296.201333258029,-829.384115706961,-305.823679378145));
#31095=CARTESIAN_POINT('Origin',(-296.201333258029,-822.885618690974,-319.967919779567));
#31096=CARTESIAN_POINT('Origin',(-0.00133325802852044,-880.857925772416,
-394.978560841159));
#31097=CARTESIAN_POINT('',(-262.701333258028,-848.884176865956,-339.598634815502));
#31098=CARTESIAN_POINT('',(-262.701333258029,-553.883251640134,171.355819236822));
#31099=CARTESIAN_POINT('',(-262.701333258028,-848.884176865956,-339.598634815502));
#31100=CARTESIAN_POINT('',(-326.201333258029,-553.883251640134,171.355819236822));
#31101=CARTESIAN_POINT('',(-262.701333258029,-553.883251640134,171.355819236822));
#31102=CARTESIAN_POINT('',(-326.201333258029,-848.884176865956,-339.598634815502));
#31103=CARTESIAN_POINT('',(-326.201333258029,-848.884176865956,-339.598634815502));
#31104=CARTESIAN_POINT('',(-262.701333258028,-848.884176865956,-339.598634815502));
#31105=CARTESIAN_POINT('Origin',(-0.00133325802852079,-869.859414642815,
-401.328580757037));
#31106=CARTESIAN_POINT('',(-262.701333258028,-837.885665736355,-345.94865473138));
#31107=CARTESIAN_POINT('',(-262.701333258029,-542.884740510533,165.005799320944));
#31108=CARTESIAN_POINT('',(-262.701333258028,-837.885665736355,-345.94865473138));
#31109=CARTESIAN_POINT('',(-326.201333258029,-837.885665736355,-345.94865473138));
#31110=CARTESIAN_POINT('',(-262.701333258028,-837.885665736355,-345.94865473138));
#31111=CARTESIAN_POINT('',(-326.201333258029,-542.884740510533,165.005799320944));
#31112=CARTESIAN_POINT('',(-326.201333258029,-837.885665736355,-345.94865473138));
#31113=CARTESIAN_POINT('',(-262.701333258029,-542.884740510533,165.005799320944));
#31114=CARTESIAN_POINT('Origin',(-262.701333258028,-848.884176865956,-339.598634815502));
#31115=CARTESIAN_POINT('',(-262.701333258029,-553.883251640134,171.355819236822));
#31116=CARTESIAN_POINT('',(-262.701333258028,-848.884176865956,-339.598634815502));
#31117=CARTESIAN_POINT('Origin',(-262.701333258029,-553.883251640134,171.355819236822));
#31118=CARTESIAN_POINT('',(-326.201333258029,-553.883251640134,171.355819236822));
#31119=CARTESIAN_POINT('Origin',(-326.201333258029,-848.884176865956,-339.598634815502));
#31120=CARTESIAN_POINT('',(-326.201333258029,-848.884176865956,-339.598634815502));
#31121=CARTESIAN_POINT('Origin',(-262.701333258028,-848.884176865956,-339.598634815502));
#31122=CARTESIAN_POINT('Origin',(-98.6991580114631,-833.335569483613,-312.663468473821));
#31123=CARTESIAN_POINT('',(-107.69915801133,-833.335611928439,-312.663443967878));
#31124=CARTESIAN_POINT('Origin',(-98.6991580114631,-833.335569483613,-312.663468473821));
#31125=CARTESIAN_POINT('',(-107.699227171676,-822.337135379446,-319.013523778122));
#31126=CARTESIAN_POINT('',(-107.69915801133,-833.335611928439,-312.663443967878));
#31127=CARTESIAN_POINT('Origin',(-98.6992271718098,-822.33709293462,-319.013548284065));
#31128=CARTESIAN_POINT('Origin',(99.300841985601,-833.334635697429,-312.664007604555));
#31129=CARTESIAN_POINT('',(90.3008419857345,-833.334678142255,-312.663983098613));
#31130=CARTESIAN_POINT('Origin',(99.300841985601,-833.334635697429,-312.664007604555));
#31131=CARTESIAN_POINT('',(90.3007728253878,-822.336201593263,-319.014062908857));
#31132=CARTESIAN_POINT('',(90.3008419857345,-833.334678142255,-312.663983098613));
#31133=CARTESIAN_POINT('Origin',(99.3007728252544,-822.336159148436,-319.014087414799));
#31134=CARTESIAN_POINT('Origin',(297.300841982665,-833.333701911245,-312.66454673529));
#31135=CARTESIAN_POINT('',(288.300841982799,-833.333744356072,-312.664522229347));
#31136=CARTESIAN_POINT('Origin',(297.300841982665,-833.333701911245,-312.66454673529));
#31137=CARTESIAN_POINT('',(288.300772822452,-822.335267807078,-319.014602039592));
#31138=CARTESIAN_POINT('',(288.300841982799,-833.333744356072,-312.664522229347));
#31139=CARTESIAN_POINT('Origin',(297.300772822319,-822.335225362252,-319.014626545534));
#31140=CARTESIAN_POINT('Origin',(391.248139232526,-685.231397443842,-56.1491526325048));
#31141=CARTESIAN_POINT('',(327.30084198222,-816.583349905157,-283.652898941708));
#31142=CARTESIAN_POINT('',(-262.699158009032,-816.586132399338,-283.651292441029));
#31143=CARTESIAN_POINT('',(327.30084198222,-816.583349905157,-283.652898941708));
#31144=CARTESIAN_POINT('',(-262.699158009031,-848.336531451029,-338.643675186809));
#31145=CARTESIAN_POINT('',(-262.699158009032,-816.586132399338,-283.651292441029));
#31146=CARTESIAN_POINT('',(327.300841982221,-848.333748956848,-338.645281687488));
#31147=CARTESIAN_POINT('',(327.300841982221,-848.333748956848,-338.645281687488));
#31148=CARTESIAN_POINT('',(327.30084198222,-816.583349905157,-283.652898941708));
#31149=CARTESIAN_POINT('Origin',(391.248070072179,-674.232920894849,-62.4992324427489));
#31150=CARTESIAN_POINT('',(327.300772821873,-805.584873356164,-290.002978751952));
#31151=CARTESIAN_POINT('',(-262.699227169378,-805.587655850345,-290.001372251273));
#31152=CARTESIAN_POINT('',(327.300772821873,-805.584873356164,-290.002978751952));
#31153=CARTESIAN_POINT('',(327.300772821874,-837.335272407855,-344.995361497732));
#31154=CARTESIAN_POINT('',(327.300772821873,-805.584873356164,-290.002978751952));
#31155=CARTESIAN_POINT('',(-262.699227169378,-837.338054902036,-344.993754997053));
#31156=CARTESIAN_POINT('',(327.300772821874,-837.335272407855,-344.995361497732));
#31157=CARTESIAN_POINT('',(-262.699227169378,-805.587655850345,-290.001372251273));
#31158=CARTESIAN_POINT('Origin',(327.30084198222,-816.583349905157,-283.652898941708));
#31159=CARTESIAN_POINT('',(-262.699158009032,-816.586132399338,-283.651292441029));
#31160=CARTESIAN_POINT('',(327.30084198222,-816.583349905157,-283.652898941708));
#31161=CARTESIAN_POINT('Origin',(-262.699158009032,-816.586132399338,-283.651292441029));
#31162=CARTESIAN_POINT('',(-262.699158009031,-848.336531451029,-338.643675186809));
#31163=CARTESIAN_POINT('Origin',(327.300841982221,-848.333748956848,-338.645281687488));
#31164=CARTESIAN_POINT('',(327.300841982221,-848.333748956848,-338.645281687488));
#31165=CARTESIAN_POINT('Origin',(327.30084198222,-816.583349905157,-283.652898941708));
#31166=CARTESIAN_POINT('Origin',(-411.000556942817,-537.996237603978,-429.826812462452));
#31167=CARTESIAN_POINT('',(-251.582431340073,-755.289566540481,-304.368610542448));
#31168=CARTESIAN_POINT('',(-400.,-532.5,-433.));
#31169=CARTESIAN_POINT('',(-400.,-532.5,-433.));
#31170=CARTESIAN_POINT('',(-262.58298828289,-760.785804144459,-301.195423004899));
#31171=CARTESIAN_POINT('',(-262.58298828289,-760.785804144459,-301.195423004899));
#31172=CARTESIAN_POINT('',(-411.000556942817,-537.996237603978,-429.826812462452));
#31173=CARTESIAN_POINT('',(-411.000556942817,-537.996237603978,-429.826812462452));
#31174=CARTESIAN_POINT('',(-411.000556942817,-537.996237603978,-429.826812462452));
#31175=CARTESIAN_POINT('Origin',(-411.000556942817,-537.996237603978,-429.826812462452));
#31176=CARTESIAN_POINT('',(-400.004719499877,-282.502358016311,0.00136137272609138));
#31177=CARTESIAN_POINT('',(-400.,-532.5,-433.));
#31178=CARTESIAN_POINT('',(-411.005276442694,-287.998595620289,3.17454891027458));
#31179=CARTESIAN_POINT('',(-411.000556942817,-537.996237603978,-429.826812462452));
#31180=CARTESIAN_POINT('',(-411.005276442694,-287.998595620289,3.17454891027458));
#31181=CARTESIAN_POINT('Origin',(-411.005276442694,-287.998595620289,3.17454891027458));
#31182=CARTESIAN_POINT('',(-251.58715083995,-505.291924556791,128.632750830278));
#31183=CARTESIAN_POINT('',(-400.004719499877,-282.502358016311,0.00136137272609138));
#31184=CARTESIAN_POINT('',(-262.587707782767,-510.788162160769,131.805938367827));
#31185=CARTESIAN_POINT('',(-411.005276442694,-287.998595620289,3.17454891027458));
#31186=CARTESIAN_POINT('',(-262.587707782767,-510.788162160769,131.805938367827));
#31187=CARTESIAN_POINT('Origin',(-262.58298828289,-760.785804144459,-301.195423004899));
#31188=CARTESIAN_POINT('',(-251.582431340073,-755.289566540481,-304.368610542448));
#31189=CARTESIAN_POINT('',(-262.58298828289,-760.785804144459,-301.195423004899));
#31190=CARTESIAN_POINT('Origin',(-417.015099327983,-208.354366262308,120.290920090289));
#31191=CARTESIAN_POINT('Origin',(-406.014542385166,-202.85812865833,117.117732552741));
#31192=CARTESIAN_POINT('Origin',(-262.7,-799.237226496489,-279.002428587459));
#31193=CARTESIAN_POINT('',(-250.,-799.237226496489,-279.002428587459));
#31194=CARTESIAN_POINT('',(-250.,-760.266369128196,-301.502923603794));
#31195=CARTESIAN_POINT('',(-250.,-799.237226496489,-279.002428587459));
#31196=CARTESIAN_POINT('',(-262.7,-799.237226496489,-279.002428587459));
#31197=CARTESIAN_POINT('',(-262.7,-799.237226496489,-279.002428587459));
#31198=CARTESIAN_POINT('',(-262.7,-760.266369128196,-301.502923603794));
#31199=CARTESIAN_POINT('',(-262.7,-799.237226496489,-279.002428587459));
#31200=CARTESIAN_POINT('',(-262.7,-760.266369128196,-301.502923603794));
#31201=CARTESIAN_POINT('Origin',(-262.7,-760.266369128196,-301.502923603794));
#31202=CARTESIAN_POINT('',(-250.,-510.263080007906,131.502773152548));
#31203=CARTESIAN_POINT('',(-250.,-760.266369128196,-301.502923603794));
#31204=CARTESIAN_POINT('',(-262.7,-510.263080007906,131.502773152548));
#31205=CARTESIAN_POINT('',(-262.7,-760.266369128196,-301.502923603794));
#31206=CARTESIAN_POINT('',(-262.7,-510.263080007906,131.502773152548));
#31207=CARTESIAN_POINT('Origin',(-262.7,-549.2339373762,154.003268168884));
#31208=CARTESIAN_POINT('',(-250.,-549.2339373762,154.003268168884));
#31209=CARTESIAN_POINT('',(-250.,-549.2339373762,154.003268168884));
#31210=CARTESIAN_POINT('',(-262.7,-549.2339373762,154.003268168884));
#31211=CARTESIAN_POINT('',(-262.7,-549.2339373762,154.003268168884));
#31212=CARTESIAN_POINT('',(-262.7,-549.2339373762,154.003268168884));
#31213=CARTESIAN_POINT('Origin',(-262.7,-799.237226496489,-279.002428587459));
#31214=CARTESIAN_POINT('',(-250.,-799.237226496489,-279.002428587459));
#31215=CARTESIAN_POINT('',(-262.7,-799.237226496489,-279.002428587459));
#31216=CARTESIAN_POINT('Origin',(-262.7,0.,0.));
#31217=CARTESIAN_POINT('Origin',(-250.,0.,0.));
#31218=CARTESIAN_POINT('Origin',(463.499333370986,293.375,15.8749999999999));
#31219=CARTESIAN_POINT('',(463.499333370986,277.5,15.8749999999999));
#31220=CARTESIAN_POINT('',(463.499333370986,277.5,66.6749999999998));
#31221=CARTESIAN_POINT('',(463.499333370986,277.5,15.8749999999999));
#31222=CARTESIAN_POINT('',(463.499333370986,293.375,15.8749999999999));
#31223=CARTESIAN_POINT('',(463.499333370986,293.375,15.8749999999999));
#31224=CARTESIAN_POINT('',(463.499333370986,293.375,66.6749999999998));
#31225=CARTESIAN_POINT('',(463.499333370986,293.375,15.8749999999999));
#31226=CARTESIAN_POINT('',(463.499333370986,293.375,66.6749999999998));
#31227=CARTESIAN_POINT('Origin',(463.499333370986,293.375,15.8749999999999));
#31228=CARTESIAN_POINT('',(-463.500666629014,277.5,15.8749999999999));
#31229=CARTESIAN_POINT('',(463.499333370986,277.5,15.8749999999999));
#31230=CARTESIAN_POINT('',(-463.500666629014,293.375,15.8749999999999));
#31231=CARTESIAN_POINT('',(-463.500666629014,293.375,15.8749999999999));
#31232=CARTESIAN_POINT('',(463.499333370986,293.375,15.8749999999999));
#31233=CARTESIAN_POINT('Origin',(-463.500666629014,293.375,15.8749999999999));
#31234=CARTESIAN_POINT('',(-463.500666629014,277.5,66.6749999999998));
#31235=CARTESIAN_POINT('',(-463.500666629014,277.5,15.8749999999999));
#31236=CARTESIAN_POINT('',(-463.500666629014,293.375,66.6749999999998));
#31237=CARTESIAN_POINT('',(-463.500666629014,293.375,66.6749999999998));
#31238=CARTESIAN_POINT('',(-463.500666629014,293.375,15.8749999999999));
#31239=CARTESIAN_POINT('Origin',(463.499333370986,293.375,66.6749999999998));
#31240=CARTESIAN_POINT('',(463.499333370986,277.5,66.6749999999998));
#31241=CARTESIAN_POINT('',(463.499333370986,293.375,66.6749999999998));
#31242=CARTESIAN_POINT('Origin',(0.,293.375,0.));
#31243=CARTESIAN_POINT('Origin',(0.,277.5,0.));
#31244=CARTESIAN_POINT('Origin',(412.7,277.5,-453.125));
#31245=CARTESIAN_POINT('',(412.7,293.375,-453.125));
#31246=CARTESIAN_POINT('',(412.7,293.375,15.8749999999999));
#31247=CARTESIAN_POINT('',(412.7,293.375,-453.125));
#31248=CARTESIAN_POINT('',(412.7,277.5,-453.125));
#31249=CARTESIAN_POINT('',(412.7,277.5,-453.125));
#31250=CARTESIAN_POINT('',(412.7,277.5,15.8749999999999));
#31251=CARTESIAN_POINT('',(412.7,277.5,-453.125));
#31252=CARTESIAN_POINT('',(412.7,277.5,15.8749999999999));
#31253=CARTESIAN_POINT('Origin',(412.7,277.5,-453.125));
#31254=CARTESIAN_POINT('',(463.499333370981,293.375,-453.125));
#31255=CARTESIAN_POINT('',(412.7,293.375,-453.125));
#31256=CARTESIAN_POINT('',(463.499333370981,277.5,-453.125));
#31257=CARTESIAN_POINT('',(463.499333370981,277.5,-453.125));
#31258=CARTESIAN_POINT('',(412.7,277.5,-453.125));
#31259=CARTESIAN_POINT('Origin',(463.499333370981,277.5,-453.125));
#31260=CARTESIAN_POINT('',(463.499333370986,293.375,15.8749999999999));
#31261=CARTESIAN_POINT('',(463.499333370981,293.375,-453.125));
#31262=CARTESIAN_POINT('',(463.499333370986,277.5,15.8749999999999));
#31263=CARTESIAN_POINT('',(463.499333370986,277.5,15.8749999999999));
#31264=CARTESIAN_POINT('',(463.499333370981,277.5,-453.125));
#31265=CARTESIAN_POINT('Origin',(412.7,277.5,15.8749999999999));
#31266=CARTESIAN_POINT('',(412.7,293.375,15.8749999999999));
#31267=CARTESIAN_POINT('',(412.7,277.5,15.8749999999999));
#31268=CARTESIAN_POINT('Origin',(0.,277.5,0.));
#31269=CARTESIAN_POINT('Origin',(0.,293.375,0.));
#31270=CARTESIAN_POINT('Origin',(-412.7,277.5,-453.125));
#31271=CARTESIAN_POINT('',(-412.7,293.375,-453.125));
#31272=CARTESIAN_POINT('',(-412.7,293.375,15.8749999999999));
#31273=CARTESIAN_POINT('',(-412.7,293.375,-453.125));
#31274=CARTESIAN_POINT('',(-412.7,277.5,15.8749999999999));
#31275=CARTESIAN_POINT('',(-412.7,277.5,15.8749999999999));
#31276=CARTESIAN_POINT('',(-412.7,277.5,-453.125));
#31277=CARTESIAN_POINT('',(-412.7,277.5,-453.125));
#31278=CARTESIAN_POINT('',(-412.7,277.5,-453.125));
#31279=CARTESIAN_POINT('Origin',(-412.7,277.5,-453.125));
#31280=CARTESIAN_POINT('',(-463.499333370981,293.375,-453.125));
#31281=CARTESIAN_POINT('',(-412.7,293.375,-453.125));
#31282=CARTESIAN_POINT('',(-463.499333370981,277.5,-453.125));
#31283=CARTESIAN_POINT('',(-412.7,277.5,-453.125));
#31284=CARTESIAN_POINT('',(-463.499333370981,277.5,-453.125));
#31285=CARTESIAN_POINT('Origin',(-463.499333370981,277.5,-453.125));
#31286=CARTESIAN_POINT('',(-463.499333370986,293.375,15.8749999999999));
#31287=CARTESIAN_POINT('',(-463.499333370981,293.375,-453.125));
#31288=CARTESIAN_POINT('',(-463.499333370986,277.5,15.8749999999999));
#31289=CARTESIAN_POINT('',(-463.499333370981,277.5,-453.125));
#31290=CARTESIAN_POINT('',(-463.499333370986,277.5,15.8749999999999));
#31291=CARTESIAN_POINT('Origin',(-412.7,277.5,15.8749999999999));
#31292=CARTESIAN_POINT('',(-412.7,293.375,15.8749999999999));
#31293=CARTESIAN_POINT('',(-412.7,277.5,15.8749999999999));
#31294=CARTESIAN_POINT('Origin',(0.,277.5,0.));
#31295=CARTESIAN_POINT('Origin',(0.,293.375,0.));
#31296=CARTESIAN_POINT('Origin',(579.199999999996,191.625,-54.1249999999996));
#31297=CARTESIAN_POINT('',(579.199999999996,191.625,-63.1249999999996));
#31298=CARTESIAN_POINT('Origin',(579.199999999996,191.625,-54.1249999999996));
#31299=CARTESIAN_POINT('',(579.199999999996,207.5,-63.1249999999996));
#31300=CARTESIAN_POINT('',(579.199999999996,191.625,-63.1249999999996));
#31301=CARTESIAN_POINT('Origin',(579.199999999996,207.5,-54.1249999999996));
#31302=CARTESIAN_POINT('Origin',(579.199999999998,191.625,-174.125));
#31303=CARTESIAN_POINT('',(579.199999999998,191.625,-183.125));
#31304=CARTESIAN_POINT('Origin',(579.199999999998,191.625,-174.125));
#31305=CARTESIAN_POINT('',(579.199999999998,207.5,-183.125));
#31306=CARTESIAN_POINT('',(579.199999999998,191.625,-183.125));
#31307=CARTESIAN_POINT('Origin',(579.199999999998,207.5,-174.125));
#31308=CARTESIAN_POINT('Origin',(579.199999999999,191.625,-294.125));
#31309=CARTESIAN_POINT('',(579.199999999999,191.625,-303.125));
#31310=CARTESIAN_POINT('Origin',(579.199999999999,191.625,-294.125));
#31311=CARTESIAN_POINT('',(579.199999999999,207.5,-303.125));
#31312=CARTESIAN_POINT('',(579.199999999999,191.625,-303.125));
#31313=CARTESIAN_POINT('Origin',(579.199999999999,207.5,-294.125));
#31314=CARTESIAN_POINT('Origin',(579.2,191.625,-414.125));
#31315=CARTESIAN_POINT('',(579.2,191.625,-423.125));
#31316=CARTESIAN_POINT('Origin',(579.2,191.625,-414.125));
#31317=CARTESIAN_POINT('',(579.2,207.5,-423.125));
#31318=CARTESIAN_POINT('',(579.2,191.625,-423.125));
#31319=CARTESIAN_POINT('Origin',(579.2,207.5,-414.125));
#31320=CARTESIAN_POINT('Origin',(0.,191.625,0.));
#31321=CARTESIAN_POINT('',(412.7,191.625,15.8749999999999));
#31322=CARTESIAN_POINT('',(412.7,191.625,-453.125));
#31323=CARTESIAN_POINT('',(412.7,191.625,-453.125));
#31324=CARTESIAN_POINT('',(595.7,191.625,-453.125));
#31325=CARTESIAN_POINT('',(412.7,191.625,-453.125));
#31326=CARTESIAN_POINT('',(595.7,191.625,15.8749999999999));
#31327=CARTESIAN_POINT('',(595.7,191.625,-453.125));
#31328=CARTESIAN_POINT('',(412.7,191.625,15.8749999999999));
#31329=CARTESIAN_POINT('Origin',(0.,207.5,0.));
#31330=CARTESIAN_POINT('',(412.7,207.5,15.8749999999999));
#31331=CARTESIAN_POINT('',(412.7,207.5,-453.125));
#31332=CARTESIAN_POINT('',(412.7,207.5,-453.125));
#31333=CARTESIAN_POINT('',(595.7,207.5,15.8749999999999));
#31334=CARTESIAN_POINT('',(412.7,207.5,15.8749999999999));
#31335=CARTESIAN_POINT('',(595.7,207.5,-453.125));
#31336=CARTESIAN_POINT('',(595.7,207.5,-453.125));
#31337=CARTESIAN_POINT('',(412.7,207.5,-453.125));
#31338=CARTESIAN_POINT('Origin',(412.7,191.625,-453.125));
#31339=CARTESIAN_POINT('',(412.7,191.625,-453.125));
#31340=CARTESIAN_POINT('',(412.7,191.625,15.8749999999999));
#31341=CARTESIAN_POINT('Origin',(412.7,191.625,-453.125));
#31342=CARTESIAN_POINT('',(595.7,191.625,-453.125));
#31343=CARTESIAN_POINT('Origin',(595.7,191.625,-453.125));
#31344=CARTESIAN_POINT('',(595.7,191.625,15.8749999999999));
#31345=CARTESIAN_POINT('Origin',(412.7,191.625,15.8749999999999));
#31346=CARTESIAN_POINT('Origin',(-265.5,207.5,135.874999999997));
#31347=CARTESIAN_POINT('',(-265.5,207.5,144.874999999997));
#31348=CARTESIAN_POINT('Origin',(-265.5,207.5,135.874999999997));
#31349=CARTESIAN_POINT('',(-265.5,191.625,144.874999999997));
#31350=CARTESIAN_POINT('',(-265.5,207.5,144.874999999997));
#31351=CARTESIAN_POINT('Origin',(-265.5,191.625,135.874999999997));
#31352=CARTESIAN_POINT('Origin',(-88.5,207.5,135.874999999999));
#31353=CARTESIAN_POINT('',(-88.5,207.5,144.874999999999));
#31354=CARTESIAN_POINT('Origin',(-88.5,207.5,135.874999999999));
#31355=CARTESIAN_POINT('',(-88.5,191.625,144.874999999999));
#31356=CARTESIAN_POINT('',(-88.5,207.5,144.874999999999));
#31357=CARTESIAN_POINT('Origin',(-88.5,191.625,135.874999999999));
#31358=CARTESIAN_POINT('Origin',(88.5,207.5,135.875));
#31359=CARTESIAN_POINT('',(88.5,207.5,144.875));
#31360=CARTESIAN_POINT('Origin',(88.5,207.5,135.875));
#31361=CARTESIAN_POINT('',(88.5,191.625,144.875));
#31362=CARTESIAN_POINT('',(88.5,207.5,144.875));
#31363=CARTESIAN_POINT('Origin',(88.5,191.625,135.875));
#31364=CARTESIAN_POINT('Origin',(265.5,207.5,135.875000000001));
#31365=CARTESIAN_POINT('',(265.5,207.5,144.875000000001));
#31366=CARTESIAN_POINT('Origin',(265.5,207.5,135.875000000001));
#31367=CARTESIAN_POINT('',(265.5,191.625,144.875000000001));
#31368=CARTESIAN_POINT('',(265.5,207.5,144.875000000001));
#31369=CARTESIAN_POINT('Origin',(265.5,191.625,135.875000000001));
#31370=CARTESIAN_POINT('Origin',(-579.2,207.5,65.8749999999998));
#31371=CARTESIAN_POINT('',(-579.2,207.5,74.8749999999998));
#31372=CARTESIAN_POINT('Origin',(-579.2,207.5,65.8749999999998));
#31373=CARTESIAN_POINT('',(-579.2,191.625,74.8749999999998));
#31374=CARTESIAN_POINT('',(-579.2,207.5,74.8749999999998));
#31375=CARTESIAN_POINT('Origin',(-579.2,191.625,65.8749999999998));
#31376=CARTESIAN_POINT('Origin',(579.2,207.5,65.8749999999999));
#31377=CARTESIAN_POINT('',(579.2,207.5,74.8749999999999));
#31378=CARTESIAN_POINT('Origin',(579.2,207.5,65.8749999999999));
#31379=CARTESIAN_POINT('',(579.2,191.625,74.8749999999999));
#31380=CARTESIAN_POINT('',(579.2,207.5,74.8749999999999));
#31381=CARTESIAN_POINT('Origin',(579.2,191.625,65.8749999999999));
#31382=CARTESIAN_POINT('Origin',(595.7,207.5,15.8749999999999));
#31383=CARTESIAN_POINT('',(595.7,191.625,15.8749999999999));
#31384=CARTESIAN_POINT('',(595.7,191.625,152.875));
#31385=CARTESIAN_POINT('',(595.7,191.625,15.8749999999999));
#31386=CARTESIAN_POINT('',(595.7,207.5,15.8749999999999));
#31387=CARTESIAN_POINT('',(595.7,207.5,15.8749999999999));
#31388=CARTESIAN_POINT('',(595.7,207.5,152.875));
#31389=CARTESIAN_POINT('',(595.7,207.5,15.8749999999999));
#31390=CARTESIAN_POINT('',(595.7,207.5,152.875));
#31391=CARTESIAN_POINT('Origin',(595.7,207.5,15.8749999999999));
#31392=CARTESIAN_POINT('',(-595.7,191.625,15.8749999999997));
#31393=CARTESIAN_POINT('',(595.7,191.625,15.8749999999999));
#31394=CARTESIAN_POINT('',(-595.7,207.5,15.8749999999997));
#31395=CARTESIAN_POINT('',(-595.7,207.5,15.8749999999997));
#31396=CARTESIAN_POINT('',(595.7,207.5,15.8749999999999));
#31397=CARTESIAN_POINT('Origin',(-595.7,207.5,15.8749999999997));
#31398=CARTESIAN_POINT('',(-595.7,191.625,152.875));
#31399=CARTESIAN_POINT('',(-595.7,191.625,15.8749999999997));
#31400=CARTESIAN_POINT('',(-595.7,207.5,152.875));
#31401=CARTESIAN_POINT('',(-595.7,207.5,152.875));
#31402=CARTESIAN_POINT('',(-595.7,207.5,15.8749999999997));
#31403=CARTESIAN_POINT('Origin',(595.7,207.5,152.875));
#31404=CARTESIAN_POINT('',(595.7,191.625,152.875));
#31405=CARTESIAN_POINT('',(595.7,207.5,152.875));
#31406=CARTESIAN_POINT('Origin',(0.,207.5,0.));
#31407=CARTESIAN_POINT('Origin',(0.,191.625,0.));
#31408=CARTESIAN_POINT('Origin',(463.699999999996,277.5,-360.509999999995));
#31409=CARTESIAN_POINT('',(463.699999999996,277.5,-347.809999999995));
#31410=CARTESIAN_POINT('',(566.699999999996,232.5,-347.809999999995));
#31411=CARTESIAN_POINT('',(463.699999999996,277.5,-347.809999999995));
#31412=CARTESIAN_POINT('',(566.699999999996,232.5,-360.509999999995));
#31413=CARTESIAN_POINT('',(566.699999999996,232.5,-360.509999999995));
#31414=CARTESIAN_POINT('',(463.699999999996,277.5,-360.509999999995));
#31415=CARTESIAN_POINT('',(463.699999999996,277.5,-360.509999999995));
#31416=CARTESIAN_POINT('',(463.699999999996,277.5,-360.509999999995));
#31417=CARTESIAN_POINT('Origin',(566.699999999996,232.5,-360.509999999995));
#31418=CARTESIAN_POINT('',(566.699999999996,207.5,-347.809999999995));
#31419=CARTESIAN_POINT('',(566.699999999996,232.5,-347.809999999995));
#31420=CARTESIAN_POINT('',(566.699999999996,207.5,-360.509999999995));
#31421=CARTESIAN_POINT('',(566.699999999996,207.5,-360.509999999995));
#31422=CARTESIAN_POINT('',(566.699999999996,232.5,-360.509999999995));
#31423=CARTESIAN_POINT('Origin',(566.699999999996,207.5,-360.509999999995));
#31424=CARTESIAN_POINT('',(422.699999999996,207.5,-347.809999999995));
#31425=CARTESIAN_POINT('',(566.699999999996,207.5,-347.809999999995));
#31426=CARTESIAN_POINT('',(422.699999999996,207.5,-360.509999999995));
#31427=CARTESIAN_POINT('',(422.699999999996,207.5,-360.509999999995));
#31428=CARTESIAN_POINT('',(566.699999999996,207.5,-360.509999999995));
#31429=CARTESIAN_POINT('Origin',(422.699999999996,207.5,-360.509999999995));
#31430=CARTESIAN_POINT('',(412.699999999996,217.5,-347.809999999995));
#31431=CARTESIAN_POINT('',(422.699999999996,207.5,-347.809999999995));
#31432=CARTESIAN_POINT('',(412.699999999996,217.5,-360.509999999995));
#31433=CARTESIAN_POINT('',(412.699999999996,217.5,-360.509999999995));
#31434=CARTESIAN_POINT('',(422.699999999996,207.5,-360.509999999995));
#31435=CARTESIAN_POINT('Origin',(412.699999999996,217.5,-360.509999999995));
#31436=CARTESIAN_POINT('',(412.699999999996,267.5,-347.809999999995));
#31437=CARTESIAN_POINT('',(412.699999999996,217.5,-347.809999999995));
#31438=CARTESIAN_POINT('',(412.699999999996,267.5,-360.509999999995));
#31439=CARTESIAN_POINT('',(412.699999999996,267.5,-360.509999999995));
#31440=CARTESIAN_POINT('',(412.699999999996,217.5,-360.509999999995));
#31441=CARTESIAN_POINT('Origin',(412.699999999996,267.5,-360.509999999995));
#31442=CARTESIAN_POINT('',(422.699999999996,277.5,-347.809999999995));
#31443=CARTESIAN_POINT('',(412.699999999996,267.5,-347.809999999995));
#31444=CARTESIAN_POINT('',(422.699999999996,277.5,-360.509999999995));
#31445=CARTESIAN_POINT('',(422.699999999996,277.5,-360.509999999995));
#31446=CARTESIAN_POINT('',(412.699999999996,267.5,-360.509999999995));
#31447=CARTESIAN_POINT('Origin',(422.699999999996,277.5,-360.509999999995));
#31448=CARTESIAN_POINT('',(422.699999999996,277.5,-347.809999999995));
#31449=CARTESIAN_POINT('',(422.699999999996,277.5,-360.509999999995));
#31450=CARTESIAN_POINT('Origin',(0.,0.,-360.509999999995));
#31451=CARTESIAN_POINT('Origin',(0.,0.,-347.809999999995));
#31452=CARTESIAN_POINT('Origin',(463.699999999997,277.5,-240.509999999995));
#31453=CARTESIAN_POINT('',(463.699999999997,277.5,-227.809999999995));
#31454=CARTESIAN_POINT('',(566.699999999997,232.5,-227.809999999995));
#31455=CARTESIAN_POINT('',(463.699999999997,277.5,-227.809999999995));
#31456=CARTESIAN_POINT('',(566.699999999997,232.5,-240.509999999995));
#31457=CARTESIAN_POINT('',(566.699999999997,232.5,-240.509999999995));
#31458=CARTESIAN_POINT('',(463.699999999997,277.5,-240.509999999995));
#31459=CARTESIAN_POINT('',(463.699999999997,277.5,-240.509999999995));
#31460=CARTESIAN_POINT('',(463.699999999997,277.5,-240.509999999995));
#31461=CARTESIAN_POINT('Origin',(566.699999999997,232.5,-240.509999999995));
#31462=CARTESIAN_POINT('',(566.699999999997,207.5,-227.809999999995));
#31463=CARTESIAN_POINT('',(566.699999999997,232.5,-227.809999999995));
#31464=CARTESIAN_POINT('',(566.699999999997,207.5,-240.509999999995));
#31465=CARTESIAN_POINT('',(566.699999999997,207.5,-240.509999999995));
#31466=CARTESIAN_POINT('',(566.699999999997,232.5,-240.509999999995));
#31467=CARTESIAN_POINT('Origin',(566.699999999997,207.5,-240.509999999995));
#31468=CARTESIAN_POINT('',(422.699999999998,207.5,-227.809999999995));
#31469=CARTESIAN_POINT('',(566.699999999997,207.5,-227.809999999995));
#31470=CARTESIAN_POINT('',(422.699999999998,207.5,-240.509999999995));
#31471=CARTESIAN_POINT('',(422.699999999998,207.5,-240.509999999995));
#31472=CARTESIAN_POINT('',(566.699999999997,207.5,-240.509999999995));
#31473=CARTESIAN_POINT('Origin',(422.699999999998,207.5,-240.509999999995));
#31474=CARTESIAN_POINT('',(412.699999999998,217.5,-227.809999999995));
#31475=CARTESIAN_POINT('',(422.699999999998,207.5,-227.809999999995));
#31476=CARTESIAN_POINT('',(412.699999999998,217.5,-240.509999999995));
#31477=CARTESIAN_POINT('',(412.699999999998,217.5,-240.509999999995));
#31478=CARTESIAN_POINT('',(422.699999999998,207.5,-240.509999999995));
#31479=CARTESIAN_POINT('Origin',(412.699999999998,217.5,-240.509999999995));
#31480=CARTESIAN_POINT('',(412.699999999998,267.5,-227.809999999995));
#31481=CARTESIAN_POINT('',(412.699999999998,217.5,-227.809999999995));
#31482=CARTESIAN_POINT('',(412.699999999998,267.5,-240.509999999995));
#31483=CARTESIAN_POINT('',(412.699999999998,267.5,-240.509999999995));
#31484=CARTESIAN_POINT('',(412.699999999998,217.5,-240.509999999995));
#31485=CARTESIAN_POINT('Origin',(412.699999999998,267.5,-240.509999999995));
#31486=CARTESIAN_POINT('',(422.699999999998,277.5,-227.809999999995));
#31487=CARTESIAN_POINT('',(412.699999999998,267.5,-227.809999999995));
#31488=CARTESIAN_POINT('',(422.699999999998,277.5,-240.509999999995));
#31489=CARTESIAN_POINT('',(422.699999999998,277.5,-240.509999999995));
#31490=CARTESIAN_POINT('',(412.699999999998,267.5,-240.509999999995));
#31491=CARTESIAN_POINT('Origin',(422.699999999998,277.5,-240.509999999995));
#31492=CARTESIAN_POINT('',(422.699999999998,277.5,-227.809999999995));
#31493=CARTESIAN_POINT('',(422.699999999998,277.5,-240.509999999995));
#31494=CARTESIAN_POINT('Origin',(1.24988860768035E-12,0.,-240.509999999995));
#31495=CARTESIAN_POINT('Origin',(1.24988860768035E-12,0.,-227.809999999995));
#31496=CARTESIAN_POINT('Origin',(463.699999999999,277.5,-120.509999999995));
#31497=CARTESIAN_POINT('',(463.699999999999,277.5,-107.809999999995));
#31498=CARTESIAN_POINT('',(566.699999999999,232.5,-107.809999999995));
#31499=CARTESIAN_POINT('',(463.699999999999,277.5,-107.809999999995));
#31500=CARTESIAN_POINT('',(566.699999999999,232.5,-120.509999999995));
#31501=CARTESIAN_POINT('',(566.699999999999,232.5,-120.509999999995));
#31502=CARTESIAN_POINT('',(463.699999999999,277.5,-120.509999999995));
#31503=CARTESIAN_POINT('',(463.699999999999,277.5,-120.509999999995));
#31504=CARTESIAN_POINT('',(463.699999999999,277.5,-120.509999999995));
#31505=CARTESIAN_POINT('Origin',(566.699999999999,232.5,-120.509999999995));
#31506=CARTESIAN_POINT('',(566.699999999999,207.5,-107.809999999995));
#31507=CARTESIAN_POINT('',(566.699999999999,232.5,-107.809999999995));
#31508=CARTESIAN_POINT('',(566.699999999999,207.5,-120.509999999995));
#31509=CARTESIAN_POINT('',(566.699999999999,207.5,-120.509999999995));
#31510=CARTESIAN_POINT('',(566.699999999999,232.5,-120.509999999995));
#31511=CARTESIAN_POINT('Origin',(566.699999999999,207.5,-120.509999999995));
#31512=CARTESIAN_POINT('',(422.699999999999,207.5,-107.809999999995));
#31513=CARTESIAN_POINT('',(566.699999999999,207.5,-107.809999999995));
#31514=CARTESIAN_POINT('',(422.699999999999,207.5,-120.509999999995));
#31515=CARTESIAN_POINT('',(422.699999999999,207.5,-120.509999999995));
#31516=CARTESIAN_POINT('',(566.699999999999,207.5,-120.509999999995));
#31517=CARTESIAN_POINT('Origin',(422.699999999999,207.5,-120.509999999995));
#31518=CARTESIAN_POINT('',(412.699999999999,217.5,-107.809999999995));
#31519=CARTESIAN_POINT('',(422.699999999999,207.5,-107.809999999995));
#31520=CARTESIAN_POINT('',(412.699999999999,217.5,-120.509999999995));
#31521=CARTESIAN_POINT('',(412.699999999999,217.5,-120.509999999995));
#31522=CARTESIAN_POINT('',(422.699999999999,207.5,-120.509999999995));
#31523=CARTESIAN_POINT('Origin',(412.699999999999,217.5,-120.509999999995));
#31524=CARTESIAN_POINT('',(412.699999999999,267.5,-107.809999999995));
#31525=CARTESIAN_POINT('',(412.699999999999,217.5,-107.809999999995));
#31526=CARTESIAN_POINT('',(412.699999999999,267.5,-120.509999999995));
#31527=CARTESIAN_POINT('',(412.699999999999,267.5,-120.509999999995));
#31528=CARTESIAN_POINT('',(412.699999999999,217.5,-120.509999999995));
#31529=CARTESIAN_POINT('Origin',(412.699999999999,267.5,-120.509999999995));
#31530=CARTESIAN_POINT('',(422.699999999999,277.5,-107.809999999995));
#31531=CARTESIAN_POINT('',(412.699999999999,267.5,-107.809999999995));
#31532=CARTESIAN_POINT('',(422.699999999999,277.5,-120.509999999995));
#31533=CARTESIAN_POINT('',(422.699999999999,277.5,-120.509999999995));
#31534=CARTESIAN_POINT('',(412.699999999999,267.5,-120.509999999995));
#31535=CARTESIAN_POINT('Origin',(422.699999999999,277.5,-120.509999999995));
#31536=CARTESIAN_POINT('',(422.699999999999,277.5,-107.809999999995));
#31537=CARTESIAN_POINT('',(422.699999999999,277.5,-120.509999999995));
#31538=CARTESIAN_POINT('Origin',(2.49977721536069E-12,0.,-120.509999999995));
#31539=CARTESIAN_POINT('Origin',(2.49977721536069E-12,0.,-107.809999999995));
#31540=CARTESIAN_POINT('Origin',(-6.35,277.5,66.6749999999998));
#31541=CARTESIAN_POINT('',(6.35,277.5,66.6749999999998));
#31542=CARTESIAN_POINT('',(6.35,232.5,152.875));
#31543=CARTESIAN_POINT('',(6.35,277.5,66.6749999999998));
#31544=CARTESIAN_POINT('',(-6.35,277.5,66.6749999999998));
#31545=CARTESIAN_POINT('',(-6.35,277.5,66.6749999999998));
#31546=CARTESIAN_POINT('',(-6.35,232.5,152.875));
#31547=CARTESIAN_POINT('',(-6.35,277.5,66.6749999999998));
#31548=CARTESIAN_POINT('',(-6.35,232.5,152.875));
#31549=CARTESIAN_POINT('Origin',(-6.35,277.5,25.8749999999999));
#31550=CARTESIAN_POINT('',(6.35,277.5,25.8749999999999));
#31551=CARTESIAN_POINT('',(6.35,277.5,25.8749999999999));
#31552=CARTESIAN_POINT('',(-6.35,277.5,25.8749999999999));
#31553=CARTESIAN_POINT('',(-6.35,277.5,25.8749999999999));
#31554=CARTESIAN_POINT('',(-6.35,277.5,25.8749999999999));
#31555=CARTESIAN_POINT('Origin',(-6.35,267.5,15.875));
#31556=CARTESIAN_POINT('',(6.35,267.5,15.875));
#31557=CARTESIAN_POINT('',(6.35,267.5,15.875));
#31558=CARTESIAN_POINT('',(-6.35,267.5,15.875));
#31559=CARTESIAN_POINT('',(-6.35,267.5,15.875));
#31560=CARTESIAN_POINT('',(-6.35,267.5,15.875));
#31561=CARTESIAN_POINT('Origin',(-6.35,217.5,15.875));
#31562=CARTESIAN_POINT('',(6.35,217.5,15.875));
#31563=CARTESIAN_POINT('',(6.35,217.5,15.875));
#31564=CARTESIAN_POINT('',(-6.35,217.5,15.875));
#31565=CARTESIAN_POINT('',(-6.35,217.5,15.875));
#31566=CARTESIAN_POINT('',(-6.35,217.5,15.875));
#31567=CARTESIAN_POINT('Origin',(-6.35,207.5,25.875));
#31568=CARTESIAN_POINT('',(6.35,207.5,25.875));
#31569=CARTESIAN_POINT('',(6.35,207.5,25.875));
#31570=CARTESIAN_POINT('',(-6.35,207.5,25.875));
#31571=CARTESIAN_POINT('',(-6.35,207.5,25.875));
#31572=CARTESIAN_POINT('',(-6.35,207.5,25.875));
#31573=CARTESIAN_POINT('Origin',(-6.35,207.5,152.875));
#31574=CARTESIAN_POINT('',(6.35,207.5,152.875));
#31575=CARTESIAN_POINT('',(6.35,207.5,152.875));
#31576=CARTESIAN_POINT('',(-6.35,207.5,152.875));
#31577=CARTESIAN_POINT('',(-6.35,207.5,152.875));
#31578=CARTESIAN_POINT('',(-6.35,207.5,152.875));
#31579=CARTESIAN_POINT('Origin',(-6.35,232.5,152.875));
#31580=CARTESIAN_POINT('',(6.35,232.5,152.875));
#31581=CARTESIAN_POINT('',(-6.35,232.5,152.875));
#31582=CARTESIAN_POINT('Origin',(-6.35,0.,0.));
#31583=CARTESIAN_POINT('Origin',(6.35,0.,0.));
#31584=CARTESIAN_POINT('Origin',(170.65,277.5,66.6749999999998));
#31585=CARTESIAN_POINT('',(183.35,277.5,66.6749999999998));
#31586=CARTESIAN_POINT('',(183.35,232.5,152.875));
#31587=CARTESIAN_POINT('',(183.35,277.5,66.6749999999998));
#31588=CARTESIAN_POINT('',(170.65,277.5,66.6749999999998));
#31589=CARTESIAN_POINT('',(170.65,277.5,66.6749999999998));
#31590=CARTESIAN_POINT('',(170.65,232.5,152.875));
#31591=CARTESIAN_POINT('',(170.65,277.5,66.6749999999998));
#31592=CARTESIAN_POINT('',(170.65,232.5,152.875));
#31593=CARTESIAN_POINT('Origin',(170.65,277.5,25.8749999999999));
#31594=CARTESIAN_POINT('',(183.35,277.5,25.8749999999999));
#31595=CARTESIAN_POINT('',(183.35,277.5,25.8749999999999));
#31596=CARTESIAN_POINT('',(170.65,277.5,25.8749999999999));
#31597=CARTESIAN_POINT('',(170.65,277.5,25.8749999999999));
#31598=CARTESIAN_POINT('',(170.65,277.5,25.8749999999999));
#31599=CARTESIAN_POINT('Origin',(170.65,267.5,15.875));
#31600=CARTESIAN_POINT('',(183.35,267.5,15.875));
#31601=CARTESIAN_POINT('',(183.35,267.5,15.875));
#31602=CARTESIAN_POINT('',(170.65,267.5,15.875));
#31603=CARTESIAN_POINT('',(170.65,267.5,15.875));
#31604=CARTESIAN_POINT('',(170.65,267.5,15.875));
#31605=CARTESIAN_POINT('Origin',(170.65,217.5,15.875));
#31606=CARTESIAN_POINT('',(183.35,217.5,15.875));
#31607=CARTESIAN_POINT('',(183.35,217.5,15.875));
#31608=CARTESIAN_POINT('',(170.65,217.5,15.875));
#31609=CARTESIAN_POINT('',(170.65,217.5,15.875));
#31610=CARTESIAN_POINT('',(170.65,217.5,15.875));
#31611=CARTESIAN_POINT('Origin',(170.65,207.5,25.875));
#31612=CARTESIAN_POINT('',(183.35,207.5,25.875));
#31613=CARTESIAN_POINT('',(183.35,207.5,25.875));
#31614=CARTESIAN_POINT('',(170.65,207.5,25.875));
#31615=CARTESIAN_POINT('',(170.65,207.5,25.875));
#31616=CARTESIAN_POINT('',(170.65,207.5,25.875));
#31617=CARTESIAN_POINT('Origin',(170.65,207.5,152.875));
#31618=CARTESIAN_POINT('',(183.35,207.5,152.875));
#31619=CARTESIAN_POINT('',(183.35,207.5,152.875));
#31620=CARTESIAN_POINT('',(170.65,207.5,152.875));
#31621=CARTESIAN_POINT('',(170.65,207.5,152.875));
#31622=CARTESIAN_POINT('',(170.65,207.5,152.875));
#31623=CARTESIAN_POINT('Origin',(170.65,232.5,152.875));
#31624=CARTESIAN_POINT('',(183.35,232.5,152.875));
#31625=CARTESIAN_POINT('',(170.65,232.5,152.875));
#31626=CARTESIAN_POINT('Origin',(170.65,0.,0.));
#31627=CARTESIAN_POINT('Origin',(183.35,0.,0.));
#31628=CARTESIAN_POINT('Origin',(347.65,277.5,66.6749999999998));
#31629=CARTESIAN_POINT('',(360.35,277.5,66.6749999999998));
#31630=CARTESIAN_POINT('',(360.35,232.5,152.875));
#31631=CARTESIAN_POINT('',(360.35,277.5,66.6749999999998));
#31632=CARTESIAN_POINT('',(347.65,277.5,66.6749999999998));
#31633=CARTESIAN_POINT('',(347.65,277.5,66.6749999999998));
#31634=CARTESIAN_POINT('',(347.65,232.5,152.875));
#31635=CARTESIAN_POINT('',(347.65,277.5,66.6749999999998));
#31636=CARTESIAN_POINT('',(347.65,232.5,152.875));
#31637=CARTESIAN_POINT('Origin',(347.65,277.5,25.8749999999999));
#31638=CARTESIAN_POINT('',(360.35,277.5,25.8749999999999));
#31639=CARTESIAN_POINT('',(360.35,277.5,25.8749999999999));
#31640=CARTESIAN_POINT('',(347.65,277.5,25.8749999999999));
#31641=CARTESIAN_POINT('',(347.65,277.5,25.8749999999999));
#31642=CARTESIAN_POINT('',(347.65,277.5,25.8749999999999));
#31643=CARTESIAN_POINT('Origin',(347.65,267.5,15.875));
#31644=CARTESIAN_POINT('',(360.35,267.5,15.875));
#31645=CARTESIAN_POINT('',(360.35,267.5,15.875));
#31646=CARTESIAN_POINT('',(347.65,267.5,15.875));
#31647=CARTESIAN_POINT('',(347.65,267.5,15.875));
#31648=CARTESIAN_POINT('',(347.65,267.5,15.875));
#31649=CARTESIAN_POINT('Origin',(347.65,217.5,15.875));
#31650=CARTESIAN_POINT('',(360.35,217.5,15.875));
#31651=CARTESIAN_POINT('',(360.35,217.5,15.875));
#31652=CARTESIAN_POINT('',(347.65,217.5,15.875));
#31653=CARTESIAN_POINT('',(347.65,217.5,15.875));
#31654=CARTESIAN_POINT('',(347.65,217.5,15.875));
#31655=CARTESIAN_POINT('Origin',(347.65,207.5,25.875));
#31656=CARTESIAN_POINT('',(360.35,207.5,25.875));
#31657=CARTESIAN_POINT('',(360.35,207.5,25.875));
#31658=CARTESIAN_POINT('',(347.65,207.5,25.875));
#31659=CARTESIAN_POINT('',(347.65,207.5,25.875));
#31660=CARTESIAN_POINT('',(347.65,207.5,25.875));
#31661=CARTESIAN_POINT('Origin',(347.65,207.5,152.875));
#31662=CARTESIAN_POINT('',(360.35,207.5,152.875));
#31663=CARTESIAN_POINT('',(360.35,207.5,152.875));
#31664=CARTESIAN_POINT('',(347.65,207.5,152.875));
#31665=CARTESIAN_POINT('',(347.65,207.5,152.875));
#31666=CARTESIAN_POINT('',(347.65,207.5,152.875));
#31667=CARTESIAN_POINT('Origin',(347.65,232.5,152.875));
#31668=CARTESIAN_POINT('',(360.35,232.5,152.875));
#31669=CARTESIAN_POINT('',(347.65,232.5,152.875));
#31670=CARTESIAN_POINT('Origin',(347.65,0.,0.));
#31671=CARTESIAN_POINT('Origin',(360.35,0.,0.));
#31672=CARTESIAN_POINT('Origin',(-170.65,277.5,66.6749999999998));
#31673=CARTESIAN_POINT('',(-183.35,277.5,66.6749999999998));
#31674=CARTESIAN_POINT('',(-183.35,232.5,152.875));
#31675=CARTESIAN_POINT('',(-183.35,277.5,66.6749999999998));
#31676=CARTESIAN_POINT('',(-170.65,232.5,152.875));
#31677=CARTESIAN_POINT('',(-170.65,232.5,152.875));
#31678=CARTESIAN_POINT('',(-170.65,277.5,66.6749999999998));
#31679=CARTESIAN_POINT('',(-170.65,277.5,66.6749999999998));
#31680=CARTESIAN_POINT('',(-170.65,277.5,66.6749999999998));
#31681=CARTESIAN_POINT('Origin',(-170.65,277.5,25.8749999999999));
#31682=CARTESIAN_POINT('',(-183.35,277.5,25.8749999999999));
#31683=CARTESIAN_POINT('',(-183.35,277.5,25.8749999999999));
#31684=CARTESIAN_POINT('',(-170.65,277.5,25.8749999999999));
#31685=CARTESIAN_POINT('',(-170.65,277.5,25.8749999999999));
#31686=CARTESIAN_POINT('',(-170.65,277.5,25.8749999999999));
#31687=CARTESIAN_POINT('Origin',(-170.65,267.5,15.875));
#31688=CARTESIAN_POINT('',(-183.35,267.5,15.875));
#31689=CARTESIAN_POINT('',(-183.35,267.5,15.875));
#31690=CARTESIAN_POINT('',(-170.65,267.5,15.875));
#31691=CARTESIAN_POINT('',(-170.65,267.5,15.875));
#31692=CARTESIAN_POINT('',(-170.65,267.5,15.875));
#31693=CARTESIAN_POINT('Origin',(-170.65,217.5,15.875));
#31694=CARTESIAN_POINT('',(-183.35,217.5,15.875));
#31695=CARTESIAN_POINT('',(-183.35,217.5,15.875));
#31696=CARTESIAN_POINT('',(-170.65,217.5,15.875));
#31697=CARTESIAN_POINT('',(-170.65,217.5,15.875));
#31698=CARTESIAN_POINT('',(-170.65,217.5,15.875));
#31699=CARTESIAN_POINT('Origin',(-170.65,207.5,25.875));
#31700=CARTESIAN_POINT('',(-183.35,207.5,25.875));
#31701=CARTESIAN_POINT('',(-183.35,207.5,25.875));
#31702=CARTESIAN_POINT('',(-170.65,207.5,25.875));
#31703=CARTESIAN_POINT('',(-170.65,207.5,25.875));
#31704=CARTESIAN_POINT('',(-170.65,207.5,25.875));
#31705=CARTESIAN_POINT('Origin',(-170.65,207.5,152.875));
#31706=CARTESIAN_POINT('',(-183.35,207.5,152.875));
#31707=CARTESIAN_POINT('',(-183.35,207.5,152.875));
#31708=CARTESIAN_POINT('',(-170.65,207.5,152.875));
#31709=CARTESIAN_POINT('',(-170.65,207.5,152.875));
#31710=CARTESIAN_POINT('',(-170.65,207.5,152.875));
#31711=CARTESIAN_POINT('Origin',(-170.65,232.5,152.875));
#31712=CARTESIAN_POINT('',(-183.35,232.5,152.875));
#31713=CARTESIAN_POINT('',(-170.65,232.5,152.875));
#31714=CARTESIAN_POINT('Origin',(-170.65,0.,0.));
#31715=CARTESIAN_POINT('Origin',(-183.35,0.,0.));
#31716=CARTESIAN_POINT('Origin',(-347.65,277.5,66.6749999999998));
#31717=CARTESIAN_POINT('',(-360.35,277.5,66.6749999999998));
#31718=CARTESIAN_POINT('',(-360.35,232.5,152.875));
#31719=CARTESIAN_POINT('',(-360.35,277.5,66.6749999999998));
#31720=CARTESIAN_POINT('',(-347.65,232.5,152.875));
#31721=CARTESIAN_POINT('',(-347.65,232.5,152.875));
#31722=CARTESIAN_POINT('',(-347.65,277.5,66.6749999999998));
#31723=CARTESIAN_POINT('',(-347.65,277.5,66.6749999999998));
#31724=CARTESIAN_POINT('',(-347.65,277.5,66.6749999999998));
#31725=CARTESIAN_POINT('Origin',(-347.65,277.5,25.8749999999999));
#31726=CARTESIAN_POINT('',(-360.35,277.5,25.8749999999999));
#31727=CARTESIAN_POINT('',(-360.35,277.5,25.8749999999999));
#31728=CARTESIAN_POINT('',(-347.65,277.5,25.8749999999999));
#31729=CARTESIAN_POINT('',(-347.65,277.5,25.8749999999999));
#31730=CARTESIAN_POINT('',(-347.65,277.5,25.8749999999999));
#31731=CARTESIAN_POINT('Origin',(-347.65,267.5,15.875));
#31732=CARTESIAN_POINT('',(-360.35,267.5,15.875));
#31733=CARTESIAN_POINT('',(-360.35,267.5,15.875));
#31734=CARTESIAN_POINT('',(-347.65,267.5,15.875));
#31735=CARTESIAN_POINT('',(-347.65,267.5,15.875));
#31736=CARTESIAN_POINT('',(-347.65,267.5,15.875));
#31737=CARTESIAN_POINT('Origin',(-347.65,217.5,15.875));
#31738=CARTESIAN_POINT('',(-360.35,217.5,15.875));
#31739=CARTESIAN_POINT('',(-360.35,217.5,15.875));
#31740=CARTESIAN_POINT('',(-347.65,217.5,15.875));
#31741=CARTESIAN_POINT('',(-347.65,217.5,15.875));
#31742=CARTESIAN_POINT('',(-347.65,217.5,15.875));
#31743=CARTESIAN_POINT('Origin',(-347.65,207.5,25.875));
#31744=CARTESIAN_POINT('',(-360.35,207.5,25.875));
#31745=CARTESIAN_POINT('',(-360.35,207.5,25.875));
#31746=CARTESIAN_POINT('',(-347.65,207.5,25.875));
#31747=CARTESIAN_POINT('',(-347.65,207.5,25.875));
#31748=CARTESIAN_POINT('',(-347.65,207.5,25.875));
#31749=CARTESIAN_POINT('Origin',(-347.65,207.5,152.875));
#31750=CARTESIAN_POINT('',(-360.35,207.5,152.875));
#31751=CARTESIAN_POINT('',(-360.35,207.5,152.875));
#31752=CARTESIAN_POINT('',(-347.65,207.5,152.875));
#31753=CARTESIAN_POINT('',(-347.65,207.5,152.875));
#31754=CARTESIAN_POINT('',(-347.65,207.5,152.875));
#31755=CARTESIAN_POINT('Origin',(-347.65,232.5,152.875));
#31756=CARTESIAN_POINT('',(-360.35,232.5,152.875));
#31757=CARTESIAN_POINT('',(-347.65,232.5,152.875));
#31758=CARTESIAN_POINT('Origin',(-347.65,0.,0.));
#31759=CARTESIAN_POINT('Origin',(-360.35,0.,0.));
#31760=CARTESIAN_POINT('Origin',(-463.699999999999,277.5,-120.509999999995));
#31761=CARTESIAN_POINT('',(-463.699999999999,277.5,-107.809999999995));
#31762=CARTESIAN_POINT('',(-566.699999999999,232.5,-107.809999999995));
#31763=CARTESIAN_POINT('',(-463.699999999999,277.5,-107.809999999995));
#31764=CARTESIAN_POINT('',(-463.699999999999,277.5,-120.509999999995));
#31765=CARTESIAN_POINT('',(-463.699999999999,277.5,-120.509999999995));
#31766=CARTESIAN_POINT('',(-566.699999999999,232.5,-120.509999999995));
#31767=CARTESIAN_POINT('',(-463.699999999999,277.5,-120.509999999995));
#31768=CARTESIAN_POINT('',(-566.699999999999,232.5,-120.509999999995));
#31769=CARTESIAN_POINT('Origin',(-566.699999999999,232.5,-120.509999999995));
#31770=CARTESIAN_POINT('',(-566.699999999999,207.5,-107.809999999995));
#31771=CARTESIAN_POINT('',(-566.699999999999,232.5,-107.809999999995));
#31772=CARTESIAN_POINT('',(-566.699999999999,207.5,-120.509999999995));
#31773=CARTESIAN_POINT('',(-566.699999999999,232.5,-120.509999999995));
#31774=CARTESIAN_POINT('',(-566.699999999999,207.5,-120.509999999995));
#31775=CARTESIAN_POINT('Origin',(-566.699999999999,207.5,-120.509999999995));
#31776=CARTESIAN_POINT('',(-422.699999999999,207.5,-107.809999999995));
#31777=CARTESIAN_POINT('',(-566.699999999999,207.5,-107.809999999995));
#31778=CARTESIAN_POINT('',(-422.699999999999,207.5,-120.509999999995));
#31779=CARTESIAN_POINT('',(-566.699999999999,207.5,-120.509999999995));
#31780=CARTESIAN_POINT('',(-422.699999999999,207.5,-120.509999999995));
#31781=CARTESIAN_POINT('Origin',(-422.699999999999,207.5,-120.509999999995));
#31782=CARTESIAN_POINT('',(-412.699999999999,217.5,-107.809999999995));
#31783=CARTESIAN_POINT('',(-422.699999999999,207.5,-107.809999999995));
#31784=CARTESIAN_POINT('',(-412.699999999999,217.5,-120.509999999995));
#31785=CARTESIAN_POINT('',(-422.699999999999,207.5,-120.509999999995));
#31786=CARTESIAN_POINT('',(-412.699999999999,217.5,-120.509999999995));
#31787=CARTESIAN_POINT('Origin',(-412.699999999999,217.5,-120.509999999995));
#31788=CARTESIAN_POINT('',(-412.699999999999,267.5,-107.809999999995));
#31789=CARTESIAN_POINT('',(-412.699999999999,217.5,-107.809999999995));
#31790=CARTESIAN_POINT('',(-412.699999999999,267.5,-120.509999999995));
#31791=CARTESIAN_POINT('',(-412.699999999999,217.5,-120.509999999995));
#31792=CARTESIAN_POINT('',(-412.699999999999,267.5,-120.509999999995));
#31793=CARTESIAN_POINT('Origin',(-412.699999999999,267.5,-120.509999999995));
#31794=CARTESIAN_POINT('',(-422.699999999999,277.5,-107.809999999995));
#31795=CARTESIAN_POINT('',(-412.699999999999,267.5,-107.809999999995));
#31796=CARTESIAN_POINT('',(-422.699999999999,277.5,-120.509999999995));
#31797=CARTESIAN_POINT('',(-412.699999999999,267.5,-120.509999999995));
#31798=CARTESIAN_POINT('',(-422.699999999999,277.5,-120.509999999995));
#31799=CARTESIAN_POINT('Origin',(-422.699999999999,277.5,-120.509999999995));
#31800=CARTESIAN_POINT('',(-422.699999999999,277.5,-107.809999999995));
#31801=CARTESIAN_POINT('',(-422.699999999999,277.5,-120.509999999995));
#31802=CARTESIAN_POINT('Origin',(-2.49977721536069E-12,0.,-120.509999999995));
#31803=CARTESIAN_POINT('Origin',(-2.49977721536069E-12,0.,-107.809999999995));
#31804=CARTESIAN_POINT('Origin',(-463.699999999997,277.5,-240.509999999995));
#31805=CARTESIAN_POINT('',(-463.699999999997,277.5,-227.809999999995));
#31806=CARTESIAN_POINT('',(-566.699999999997,232.5,-227.809999999995));
#31807=CARTESIAN_POINT('',(-463.699999999997,277.5,-227.809999999995));
#31808=CARTESIAN_POINT('',(-463.699999999997,277.5,-240.509999999995));
#31809=CARTESIAN_POINT('',(-463.699999999997,277.5,-240.509999999995));
#31810=CARTESIAN_POINT('',(-566.699999999997,232.5,-240.509999999995));
#31811=CARTESIAN_POINT('',(-463.699999999997,277.5,-240.509999999995));
#31812=CARTESIAN_POINT('',(-566.699999999997,232.5,-240.509999999995));
#31813=CARTESIAN_POINT('Origin',(-566.699999999997,232.5,-240.509999999995));
#31814=CARTESIAN_POINT('',(-566.699999999997,207.5,-227.809999999995));
#31815=CARTESIAN_POINT('',(-566.699999999997,232.5,-227.809999999995));
#31816=CARTESIAN_POINT('',(-566.699999999997,207.5,-240.509999999995));
#31817=CARTESIAN_POINT('',(-566.699999999997,232.5,-240.509999999995));
#31818=CARTESIAN_POINT('',(-566.699999999997,207.5,-240.509999999995));
#31819=CARTESIAN_POINT('Origin',(-566.699999999997,207.5,-240.509999999995));
#31820=CARTESIAN_POINT('',(-422.699999999998,207.5,-227.809999999995));
#31821=CARTESIAN_POINT('',(-566.699999999997,207.5,-227.809999999995));
#31822=CARTESIAN_POINT('',(-422.699999999998,207.5,-240.509999999995));
#31823=CARTESIAN_POINT('',(-566.699999999997,207.5,-240.509999999995));
#31824=CARTESIAN_POINT('',(-422.699999999998,207.5,-240.509999999995));
#31825=CARTESIAN_POINT('Origin',(-422.699999999998,207.5,-240.509999999995));
#31826=CARTESIAN_POINT('',(-412.699999999998,217.5,-227.809999999995));
#31827=CARTESIAN_POINT('',(-422.699999999998,207.5,-227.809999999995));
#31828=CARTESIAN_POINT('',(-412.699999999998,217.5,-240.509999999995));
#31829=CARTESIAN_POINT('',(-422.699999999998,207.5,-240.509999999995));
#31830=CARTESIAN_POINT('',(-412.699999999998,217.5,-240.509999999995));
#31831=CARTESIAN_POINT('Origin',(-412.699999999998,217.5,-240.509999999995));
#31832=CARTESIAN_POINT('',(-412.699999999998,267.5,-227.809999999995));
#31833=CARTESIAN_POINT('',(-412.699999999998,217.5,-227.809999999995));
#31834=CARTESIAN_POINT('',(-412.699999999998,267.5,-240.509999999995));
#31835=CARTESIAN_POINT('',(-412.699999999998,217.5,-240.509999999995));
#31836=CARTESIAN_POINT('',(-412.699999999998,267.5,-240.509999999995));
#31837=CARTESIAN_POINT('Origin',(-412.699999999998,267.5,-240.509999999995));
#31838=CARTESIAN_POINT('',(-422.699999999998,277.5,-227.809999999995));
#31839=CARTESIAN_POINT('',(-412.699999999998,267.5,-227.809999999995));
#31840=CARTESIAN_POINT('',(-422.699999999998,277.5,-240.509999999995));
#31841=CARTESIAN_POINT('',(-412.699999999998,267.5,-240.509999999995));
#31842=CARTESIAN_POINT('',(-422.699999999998,277.5,-240.509999999995));
#31843=CARTESIAN_POINT('Origin',(-422.699999999998,277.5,-240.509999999995));
#31844=CARTESIAN_POINT('',(-422.699999999998,277.5,-227.809999999995));
#31845=CARTESIAN_POINT('',(-422.699999999998,277.5,-240.509999999995));
#31846=CARTESIAN_POINT('Origin',(-1.24988860768035E-12,0.,-240.509999999995));
#31847=CARTESIAN_POINT('Origin',(-1.24988860768035E-12,0.,-227.809999999995));
#31848=CARTESIAN_POINT('Origin',(-463.699999999996,277.5,-360.509999999995));
#31849=CARTESIAN_POINT('',(-463.699999999996,277.5,-347.809999999995));
#31850=CARTESIAN_POINT('',(-566.699999999996,232.5,-347.809999999995));
#31851=CARTESIAN_POINT('',(-463.699999999996,277.5,-347.809999999995));
#31852=CARTESIAN_POINT('',(-463.699999999996,277.5,-360.509999999995));
#31853=CARTESIAN_POINT('',(-463.699999999996,277.5,-360.509999999995));
#31854=CARTESIAN_POINT('',(-566.699999999996,232.5,-360.509999999995));
#31855=CARTESIAN_POINT('',(-463.699999999996,277.5,-360.509999999995));
#31856=CARTESIAN_POINT('',(-566.699999999996,232.5,-360.509999999995));
#31857=CARTESIAN_POINT('Origin',(-566.699999999996,232.5,-360.509999999995));
#31858=CARTESIAN_POINT('',(-566.699999999996,207.5,-347.809999999995));
#31859=CARTESIAN_POINT('',(-566.699999999996,232.5,-347.809999999995));
#31860=CARTESIAN_POINT('',(-566.699999999996,207.5,-360.509999999995));
#31861=CARTESIAN_POINT('',(-566.699999999996,232.5,-360.509999999995));
#31862=CARTESIAN_POINT('',(-566.699999999996,207.5,-360.509999999995));
#31863=CARTESIAN_POINT('Origin',(-566.699999999996,207.5,-360.509999999995));
#31864=CARTESIAN_POINT('',(-422.699999999996,207.5,-347.809999999995));
#31865=CARTESIAN_POINT('',(-566.699999999996,207.5,-347.809999999995));
#31866=CARTESIAN_POINT('',(-422.699999999996,207.5,-360.509999999995));
#31867=CARTESIAN_POINT('',(-566.699999999996,207.5,-360.509999999995));
#31868=CARTESIAN_POINT('',(-422.699999999996,207.5,-360.509999999995));
#31869=CARTESIAN_POINT('Origin',(-422.699999999996,207.5,-360.509999999995));
#31870=CARTESIAN_POINT('',(-412.699999999996,217.5,-347.809999999995));
#31871=CARTESIAN_POINT('',(-422.699999999996,207.5,-347.809999999995));
#31872=CARTESIAN_POINT('',(-412.699999999996,217.5,-360.509999999995));
#31873=CARTESIAN_POINT('',(-422.699999999996,207.5,-360.509999999995));
#31874=CARTESIAN_POINT('',(-412.699999999996,217.5,-360.509999999995));
#31875=CARTESIAN_POINT('Origin',(-412.699999999996,217.5,-360.509999999995));
#31876=CARTESIAN_POINT('',(-412.699999999996,267.5,-347.809999999995));
#31877=CARTESIAN_POINT('',(-412.699999999996,217.5,-347.809999999995));
#31878=CARTESIAN_POINT('',(-412.699999999996,267.5,-360.509999999995));
#31879=CARTESIAN_POINT('',(-412.699999999996,217.5,-360.509999999995));
#31880=CARTESIAN_POINT('',(-412.699999999996,267.5,-360.509999999995));
#31881=CARTESIAN_POINT('Origin',(-412.699999999996,267.5,-360.509999999995));
#31882=CARTESIAN_POINT('',(-422.699999999996,277.5,-347.809999999995));
#31883=CARTESIAN_POINT('',(-412.699999999996,267.5,-347.809999999995));
#31884=CARTESIAN_POINT('',(-422.699999999996,277.5,-360.509999999995));
#31885=CARTESIAN_POINT('',(-412.699999999996,267.5,-360.509999999995));
#31886=CARTESIAN_POINT('',(-422.699999999996,277.5,-360.509999999995));
#31887=CARTESIAN_POINT('Origin',(-422.699999999996,277.5,-360.509999999995));
#31888=CARTESIAN_POINT('',(-422.699999999996,277.5,-347.809999999995));
#31889=CARTESIAN_POINT('',(-422.699999999996,277.5,-360.509999999995));
#31890=CARTESIAN_POINT('Origin',(0.,0.,-360.509999999995));
#31891=CARTESIAN_POINT('Origin',(0.,0.,-347.809999999995));
#31892=CARTESIAN_POINT('Origin',(-579.199999999996,191.625,-54.1249999999996));
#31893=CARTESIAN_POINT('',(-579.199999999996,191.625,-63.1249999999996));
#31894=CARTESIAN_POINT('Origin',(-579.199999999996,191.625,-54.1249999999996));
#31895=CARTESIAN_POINT('',(-579.199999999996,207.5,-63.1249999999996));
#31896=CARTESIAN_POINT('',(-579.199999999996,191.625,-63.1249999999996));
#31897=CARTESIAN_POINT('Origin',(-579.199999999996,207.5,-54.1249999999996));
#31898=CARTESIAN_POINT('Origin',(-579.199999999998,191.625,-174.125));
#31899=CARTESIAN_POINT('',(-579.199999999998,191.625,-183.125));
#31900=CARTESIAN_POINT('Origin',(-579.199999999998,191.625,-174.125));
#31901=CARTESIAN_POINT('',(-579.199999999998,207.5,-183.125));
#31902=CARTESIAN_POINT('',(-579.199999999998,191.625,-183.125));
#31903=CARTESIAN_POINT('Origin',(-579.199999999998,207.5,-174.125));
#31904=CARTESIAN_POINT('Origin',(-579.199999999999,191.625,-294.125));
#31905=CARTESIAN_POINT('',(-579.199999999999,191.625,-303.125));
#31906=CARTESIAN_POINT('Origin',(-579.199999999999,191.625,-294.125));
#31907=CARTESIAN_POINT('',(-579.199999999999,207.5,-303.125));
#31908=CARTESIAN_POINT('',(-579.199999999999,191.625,-303.125));
#31909=CARTESIAN_POINT('Origin',(-579.199999999999,207.5,-294.125));
#31910=CARTESIAN_POINT('Origin',(-579.2,191.625,-414.125));
#31911=CARTESIAN_POINT('',(-579.2,191.625,-423.125));
#31912=CARTESIAN_POINT('Origin',(-579.2,191.625,-414.125));
#31913=CARTESIAN_POINT('',(-579.2,207.5,-423.125));
#31914=CARTESIAN_POINT('',(-579.2,191.625,-423.125));
#31915=CARTESIAN_POINT('Origin',(-579.2,207.5,-414.125));
#31916=CARTESIAN_POINT('Origin',(0.,191.625,0.));
#31917=CARTESIAN_POINT('',(-412.7,191.625,15.8749999999999));
#31918=CARTESIAN_POINT('',(-412.7,191.625,-453.125));
#31919=CARTESIAN_POINT('',(-412.7,191.625,-453.125));
#31920=CARTESIAN_POINT('',(-595.7,191.625,15.8749999999999));
#31921=CARTESIAN_POINT('',(-412.7,191.625,15.8749999999999));
#31922=CARTESIAN_POINT('',(-595.7,191.625,-453.125));
#31923=CARTESIAN_POINT('',(-595.7,191.625,-453.125));
#31924=CARTESIAN_POINT('',(-412.7,191.625,-453.125));
#31925=CARTESIAN_POINT('Origin',(0.,207.5,0.));
#31926=CARTESIAN_POINT('',(-412.7,207.5,15.8749999999999));
#31927=CARTESIAN_POINT('',(-412.7,207.5,-453.125));
#31928=CARTESIAN_POINT('',(-412.7,207.5,-453.125));
#31929=CARTESIAN_POINT('',(-595.7,207.5,-453.125));
#31930=CARTESIAN_POINT('',(-412.7,207.5,-453.125));
#31931=CARTESIAN_POINT('',(-595.7,207.5,15.8749999999999));
#31932=CARTESIAN_POINT('',(-595.7,207.5,-453.125));
#31933=CARTESIAN_POINT('',(-412.7,207.5,15.8749999999999));
#31934=CARTESIAN_POINT('Origin',(-412.7,191.625,-453.125));
#31935=CARTESIAN_POINT('',(-412.7,191.625,15.8749999999999));
#31936=CARTESIAN_POINT('',(-412.7,191.625,-453.125));
#31937=CARTESIAN_POINT('Origin',(-412.7,191.625,-453.125));
#31938=CARTESIAN_POINT('',(-595.7,191.625,-453.125));
#31939=CARTESIAN_POINT('Origin',(-595.7,191.625,-453.125));
#31940=CARTESIAN_POINT('',(-595.7,191.625,15.8749999999999));
#31941=CARTESIAN_POINT('Origin',(-412.7,191.625,15.8749999999999));
#31942=CARTESIAN_POINT('Origin',(-374.6,-56.6030981210581,-692.742399072376));
#31943=CARTESIAN_POINT('',(-374.6,-63.1029956157432,-704.000788502422));
#31944=CARTESIAN_POINT('',(-374.6,-400.854678517142,-509.003863661867));
#31945=CARTESIAN_POINT('',(-374.6,-63.1029956157432,-704.000788502422));
#31946=CARTESIAN_POINT('',(-374.6,-394.354781022457,-497.74547423182));
#31947=CARTESIAN_POINT('',(-374.6,-394.354781022457,-497.74547423182));
#31948=CARTESIAN_POINT('',(-374.6,-56.6030981210581,-692.742399072376));
#31949=CARTESIAN_POINT('',(-374.6,-56.6030981210581,-692.742399072376));
#31950=CARTESIAN_POINT('',(-374.6,-56.6030981210581,-692.742399072376));
#31951=CARTESIAN_POINT('Origin',(-374.6,-394.354781022457,-497.74547423182));
#31952=CARTESIAN_POINT('',(-194.8,-400.854678517142,-509.003863661867));
#31953=CARTESIAN_POINT('',(-374.6,-400.854678517142,-509.003863661867));
#31954=CARTESIAN_POINT('',(-194.8,-394.354781022457,-497.74547423182));
#31955=CARTESIAN_POINT('',(-194.8,-394.354781022457,-497.74547423182));
#31956=CARTESIAN_POINT('',(-374.6,-394.354781022457,-497.74547423182));
#31957=CARTESIAN_POINT('Origin',(-194.8,-56.6030981210581,-692.742399072376));
#31958=CARTESIAN_POINT('',(-194.8,-63.1029956157432,-704.000788502422));
#31959=CARTESIAN_POINT('',(-194.8,-63.1029956157432,-704.000788502422));
#31960=CARTESIAN_POINT('',(-194.8,-56.6030981210581,-692.742399072376));
#31961=CARTESIAN_POINT('',(-194.8,-56.6030981210581,-692.742399072376));
#31962=CARTESIAN_POINT('',(-194.8,-56.6030981210581,-692.742399072376));
#31963=CARTESIAN_POINT('Origin',(-374.6,-56.6030981210581,-692.742399072376));
#31964=CARTESIAN_POINT('',(-374.6,-63.1029956157432,-704.000788502422));
#31965=CARTESIAN_POINT('',(-374.6,-56.6030981210581,-692.742399072376));
#31966=CARTESIAN_POINT('Origin',(0.,-314.113432458224,-544.071864320163));
#31967=CARTESIAN_POINT('Origin',(0.,-320.613329952909,-555.33025375021));
#31968=CARTESIAN_POINT('Origin',(5.,-403.015080584031,-492.745553082062));
#31969=CARTESIAN_POINT('',(5.,-409.514978078716,-504.003942512109));
#31970=CARTESIAN_POINT('',(4.99999999999989,-526.609655925898,-436.400720229833));
#31971=CARTESIAN_POINT('',(5.,-409.514978078716,-504.003942512109));
#31972=CARTESIAN_POINT('',(4.99999999999989,-520.109758431213,-425.142330799786));
#31973=CARTESIAN_POINT('',(4.99999999999989,-520.109758431213,-425.142330799786));
#31974=CARTESIAN_POINT('',(5.,-403.015080584031,-492.745553082062));
#31975=CARTESIAN_POINT('',(5.,-403.015080584031,-492.745553082062));
#31976=CARTESIAN_POINT('',(5.,-403.015080584031,-492.745553082062));
#31977=CARTESIAN_POINT('Origin',(4.99999999999989,-520.109758431213,-425.142330799786));
#31978=CARTESIAN_POINT('',(374.6,-526.609655925898,-436.400720229833));
#31979=CARTESIAN_POINT('',(4.99999999999989,-526.609655925898,-436.400720229833));
#31980=CARTESIAN_POINT('',(374.6,-520.109758431213,-425.142330799786));
#31981=CARTESIAN_POINT('',(374.6,-520.109758431213,-425.142330799786));
#31982=CARTESIAN_POINT('',(4.99999999999989,-520.109758431213,-425.142330799786));
#31983=CARTESIAN_POINT('Origin',(374.6,-403.015080584031,-492.745553082062));
#31984=CARTESIAN_POINT('',(374.6,-409.514978078716,-504.003942512109));
#31985=CARTESIAN_POINT('',(374.6,-409.514978078716,-504.003942512109));
#31986=CARTESIAN_POINT('',(374.6,-403.015080584031,-492.745553082062));
#31987=CARTESIAN_POINT('',(374.6,-403.015080584031,-492.745553082062));
#31988=CARTESIAN_POINT('',(374.6,-403.015080584031,-492.745553082062));
#31989=CARTESIAN_POINT('Origin',(5.,-403.015080584031,-492.745553082062));
#31990=CARTESIAN_POINT('',(5.,-409.514978078716,-504.003942512109));
#31991=CARTESIAN_POINT('',(5.,-403.015080584031,-492.745553082062));
#31992=CARTESIAN_POINT('Origin',(0.,-314.113432458223,-544.071864320163));
#31993=CARTESIAN_POINT('Origin',(0.,-320.613329952908,-555.33025375021));
#31994=CARTESIAN_POINT('Origin',(-184.8,-56.6030981210581,-692.742399072376));
#31995=CARTESIAN_POINT('',(-184.8,-63.1029956157432,-704.000788502422));
#31996=CARTESIAN_POINT('',(-184.8,-400.854678517142,-509.003863661867));
#31997=CARTESIAN_POINT('',(-184.8,-63.1029956157432,-704.000788502422));
#31998=CARTESIAN_POINT('',(-184.8,-394.354781022457,-497.74547423182));
#31999=CARTESIAN_POINT('',(-184.8,-394.354781022457,-497.74547423182));
#32000=CARTESIAN_POINT('',(-184.8,-56.6030981210581,-692.742399072376));
#32001=CARTESIAN_POINT('',(-184.8,-56.6030981210581,-692.742399072376));
#32002=CARTESIAN_POINT('',(-184.8,-56.6030981210581,-692.742399072376));
#32003=CARTESIAN_POINT('Origin',(-184.8,-394.354781022457,-497.74547423182));
#32004=CARTESIAN_POINT('',(-4.99999999999998,-400.854678517142,-509.003863661867));
#32005=CARTESIAN_POINT('',(-184.8,-400.854678517142,-509.003863661867));
#32006=CARTESIAN_POINT('',(-4.99999999999998,-394.354781022457,-497.74547423182));
#32007=CARTESIAN_POINT('',(-4.99999999999998,-394.354781022457,-497.74547423182));
#32008=CARTESIAN_POINT('',(-184.8,-394.354781022457,-497.74547423182));
#32009=CARTESIAN_POINT('Origin',(-4.99999999999998,-56.6030981210581,-692.742399072376));
#32010=CARTESIAN_POINT('',(-4.99999999999998,-63.1029956157432,-704.000788502422));
#32011=CARTESIAN_POINT('',(-4.99999999999998,-63.1029956157432,-704.000788502422));
#32012=CARTESIAN_POINT('',(-4.99999999999998,-56.6030981210581,-692.742399072376));
#32013=CARTESIAN_POINT('',(-4.99999999999998,-56.6030981210581,-692.742399072376));
#32014=CARTESIAN_POINT('',(-4.99999999999998,-56.6030981210581,-692.742399072376));
#32015=CARTESIAN_POINT('Origin',(-184.8,-56.6030981210581,-692.742399072376));
#32016=CARTESIAN_POINT('',(-184.8,-63.1029956157432,-704.000788502422));
#32017=CARTESIAN_POINT('',(-184.8,-56.6030981210581,-692.742399072376));
#32018=CARTESIAN_POINT('Origin',(0.,-314.113432458224,-544.071864320163));
#32019=CARTESIAN_POINT('Origin',(0.,-320.613329952909,-555.33025375021));
#32020=CARTESIAN_POINT('Origin',(5.,-56.6030981210581,-692.742399072376));
#32021=CARTESIAN_POINT('',(5.,-63.1029956157432,-704.000788502422));
#32022=CARTESIAN_POINT('',(5.,-400.854678517142,-509.003863661867));
#32023=CARTESIAN_POINT('',(5.,-63.1029956157432,-704.000788502422));
#32024=CARTESIAN_POINT('',(5.,-394.354781022457,-497.74547423182));
#32025=CARTESIAN_POINT('',(5.,-394.354781022457,-497.74547423182));
#32026=CARTESIAN_POINT('',(5.,-56.6030981210581,-692.742399072376));
#32027=CARTESIAN_POINT('',(5.,-56.6030981210581,-692.742399072376));
#32028=CARTESIAN_POINT('',(5.,-56.6030981210581,-692.742399072376));
#32029=CARTESIAN_POINT('Origin',(5.,-394.354781022457,-497.74547423182));
#32030=CARTESIAN_POINT('',(184.8,-400.854678517142,-509.003863661867));
#32031=CARTESIAN_POINT('',(5.,-400.854678517142,-509.003863661867));
#32032=CARTESIAN_POINT('',(184.8,-394.354781022457,-497.74547423182));
#32033=CARTESIAN_POINT('',(184.8,-394.354781022457,-497.74547423182));
#32034=CARTESIAN_POINT('',(5.,-394.354781022457,-497.74547423182));
#32035=CARTESIAN_POINT('Origin',(184.8,-56.6030981210581,-692.742399072376));
#32036=CARTESIAN_POINT('',(184.8,-63.1029956157432,-704.000788502422));
#32037=CARTESIAN_POINT('',(184.8,-63.1029956157432,-704.000788502422));
#32038=CARTESIAN_POINT('',(184.8,-56.6030981210581,-692.742399072376));
#32039=CARTESIAN_POINT('',(184.8,-56.6030981210581,-692.742399072376));
#32040=CARTESIAN_POINT('',(184.8,-56.6030981210581,-692.742399072376));
#32041=CARTESIAN_POINT('Origin',(5.,-56.6030981210581,-692.742399072376));
#32042=CARTESIAN_POINT('',(5.,-63.1029956157432,-704.000788502422));
#32043=CARTESIAN_POINT('',(5.,-56.6030981210581,-692.742399072376));
#32044=CARTESIAN_POINT('Origin',(0.,-314.113432458224,-544.071864320163));
#32045=CARTESIAN_POINT('Origin',(0.,-320.613329952909,-555.33025375021));
#32046=CARTESIAN_POINT('Origin',(194.8,-56.6030981210581,-692.742399072376));
#32047=CARTESIAN_POINT('',(194.8,-63.1029956157432,-704.000788502422));
#32048=CARTESIAN_POINT('',(194.8,-400.854678517142,-509.003863661867));
#32049=CARTESIAN_POINT('',(194.8,-63.1029956157432,-704.000788502422));
#32050=CARTESIAN_POINT('',(194.8,-394.354781022457,-497.74547423182));
#32051=CARTESIAN_POINT('',(194.8,-394.354781022457,-497.74547423182));
#32052=CARTESIAN_POINT('',(194.8,-56.6030981210581,-692.742399072376));
#32053=CARTESIAN_POINT('',(194.8,-56.6030981210581,-692.742399072376));
#32054=CARTESIAN_POINT('',(194.8,-56.6030981210581,-692.742399072376));
#32055=CARTESIAN_POINT('Origin',(194.8,-394.354781022457,-497.74547423182));
#32056=CARTESIAN_POINT('',(374.6,-400.854678517142,-509.003863661867));
#32057=CARTESIAN_POINT('',(194.8,-400.854678517142,-509.003863661867));
#32058=CARTESIAN_POINT('',(374.6,-394.354781022457,-497.74547423182));
#32059=CARTESIAN_POINT('',(374.6,-394.354781022457,-497.74547423182));
#32060=CARTESIAN_POINT('',(194.8,-394.354781022457,-497.74547423182));
#32061=CARTESIAN_POINT('Origin',(374.6,-56.6030981210581,-692.742399072376));
#32062=CARTESIAN_POINT('',(374.6,-63.1029956157432,-704.000788502422));
#32063=CARTESIAN_POINT('',(374.6,-63.1029956157432,-704.000788502422));
#32064=CARTESIAN_POINT('',(374.6,-56.6030981210581,-692.742399072376));
#32065=CARTESIAN_POINT('',(374.6,-56.6030981210581,-692.742399072376));
#32066=CARTESIAN_POINT('',(374.6,-56.6030981210581,-692.742399072376));
#32067=CARTESIAN_POINT('Origin',(194.8,-56.6030981210581,-692.742399072376));
#32068=CARTESIAN_POINT('',(194.8,-63.1029956157432,-704.000788502422));
#32069=CARTESIAN_POINT('',(194.8,-56.6030981210581,-692.742399072376));
#32070=CARTESIAN_POINT('Origin',(0.,-314.113432458224,-544.071864320163));
#32071=CARTESIAN_POINT('Origin',(0.,-320.613329952909,-555.33025375021));
#32072=CARTESIAN_POINT('Origin',(-374.6,-403.015080584031,-492.745553082062));
#32073=CARTESIAN_POINT('',(-374.6,-409.514978078716,-504.003942512109));
#32074=CARTESIAN_POINT('',(-374.6,-526.609655925898,-436.400720229833));
#32075=CARTESIAN_POINT('',(-374.6,-409.514978078716,-504.003942512109));
#32076=CARTESIAN_POINT('',(-374.6,-520.109758431213,-425.142330799786));
#32077=CARTESIAN_POINT('',(-374.6,-520.109758431213,-425.142330799786));
#32078=CARTESIAN_POINT('',(-374.6,-403.015080584031,-492.745553082062));
#32079=CARTESIAN_POINT('',(-374.6,-403.015080584031,-492.745553082062));
#32080=CARTESIAN_POINT('',(-374.6,-403.015080584031,-492.745553082062));
#32081=CARTESIAN_POINT('Origin',(-374.6,-520.109758431213,-425.142330799786));
#32082=CARTESIAN_POINT('',(-5.00000000000006,-526.609655925898,-436.400720229833));
#32083=CARTESIAN_POINT('',(-374.6,-526.609655925898,-436.400720229833));
#32084=CARTESIAN_POINT('',(-5.00000000000006,-520.109758431213,-425.142330799786));
#32085=CARTESIAN_POINT('',(-5.00000000000006,-520.109758431213,-425.142330799786));
#32086=CARTESIAN_POINT('',(-374.6,-520.109758431213,-425.142330799786));
#32087=CARTESIAN_POINT('Origin',(-4.99999999999995,-403.015080584031,-492.745553082062));
#32088=CARTESIAN_POINT('',(-4.99999999999995,-409.514978078716,-504.003942512109));
#32089=CARTESIAN_POINT('',(-4.99999999999995,-409.514978078716,-504.003942512109));
#32090=CARTESIAN_POINT('',(-4.99999999999995,-403.015080584031,-492.745553082062));
#32091=CARTESIAN_POINT('',(-4.99999999999995,-403.015080584031,-492.745553082062));
#32092=CARTESIAN_POINT('',(-4.99999999999995,-403.015080584031,-492.745553082062));
#32093=CARTESIAN_POINT('Origin',(-374.6,-403.015080584031,-492.745553082062));
#32094=CARTESIAN_POINT('',(-374.6,-409.514978078716,-504.003942512109));
#32095=CARTESIAN_POINT('',(-374.6,-403.015080584031,-492.745553082062));
#32096=CARTESIAN_POINT('Origin',(0.,-314.113432458223,-544.071864320163));
#32097=CARTESIAN_POINT('Origin',(0.,-320.613329952908,-555.33025375021));
#32098=CARTESIAN_POINT('Origin',(368.830769230769,-528.770057992788,-420.142409650028));
#32099=CARTESIAN_POINT('',(368.830769230769,-535.269955487473,-431.400799080075));
#32100=CARTESIAN_POINT('',(-368.830769230769,-535.269955487473,-431.400799080075));
#32101=CARTESIAN_POINT('',(368.830769230769,-535.269955487473,-431.400799080075));
#32102=CARTESIAN_POINT('',(-368.830769230769,-528.770057992788,-420.142409650028));
#32103=CARTESIAN_POINT('',(-368.830769230769,-528.770057992788,-420.142409650028));
#32104=CARTESIAN_POINT('',(368.830769230769,-528.770057992788,-420.142409650028));
#32105=CARTESIAN_POINT('',(368.830769230769,-528.770057992788,-420.142409650028));
#32106=CARTESIAN_POINT('',(368.830769230769,-528.770057992788,-420.142409650028));
#32107=CARTESIAN_POINT('Origin',(-368.830769230769,-528.770057992788,-420.142409650028));
#32108=CARTESIAN_POINT('',(-201.637568622845,-786.246777154128,-286.502310312096));
#32109=CARTESIAN_POINT('',(-368.830769230769,-535.269955487473,-431.400799080075));
#32110=CARTESIAN_POINT('',(-201.637568622845,-779.746879659443,-275.243920882049));
#32111=CARTESIAN_POINT('',(-201.637568622845,-779.746879659443,-275.243920882049));
#32112=CARTESIAN_POINT('',(-368.830769230769,-528.770057992788,-420.142409650028));
#32113=CARTESIAN_POINT('Origin',(-201.637568622845,-779.746879659443,-275.243920882049));
#32114=CARTESIAN_POINT('',(201.637568622845,-786.246777154128,-286.502310312096));
#32115=CARTESIAN_POINT('',(-201.637568622845,-786.246777154128,-286.502310312096));
#32116=CARTESIAN_POINT('',(201.637568622845,-779.746879659443,-275.243920882049));
#32117=CARTESIAN_POINT('',(201.637568622845,-779.746879659443,-275.243920882049));
#32118=CARTESIAN_POINT('',(-201.637568622845,-779.746879659443,-275.243920882049));
#32119=CARTESIAN_POINT('Origin',(201.637568622845,-779.746879659443,-275.243920882049));
#32120=CARTESIAN_POINT('',(201.637568622845,-786.246777154128,-286.502310312096));
#32121=CARTESIAN_POINT('',(201.637568622845,-779.746879659443,-275.243920882049));
#32122=CARTESIAN_POINT('Origin',(6.46395147870936E-15,-314.113432458224,
-544.071864320163));
#32123=CARTESIAN_POINT('Origin',(6.46395147870936E-15,-320.613329952909,
-555.33025375021));
#32124=CARTESIAN_POINT('Origin',(376.048949668551,-533.224282489496,-403.252604600343));
#32125=CARTESIAN_POINT('',(387.309362287183,-538.85035247782,-400.004459876868));
#32126=CARTESIAN_POINT('',(328.342112775413,-627.367186960784,-348.900316227531));
#32127=CARTESIAN_POINT('',(387.309362287183,-538.85035247782,-400.004459876868));
#32128=CARTESIAN_POINT('',(317.081700156781,-621.74111697246,-352.148460951006));
#32129=CARTESIAN_POINT('',(317.081700156781,-621.74111697246,-352.148460951006));
#32130=CARTESIAN_POINT('',(376.048949668551,-533.224282489496,-403.252604600343));
#32131=CARTESIAN_POINT('',(376.048949668551,-533.224282489496,-403.252604600343));
#32132=CARTESIAN_POINT('',(376.048949668551,-533.224282489496,-403.252604600343));
#32133=CARTESIAN_POINT('Origin',(317.081700156781,-621.74111697246,-352.148460951006));
#32134=CARTESIAN_POINT('',(328.342112775413,-517.568918512102,-158.720137855359));
#32135=CARTESIAN_POINT('',(328.342112775413,-627.367186960784,-348.900316227531));
#32136=CARTESIAN_POINT('',(317.081700156781,-511.942848523778,-161.968282578834));
#32137=CARTESIAN_POINT('',(317.081700156781,-511.942848523778,-161.968282578834));
#32138=CARTESIAN_POINT('',(317.081700156781,-621.74111697246,-352.148460951006));
#32139=CARTESIAN_POINT('Origin',(376.048949668551,-423.426014040814,-213.072426228171));
#32140=CARTESIAN_POINT('',(387.309362287183,-429.052084029138,-209.824281504696));
#32141=CARTESIAN_POINT('',(387.309362287183,-429.052084029138,-209.824281504696));
#32142=CARTESIAN_POINT('',(376.048949668551,-423.426014040814,-213.072426228171));
#32143=CARTESIAN_POINT('',(376.048949668551,-423.426014040814,-213.072426228171));
#32144=CARTESIAN_POINT('',(376.048949668551,-423.426014040814,-213.072426228171));
#32145=CARTESIAN_POINT('Origin',(376.048949668551,-533.224282489496,-403.252604600343));
#32146=CARTESIAN_POINT('',(387.309362287183,-538.85035247782,-400.004459876868));
#32147=CARTESIAN_POINT('',(376.048949668551,-533.224282489496,-403.252604600343));
#32148=CARTESIAN_POINT('Origin',(394.754129766534,-197.232058670006,113.869587829266));
#32149=CARTESIAN_POINT('Origin',(406.014542385166,-202.85812865833,117.117732552741));
#32150=CARTESIAN_POINT('Origin',(376.051116910575,-418.422839624243,-204.414004948869));
#32151=CARTESIAN_POINT('',(387.311529529207,-424.048909612567,-201.165860225394));
#32152=CARTESIAN_POINT('',(328.344280017437,-512.565744095532,-150.061716576057));
#32153=CARTESIAN_POINT('',(387.311529529207,-424.048909612567,-201.165860225394));
#32154=CARTESIAN_POINT('',(317.083867398805,-506.939674107208,-153.309861299531));
#32155=CARTESIAN_POINT('',(317.083867398805,-506.939674107208,-153.309861299531));
#32156=CARTESIAN_POINT('',(376.051116910575,-418.422839624243,-204.414004948869));
#32157=CARTESIAN_POINT('',(376.051116910575,-418.422839624243,-204.414004948869));
#32158=CARTESIAN_POINT('',(376.051116910575,-418.422839624243,-204.414004948869));
#32159=CARTESIAN_POINT('Origin',(317.083867398805,-506.939674107208,-153.309861299531));
#32160=CARTESIAN_POINT('',(328.344280017437,-402.76747564685,40.1184617961154));
#32161=CARTESIAN_POINT('',(328.344280017437,-512.565744095532,-150.061716576057));
#32162=CARTESIAN_POINT('',(317.083867398805,-397.141405658526,36.8703170726406));
#32163=CARTESIAN_POINT('',(317.083867398805,-397.141405658526,36.8703170726406));
#32164=CARTESIAN_POINT('',(317.083867398805,-506.939674107208,-153.309861299531));
#32165=CARTESIAN_POINT('Origin',(376.051116910575,-308.624571175561,-14.2338265766968));
#32166=CARTESIAN_POINT('',(387.311529529207,-314.250641163885,-10.985681853222));
#32167=CARTESIAN_POINT('',(387.311529529207,-314.250641163885,-10.985681853222));
#32168=CARTESIAN_POINT('',(376.051116910575,-308.624571175561,-14.2338265766968));
#32169=CARTESIAN_POINT('',(376.051116910575,-308.624571175561,-14.2338265766968));
#32170=CARTESIAN_POINT('',(376.051116910575,-308.624571175561,-14.2338265766968));
#32171=CARTESIAN_POINT('Origin',(376.051116910575,-418.422839624243,-204.414004948869));
#32172=CARTESIAN_POINT('',(387.311529529207,-424.048909612567,-201.165860225394));
#32173=CARTESIAN_POINT('',(376.051116910575,-418.422839624243,-204.414004948869));
#32174=CARTESIAN_POINT('Origin',(394.756297008558,-82.4306158047535,312.70818748074));
#32175=CARTESIAN_POINT('Origin',(406.016709627189,-88.0566857930775,315.956332204215));
#32176=CARTESIAN_POINT('Origin',(312.084475633296,-629.241334735898,-347.815507460388));
#32177=CARTESIAN_POINT('',(323.344888251928,-634.867404724222,-344.567362736913));
#32178=CARTESIAN_POINT('',(264.377638740158,-723.384239207187,-293.463219087576));
#32179=CARTESIAN_POINT('',(323.344888251928,-634.867404724222,-344.567362736913));
#32180=CARTESIAN_POINT('',(253.117226121526,-717.758169218862,-296.711363811051));
#32181=CARTESIAN_POINT('',(253.117226121526,-717.758169218862,-296.711363811051));
#32182=CARTESIAN_POINT('',(312.084475633296,-629.241334735898,-347.815507460388));
#32183=CARTESIAN_POINT('',(312.084475633296,-629.241334735898,-347.815507460388));
#32184=CARTESIAN_POINT('',(312.084475633296,-629.241334735898,-347.815507460388));
#32185=CARTESIAN_POINT('Origin',(253.117226121526,-717.758169218862,-296.711363811051));
#32186=CARTESIAN_POINT('',(264.377638740158,-613.585970758505,-103.283040715404));
#32187=CARTESIAN_POINT('',(264.377638740158,-723.384239207187,-293.463219087576));
#32188=CARTESIAN_POINT('',(253.117226121526,-607.959900770181,-106.531185438879));
#32189=CARTESIAN_POINT('',(253.117226121526,-607.959900770181,-106.531185438879));
#32190=CARTESIAN_POINT('',(253.117226121526,-717.758169218862,-296.711363811051));
#32191=CARTESIAN_POINT('Origin',(312.084475633296,-519.443066287216,-157.635329088216));
#32192=CARTESIAN_POINT('',(323.344888251928,-525.06913627554,-154.387184364741));
#32193=CARTESIAN_POINT('',(323.344888251928,-525.06913627554,-154.387184364741));
#32194=CARTESIAN_POINT('',(312.084475633296,-519.443066287216,-157.635329088216));
#32195=CARTESIAN_POINT('',(312.084475633296,-519.443066287216,-157.635329088216));
#32196=CARTESIAN_POINT('',(312.084475633296,-519.443066287216,-157.635329088216));
#32197=CARTESIAN_POINT('Origin',(312.084475633296,-629.241334735898,-347.815507460388));
#32198=CARTESIAN_POINT('',(323.344888251928,-634.867404724222,-344.567362736913));
#32199=CARTESIAN_POINT('',(312.084475633296,-629.241334735898,-347.815507460388));
#32200=CARTESIAN_POINT('Origin',(330.789655731279,-293.249110916408,169.306684969221));
#32201=CARTESIAN_POINT('Origin',(342.050068349911,-298.875180904732,172.554829692696));
#32202=CARTESIAN_POINT('Origin',(312.08664287532,-514.439891870646,-148.976907808914));
#32203=CARTESIAN_POINT('',(323.347055493952,-520.06596185897,-145.728763085439));
#32204=CARTESIAN_POINT('',(264.379805982182,-608.582796341934,-94.6246194361014));
#32205=CARTESIAN_POINT('',(323.347055493952,-520.06596185897,-145.728763085439));
#32206=CARTESIAN_POINT('',(253.11939336355,-602.95672635361,-97.8727641595762));
#32207=CARTESIAN_POINT('',(253.11939336355,-602.95672635361,-97.8727641595762));
#32208=CARTESIAN_POINT('',(312.08664287532,-514.439891870646,-148.976907808914));
#32209=CARTESIAN_POINT('',(312.08664287532,-514.439891870646,-148.976907808914));
#32210=CARTESIAN_POINT('',(312.08664287532,-514.439891870646,-148.976907808914));
#32211=CARTESIAN_POINT('Origin',(253.11939336355,-602.95672635361,-97.8727641595762));
#32212=CARTESIAN_POINT('',(264.379805982182,-498.784527893252,95.5555589360706));
#32213=CARTESIAN_POINT('',(264.379805982182,-608.582796341934,-94.6246194361014));
#32214=CARTESIAN_POINT('',(253.11939336355,-493.158457904928,92.3074142125958));
#32215=CARTESIAN_POINT('',(253.11939336355,-493.158457904928,92.3074142125958));
#32216=CARTESIAN_POINT('',(253.11939336355,-602.95672635361,-97.8727641595762));
#32217=CARTESIAN_POINT('Origin',(312.08664287532,-404.641623421964,41.2032705632584));
#32218=CARTESIAN_POINT('',(323.347055493952,-410.267693410288,44.4514152867332));
#32219=CARTESIAN_POINT('',(323.347055493952,-410.267693410288,44.4514152867332));
#32220=CARTESIAN_POINT('',(312.08664287532,-404.641623421964,41.2032705632584));
#32221=CARTESIAN_POINT('',(312.08664287532,-404.641623421964,41.2032705632584));
#32222=CARTESIAN_POINT('',(312.08664287532,-404.641623421964,41.2032705632584));
#32223=CARTESIAN_POINT('Origin',(312.08664287532,-514.439891870646,-148.976907808914));
#32224=CARTESIAN_POINT('',(323.347055493952,-520.06596185897,-145.728763085439));
#32225=CARTESIAN_POINT('',(312.08664287532,-514.439891870646,-148.976907808914));
#32226=CARTESIAN_POINT('Origin',(330.791822973303,-178.447668051156,368.145284620695));
#32227=CARTESIAN_POINT('Origin',(342.052235591935,-184.07373803948,371.39342934417));
#32228=CARTESIAN_POINT('Origin',(-376.048949668551,-533.224282489496,-403.252604600343));
#32229=CARTESIAN_POINT('',(-387.309362287183,-538.85035247782,-400.004459876868));
#32230=CARTESIAN_POINT('',(-328.342112775413,-627.367186960784,-348.900316227531));
#32231=CARTESIAN_POINT('',(-387.309362287183,-538.85035247782,-400.004459876868));
#32232=CARTESIAN_POINT('',(-376.048949668551,-533.224282489496,-403.252604600343));
#32233=CARTESIAN_POINT('',(-376.048949668551,-533.224282489496,-403.252604600343));
#32234=CARTESIAN_POINT('',(-317.081700156781,-621.74111697246,-352.148460951006));
#32235=CARTESIAN_POINT('',(-376.048949668551,-533.224282489496,-403.252604600343));
#32236=CARTESIAN_POINT('',(-317.081700156781,-621.74111697246,-352.148460951006));
#32237=CARTESIAN_POINT('Origin',(-317.081700156781,-621.74111697246,-352.148460951006));
#32238=CARTESIAN_POINT('',(-328.342112775413,-517.568918512102,-158.720137855359));
#32239=CARTESIAN_POINT('',(-328.342112775413,-627.367186960784,-348.900316227531));
#32240=CARTESIAN_POINT('',(-317.081700156781,-511.942848523778,-161.968282578834));
#32241=CARTESIAN_POINT('',(-317.081700156781,-621.74111697246,-352.148460951006));
#32242=CARTESIAN_POINT('',(-317.081700156781,-511.942848523778,-161.968282578834));
#32243=CARTESIAN_POINT('Origin',(-376.048949668551,-423.426014040814,-213.072426228171));
#32244=CARTESIAN_POINT('',(-387.309362287183,-429.052084029138,-209.824281504696));
#32245=CARTESIAN_POINT('',(-387.309362287183,-429.052084029138,-209.824281504696));
#32246=CARTESIAN_POINT('',(-376.048949668551,-423.426014040814,-213.072426228171));
#32247=CARTESIAN_POINT('',(-376.048949668551,-423.426014040814,-213.072426228171));
#32248=CARTESIAN_POINT('',(-376.048949668551,-423.426014040814,-213.072426228171));
#32249=CARTESIAN_POINT('Origin',(-376.048949668551,-533.224282489496,-403.252604600343));
#32250=CARTESIAN_POINT('',(-387.309362287183,-538.85035247782,-400.004459876868));
#32251=CARTESIAN_POINT('',(-376.048949668551,-533.224282489496,-403.252604600343));
#32252=CARTESIAN_POINT('Origin',(-394.754129766534,-197.232058670006,113.869587829266));
#32253=CARTESIAN_POINT('Origin',(-406.014542385166,-202.85812865833,117.117732552741));
#32254=CARTESIAN_POINT('Origin',(-376.051116910575,-418.422839624243,-204.414004948869));
#32255=CARTESIAN_POINT('',(-387.311529529207,-424.048909612567,-201.165860225394));
#32256=CARTESIAN_POINT('',(-328.344280017437,-512.565744095532,-150.061716576057));
#32257=CARTESIAN_POINT('',(-387.311529529207,-424.048909612567,-201.165860225394));
#32258=CARTESIAN_POINT('',(-376.051116910575,-418.422839624243,-204.414004948869));
#32259=CARTESIAN_POINT('',(-376.051116910575,-418.422839624243,-204.414004948869));
#32260=CARTESIAN_POINT('',(-317.083867398805,-506.939674107208,-153.309861299531));
#32261=CARTESIAN_POINT('',(-376.051116910575,-418.422839624243,-204.414004948869));
#32262=CARTESIAN_POINT('',(-317.083867398805,-506.939674107208,-153.309861299531));
#32263=CARTESIAN_POINT('Origin',(-317.083867398805,-506.939674107208,-153.309861299531));
#32264=CARTESIAN_POINT('',(-328.344280017437,-402.76747564685,40.1184617961154));
#32265=CARTESIAN_POINT('',(-328.344280017437,-512.565744095532,-150.061716576057));
#32266=CARTESIAN_POINT('',(-317.083867398805,-397.141405658526,36.8703170726406));
#32267=CARTESIAN_POINT('',(-317.083867398805,-506.939674107208,-153.309861299531));
#32268=CARTESIAN_POINT('',(-317.083867398805,-397.141405658526,36.8703170726406));
#32269=CARTESIAN_POINT('Origin',(-376.051116910575,-308.624571175561,-14.2338265766968));
#32270=CARTESIAN_POINT('',(-387.311529529207,-314.250641163885,-10.985681853222));
#32271=CARTESIAN_POINT('',(-387.311529529207,-314.250641163885,-10.985681853222));
#32272=CARTESIAN_POINT('',(-376.051116910575,-308.624571175561,-14.2338265766968));
#32273=CARTESIAN_POINT('',(-376.051116910575,-308.624571175561,-14.2338265766968));
#32274=CARTESIAN_POINT('',(-376.051116910575,-308.624571175561,-14.2338265766968));
#32275=CARTESIAN_POINT('Origin',(-376.051116910575,-418.422839624243,-204.414004948869));
#32276=CARTESIAN_POINT('',(-387.311529529207,-424.048909612567,-201.165860225394));
#32277=CARTESIAN_POINT('',(-376.051116910575,-418.422839624243,-204.414004948869));
#32278=CARTESIAN_POINT('Origin',(-394.756297008558,-82.4306158047535,312.70818748074));
#32279=CARTESIAN_POINT('Origin',(-406.016709627189,-88.0566857930775,315.956332204215));
#32280=CARTESIAN_POINT('Origin',(-312.084475633296,-629.241334735898,-347.815507460388));
#32281=CARTESIAN_POINT('',(-323.344888251928,-634.867404724222,-344.567362736913));
#32282=CARTESIAN_POINT('',(-264.377638740158,-723.384239207187,-293.463219087576));
#32283=CARTESIAN_POINT('',(-323.344888251928,-634.867404724222,-344.567362736913));
#32284=CARTESIAN_POINT('',(-312.084475633296,-629.241334735898,-347.815507460388));
#32285=CARTESIAN_POINT('',(-312.084475633296,-629.241334735898,-347.815507460388));
#32286=CARTESIAN_POINT('',(-253.117226121526,-717.758169218862,-296.711363811051));
#32287=CARTESIAN_POINT('',(-312.084475633296,-629.241334735898,-347.815507460388));
#32288=CARTESIAN_POINT('',(-253.117226121526,-717.758169218862,-296.711363811051));
#32289=CARTESIAN_POINT('Origin',(-253.117226121526,-717.758169218862,-296.711363811051));
#32290=CARTESIAN_POINT('',(-264.377638740158,-613.585970758505,-103.283040715404));
#32291=CARTESIAN_POINT('',(-264.377638740158,-723.384239207187,-293.463219087576));
#32292=CARTESIAN_POINT('',(-253.117226121526,-607.959900770181,-106.531185438879));
#32293=CARTESIAN_POINT('',(-253.117226121526,-717.758169218862,-296.711363811051));
#32294=CARTESIAN_POINT('',(-253.117226121526,-607.959900770181,-106.531185438879));
#32295=CARTESIAN_POINT('Origin',(-312.084475633296,-519.443066287216,-157.635329088216));
#32296=CARTESIAN_POINT('',(-323.344888251928,-525.06913627554,-154.387184364741));
#32297=CARTESIAN_POINT('',(-323.344888251928,-525.06913627554,-154.387184364741));
#32298=CARTESIAN_POINT('',(-312.084475633296,-519.443066287216,-157.635329088216));
#32299=CARTESIAN_POINT('',(-312.084475633296,-519.443066287216,-157.635329088216));
#32300=CARTESIAN_POINT('',(-312.084475633296,-519.443066287216,-157.635329088216));
#32301=CARTESIAN_POINT('Origin',(-312.084475633296,-629.241334735898,-347.815507460388));
#32302=CARTESIAN_POINT('',(-323.344888251928,-634.867404724222,-344.567362736913));
#32303=CARTESIAN_POINT('',(-312.084475633296,-629.241334735898,-347.815507460388));
#32304=CARTESIAN_POINT('Origin',(-330.789655731279,-293.249110916408,169.306684969221));
#32305=CARTESIAN_POINT('Origin',(-342.050068349911,-298.875180904732,172.554829692696));
#32306=CARTESIAN_POINT('Origin',(-312.08664287532,-514.439891870646,-148.976907808914));
#32307=CARTESIAN_POINT('',(-323.347055493952,-520.06596185897,-145.728763085439));
#32308=CARTESIAN_POINT('',(-264.379805982182,-608.582796341934,-94.6246194361014));
#32309=CARTESIAN_POINT('',(-323.347055493952,-520.06596185897,-145.728763085439));
#32310=CARTESIAN_POINT('',(-312.08664287532,-514.439891870646,-148.976907808914));
#32311=CARTESIAN_POINT('',(-312.08664287532,-514.439891870646,-148.976907808914));
#32312=CARTESIAN_POINT('',(-253.11939336355,-602.95672635361,-97.8727641595762));
#32313=CARTESIAN_POINT('',(-312.08664287532,-514.439891870646,-148.976907808914));
#32314=CARTESIAN_POINT('',(-253.11939336355,-602.95672635361,-97.8727641595762));
#32315=CARTESIAN_POINT('Origin',(-253.11939336355,-602.95672635361,-97.8727641595762));
#32316=CARTESIAN_POINT('',(-264.379805982182,-498.784527893252,95.5555589360706));
#32317=CARTESIAN_POINT('',(-264.379805982182,-608.582796341934,-94.6246194361014));
#32318=CARTESIAN_POINT('',(-253.11939336355,-493.158457904928,92.3074142125958));
#32319=CARTESIAN_POINT('',(-253.11939336355,-602.95672635361,-97.8727641595762));
#32320=CARTESIAN_POINT('',(-253.11939336355,-493.158457904928,92.3074142125958));
#32321=CARTESIAN_POINT('Origin',(-312.08664287532,-404.641623421964,41.2032705632584));
#32322=CARTESIAN_POINT('',(-323.347055493952,-410.267693410288,44.4514152867332));
#32323=CARTESIAN_POINT('',(-323.347055493952,-410.267693410288,44.4514152867332));
#32324=CARTESIAN_POINT('',(-312.08664287532,-404.641623421964,41.2032705632584));
#32325=CARTESIAN_POINT('',(-312.08664287532,-404.641623421964,41.2032705632584));
#32326=CARTESIAN_POINT('',(-312.08664287532,-404.641623421964,41.2032705632584));
#32327=CARTESIAN_POINT('Origin',(-312.08664287532,-514.439891870646,-148.976907808914));
#32328=CARTESIAN_POINT('',(-323.347055493952,-520.06596185897,-145.728763085439));
#32329=CARTESIAN_POINT('',(-312.08664287532,-514.439891870646,-148.976907808914));
#32330=CARTESIAN_POINT('Origin',(-330.791822973303,-178.447668051156,368.145284620695));
#32331=CARTESIAN_POINT('Origin',(-342.052235591935,-184.07373803948,371.39342934417));
#32332=CARTESIAN_POINT('Origin',(368.833006272647,-291.775764149142,-9.65537551417994));
#32333=CARTESIAN_POINT('',(368.833128982344,-285.27568245381,1.60290756713166));
#32334=CARTESIAN_POINT('',(-368.828409446333,-285.27220098925,1.60893765350545));
#32335=CARTESIAN_POINT('',(368.833128982344,-285.27568245381,1.60290756713166));
#32336=CARTESIAN_POINT('',(368.833006272647,-291.775764149142,-9.65537551417994));
#32337=CARTESIAN_POINT('',(368.833006272647,-291.775764149142,-9.65537551417994));
#32338=CARTESIAN_POINT('',(-368.828532156029,-291.772282684582,-9.64934542780627));
#32339=CARTESIAN_POINT('',(368.833006272647,-291.775764149142,-9.65537551417994));
#32340=CARTESIAN_POINT('',(-368.828532156029,-291.772282684582,-9.64934542780627));
#32341=CARTESIAN_POINT('Origin',(-368.828532156029,-291.772282684582,-9.64934542780627));
#32342=CARTESIAN_POINT('',(-201.635208823479,-536.24744098009,146.510165970204));
#32343=CARTESIAN_POINT('',(-368.828409446333,-285.27220098925,1.60893765350545));
#32344=CARTESIAN_POINT('',(-201.635331533176,-542.747522675422,135.251882888892));
#32345=CARTESIAN_POINT('',(-368.828532156029,-291.772282684582,-9.64934542780627));
#32346=CARTESIAN_POINT('',(-201.635331533176,-542.747522675422,135.251882888892));
#32347=CARTESIAN_POINT('Origin',(-201.635331533176,-542.747522675422,135.251882888892));
#32348=CARTESIAN_POINT('',(201.639928404246,-536.249344275877,146.506869358163));
#32349=CARTESIAN_POINT('',(-201.635208823479,-536.24744098009,146.510165970204));
#32350=CARTESIAN_POINT('',(201.63980569455,-542.74942597121,135.248586276851));
#32351=CARTESIAN_POINT('',(-201.635331533176,-542.747522675422,135.251882888892));
#32352=CARTESIAN_POINT('',(201.63980569455,-542.74942597121,135.248586276851));
#32353=CARTESIAN_POINT('Origin',(201.63980569455,-542.74942597121,135.248586276851));
#32354=CARTESIAN_POINT('',(201.639928404246,-536.249344275877,146.506869358163));
#32355=CARTESIAN_POINT('',(201.63980569455,-542.74942597121,135.248586276851));
#32356=CARTESIAN_POINT('Origin',(0.0022370391692238,-77.1194255571307,-133.585327184455));
#32357=CARTESIAN_POINT('Origin',(0.00235974886567285,-70.6193438617984,
-122.327044103143));
#32358=CARTESIAN_POINT('Origin',(374.6,62.3000000000001,-13.));
#32359=CARTESIAN_POINT('',(374.6,62.3000000000001,0.));
#32360=CARTESIAN_POINT('',(374.6,-267.5,0.));
#32361=CARTESIAN_POINT('',(374.6,62.3000000000001,0.));
#32362=CARTESIAN_POINT('',(374.6,-267.5,-13.));
#32363=CARTESIAN_POINT('',(374.6,-267.5,-13.));
#32364=CARTESIAN_POINT('',(374.6,62.3000000000001,-13.));
#32365=CARTESIAN_POINT('',(374.6,62.3000000000001,-13.));
#32366=CARTESIAN_POINT('',(374.6,62.3000000000001,-13.));
#32367=CARTESIAN_POINT('Origin',(374.6,-267.5,-13.));
#32368=CARTESIAN_POINT('',(194.8,-267.5,0.));
#32369=CARTESIAN_POINT('',(374.6,-267.5,0.));
#32370=CARTESIAN_POINT('',(194.8,-267.5,-13.));
#32371=CARTESIAN_POINT('',(194.8,-267.5,-13.));
#32372=CARTESIAN_POINT('',(374.6,-267.5,-13.));
#32373=CARTESIAN_POINT('Origin',(194.8,62.3000000000001,-13.));
#32374=CARTESIAN_POINT('',(194.8,62.3000000000001,0.));
#32375=CARTESIAN_POINT('',(194.8,62.3000000000001,0.));
#32376=CARTESIAN_POINT('',(194.8,62.3000000000001,-13.));
#32377=CARTESIAN_POINT('',(194.8,62.3000000000001,-13.));
#32378=CARTESIAN_POINT('',(194.8,62.3000000000001,-13.));
#32379=CARTESIAN_POINT('Origin',(374.6,62.3000000000001,-13.));
#32380=CARTESIAN_POINT('',(374.6,62.3000000000001,0.));
#32381=CARTESIAN_POINT('',(374.6,62.3000000000001,-13.));
#32382=CARTESIAN_POINT('Origin',(0.,0.,-13.));
#32383=CARTESIAN_POINT('Origin',(0.,0.,0.));
#32384=CARTESIAN_POINT('Origin',(184.8,62.3000000000001,-13.));
#32385=CARTESIAN_POINT('',(184.8,62.3000000000001,0.));
#32386=CARTESIAN_POINT('',(184.8,-267.5,0.));
#32387=CARTESIAN_POINT('',(184.8,62.3000000000001,0.));
#32388=CARTESIAN_POINT('',(184.8,-267.5,-13.));
#32389=CARTESIAN_POINT('',(184.8,-267.5,-13.));
#32390=CARTESIAN_POINT('',(184.8,62.3000000000001,-13.));
#32391=CARTESIAN_POINT('',(184.8,62.3000000000001,-13.));
#32392=CARTESIAN_POINT('',(184.8,62.3000000000001,-13.));
#32393=CARTESIAN_POINT('Origin',(184.8,-267.5,-13.));
#32394=CARTESIAN_POINT('',(4.99999999999998,-267.5,0.));
#32395=CARTESIAN_POINT('',(184.8,-267.5,0.));
#32396=CARTESIAN_POINT('',(4.99999999999998,-267.5,-13.));
#32397=CARTESIAN_POINT('',(4.99999999999998,-267.5,-13.));
#32398=CARTESIAN_POINT('',(184.8,-267.5,-13.));
#32399=CARTESIAN_POINT('Origin',(5.00000000000003,62.3000000000001,-13.));
#32400=CARTESIAN_POINT('',(5.00000000000003,62.3000000000001,0.));
#32401=CARTESIAN_POINT('',(5.00000000000003,62.3000000000001,0.));
#32402=CARTESIAN_POINT('',(5.00000000000003,62.3000000000001,-13.));
#32403=CARTESIAN_POINT('',(5.00000000000003,62.3000000000001,-13.));
#32404=CARTESIAN_POINT('',(5.00000000000003,62.3000000000001,-13.));
#32405=CARTESIAN_POINT('Origin',(184.8,62.3000000000001,-13.));
#32406=CARTESIAN_POINT('',(184.8,62.3000000000001,0.));
#32407=CARTESIAN_POINT('',(184.8,62.3000000000001,-13.));
#32408=CARTESIAN_POINT('Origin',(0.,0.,-13.));
#32409=CARTESIAN_POINT('Origin',(0.,0.,0.));
#32410=CARTESIAN_POINT('Origin',(374.6,72.3000000000001,-13.));
#32411=CARTESIAN_POINT('',(374.6,252.1,0.));
#32412=CARTESIAN_POINT('',(374.6,72.3000000000001,0.));
#32413=CARTESIAN_POINT('',(374.6,72.3000000000001,0.));
#32414=CARTESIAN_POINT('',(374.6,72.3000000000001,-13.));
#32415=CARTESIAN_POINT('',(374.6,72.3000000000001,-13.));
#32416=CARTESIAN_POINT('',(374.6,252.1,-13.));
#32417=CARTESIAN_POINT('',(374.6,72.3000000000001,-13.));
#32418=CARTESIAN_POINT('',(374.6,252.1,-13.));
#32419=CARTESIAN_POINT('Origin',(374.6,72.3000000000001,-13.));
#32420=CARTESIAN_POINT('',(5.,72.3000000000001,0.));
#32421=CARTESIAN_POINT('',(374.6,72.3000000000001,0.));
#32422=CARTESIAN_POINT('',(5.,72.3000000000001,-13.));
#32423=CARTESIAN_POINT('',(5.,72.3000000000001,-13.));
#32424=CARTESIAN_POINT('',(374.6,72.3000000000001,-13.));
#32425=CARTESIAN_POINT('Origin',(5.,72.3000000000001,-13.));
#32426=CARTESIAN_POINT('',(5.,252.1,0.));
#32427=CARTESIAN_POINT('',(5.,72.3000000000001,0.));
#32428=CARTESIAN_POINT('',(5.,252.1,-13.));
#32429=CARTESIAN_POINT('',(5.,252.1,-13.));
#32430=CARTESIAN_POINT('',(5.,72.3000000000001,-13.));
#32431=CARTESIAN_POINT('Origin',(374.6,252.1,-13.));
#32432=CARTESIAN_POINT('',(374.6,252.1,0.));
#32433=CARTESIAN_POINT('',(374.6,252.1,-13.));
#32434=CARTESIAN_POINT('Origin',(0.,0.,-13.));
#32435=CARTESIAN_POINT('Origin',(0.,0.,0.));
#32436=CARTESIAN_POINT('Origin',(-5.,72.3000000000001,-13.));
#32437=CARTESIAN_POINT('',(-5.,252.1,0.));
#32438=CARTESIAN_POINT('',(-5.,72.3000000000001,0.));
#32439=CARTESIAN_POINT('',(-5.,72.3000000000001,0.));
#32440=CARTESIAN_POINT('',(-5.,72.3000000000001,-13.));
#32441=CARTESIAN_POINT('',(-5.,72.3000000000001,-13.));
#32442=CARTESIAN_POINT('',(-5.,252.1,-13.));
#32443=CARTESIAN_POINT('',(-5.,72.3000000000001,-13.));
#32444=CARTESIAN_POINT('',(-5.,252.1,-13.));
#32445=CARTESIAN_POINT('Origin',(-5.,72.3000000000001,-13.));
#32446=CARTESIAN_POINT('',(-374.6,72.3000000000001,0.));
#32447=CARTESIAN_POINT('',(-5.,72.3000000000001,0.));
#32448=CARTESIAN_POINT('',(-374.6,72.3000000000001,-13.));
#32449=CARTESIAN_POINT('',(-374.6,72.3000000000001,-13.));
#32450=CARTESIAN_POINT('',(-5.,72.3000000000001,-13.));
#32451=CARTESIAN_POINT('Origin',(-374.6,72.3000000000001,-13.));
#32452=CARTESIAN_POINT('',(-374.6,252.1,0.));
#32453=CARTESIAN_POINT('',(-374.6,72.3000000000001,0.));
#32454=CARTESIAN_POINT('',(-374.6,252.1,-13.));
#32455=CARTESIAN_POINT('',(-374.6,252.1,-13.));
#32456=CARTESIAN_POINT('',(-374.6,72.3000000000001,-13.));
#32457=CARTESIAN_POINT('Origin',(-5.,252.1,-13.));
#32458=CARTESIAN_POINT('',(-5.,252.1,0.));
#32459=CARTESIAN_POINT('',(-5.,252.1,-13.));
#32460=CARTESIAN_POINT('Origin',(0.,0.,-13.));
#32461=CARTESIAN_POINT('Origin',(0.,0.,0.));
#32462=CARTESIAN_POINT('Origin',(-4.99999999999989,62.3000000000001,-13.));
#32463=CARTESIAN_POINT('',(-4.99999999999989,62.3000000000001,0.));
#32464=CARTESIAN_POINT('',(-5.00000000000002,-267.5,0.));
#32465=CARTESIAN_POINT('',(-4.99999999999989,62.3000000000001,0.));
#32466=CARTESIAN_POINT('',(-5.00000000000002,-267.5,-13.));
#32467=CARTESIAN_POINT('',(-5.00000000000002,-267.5,-13.));
#32468=CARTESIAN_POINT('',(-4.99999999999989,62.3000000000001,-13.));
#32469=CARTESIAN_POINT('',(-4.99999999999989,62.3000000000001,-13.));
#32470=CARTESIAN_POINT('',(-4.99999999999989,62.3000000000001,-13.));
#32471=CARTESIAN_POINT('Origin',(-5.00000000000002,-267.5,-13.));
#32472=CARTESIAN_POINT('',(-184.8,-267.5,0.));
#32473=CARTESIAN_POINT('',(-5.00000000000002,-267.5,0.));
#32474=CARTESIAN_POINT('',(-184.8,-267.5,-13.));
#32475=CARTESIAN_POINT('',(-184.8,-267.5,-13.));
#32476=CARTESIAN_POINT('',(-5.00000000000002,-267.5,-13.));
#32477=CARTESIAN_POINT('Origin',(-184.8,62.3000000000001,-13.));
#32478=CARTESIAN_POINT('',(-184.8,62.3000000000001,0.));
#32479=CARTESIAN_POINT('',(-184.8,62.3000000000001,0.));
#32480=CARTESIAN_POINT('',(-184.8,62.3000000000001,-13.));
#32481=CARTESIAN_POINT('',(-184.8,62.3000000000001,-13.));
#32482=CARTESIAN_POINT('',(-184.8,62.3000000000001,-13.));
#32483=CARTESIAN_POINT('Origin',(-4.99999999999989,62.3000000000001,-13.));
#32484=CARTESIAN_POINT('',(-4.99999999999989,62.3000000000001,0.));
#32485=CARTESIAN_POINT('',(-4.99999999999989,62.3000000000001,-13.));
#32486=CARTESIAN_POINT('Origin',(0.,0.,-13.));
#32487=CARTESIAN_POINT('Origin',(0.,0.,0.));
#32488=CARTESIAN_POINT('Origin',(-194.8,62.3000000000001,-13.));
#32489=CARTESIAN_POINT('',(-194.8,62.3000000000001,0.));
#32490=CARTESIAN_POINT('',(-194.8,-267.5,0.));
#32491=CARTESIAN_POINT('',(-194.8,62.3000000000001,0.));
#32492=CARTESIAN_POINT('',(-194.8,-267.5,-13.));
#32493=CARTESIAN_POINT('',(-194.8,-267.5,-13.));
#32494=CARTESIAN_POINT('',(-194.8,62.3000000000001,-13.));
#32495=CARTESIAN_POINT('',(-194.8,62.3000000000001,-13.));
#32496=CARTESIAN_POINT('',(-194.8,62.3000000000001,-13.));
#32497=CARTESIAN_POINT('Origin',(-194.8,-267.5,-13.));
#32498=CARTESIAN_POINT('',(-374.6,-267.5,0.));
#32499=CARTESIAN_POINT('',(-194.8,-267.5,0.));
#32500=CARTESIAN_POINT('',(-374.6,-267.5,-13.));
#32501=CARTESIAN_POINT('',(-374.6,-267.5,-13.));
#32502=CARTESIAN_POINT('',(-194.8,-267.5,-13.));
#32503=CARTESIAN_POINT('Origin',(-374.6,62.3000000000001,-13.));
#32504=CARTESIAN_POINT('',(-374.6,62.3000000000001,0.));
#32505=CARTESIAN_POINT('',(-374.6,62.3000000000001,0.));
#32506=CARTESIAN_POINT('',(-374.6,62.3000000000001,-13.));
#32507=CARTESIAN_POINT('',(-374.6,62.3000000000001,-13.));
#32508=CARTESIAN_POINT('',(-374.6,62.3000000000001,-13.));
#32509=CARTESIAN_POINT('Origin',(-194.8,62.3000000000001,-13.));
#32510=CARTESIAN_POINT('',(-194.8,62.3000000000001,0.));
#32511=CARTESIAN_POINT('',(-194.8,62.3000000000001,-13.));
#32512=CARTESIAN_POINT('Origin',(0.,0.,-13.));
#32513=CARTESIAN_POINT('Origin',(0.,0.,0.));
#32882=UNCERTAINTY_MEASURE_WITH_UNIT(LENGTH_MEASURE(0.01),#32904,
'DISTANCE_ACCURACY_VALUE',
'Maximum model space distance between geometric entities at asserted c
onnectivities');
#32886=UNCERTAINTY_MEASURE_WITH_UNIT(LENGTH_MEASURE(0.01),#32904,
'DISTANCE_ACCURACY_VALUE',
'Maximum model space distance between geometric entities at asserted c
onnectivities');
#32899=(
GEOMETRIC_REPRESENTATION_CONTEXT(3)
GLOBAL_UNCERTAINTY_ASSIGNED_CONTEXT((#32882))
GLOBAL_UNIT_ASSIGNED_CONTEXT((#32904,#32906,#32907))
REPRESENTATION_CONTEXT('','3D')
);
#32903=(
GEOMETRIC_REPRESENTATION_CONTEXT(3)
GLOBAL_UNCERTAINTY_ASSIGNED_CONTEXT((#32886))
GLOBAL_UNIT_ASSIGNED_CONTEXT((#32904,#32906,#32907))
REPRESENTATION_CONTEXT('','3D')
);
#32904=(
LENGTH_UNIT()
NAMED_UNIT(*)
SI_UNIT(.MILLI.,.METRE.)
);
#32906=(
NAMED_UNIT(*)
PLANE_ANGLE_UNIT()
SI_UNIT($,.RADIAN.)
);
#32907=(
NAMED_UNIT(*)
SI_UNIT($,.STERADIAN.)
SOLID_ANGLE_UNIT()
);
#32920=SHAPE_DEFINITION_REPRESENTATION(#32956,#33024);
#32956=PRODUCT_DEFINITION_SHAPE('',$,#33041);
#33024=SHAPE_REPRESENTATION('',(#16548),#32899);
#33028=PRODUCT_DEFINITION_CONTEXT('part definition',#33078,'design');
#33041=PRODUCT_DEFINITION('Chute Body','Chute Body',#33057,#33028);
#33057=PRODUCT_DEFINITION_FORMATION('',$,#33092);
#33078=APPLICATION_CONTEXT(
'Core Data for Automotive Mechanical Design Process');
#33079=PRODUCT_CONTEXT('part definition',#33078,'mechanical');
#33092=PRODUCT('Chute Body','Chute Body',$,(#33079));
#33101=PRESENTATION_STYLE_ASSIGNMENT((#33107));
#33107=SURFACE_STYLE_USAGE(.BOTH.,#33113);
#33113=SURFACE_SIDE_STYLE('',(#33119));
#33119=SURFACE_STYLE_FILL_AREA(#33125);
#33125=FILL_AREA_STYLE('Opaque(20,51,87)',(#33131));
#33131=FILL_AREA_STYLE_COLOUR('Opaque(20,51,87)',#33137);
#33137=COLOUR_RGB('Opaque(20,51,87)',0.0784313725490196,0.2,0.341176470588235);
ENDSEC;
END-ISO-10303-21;
